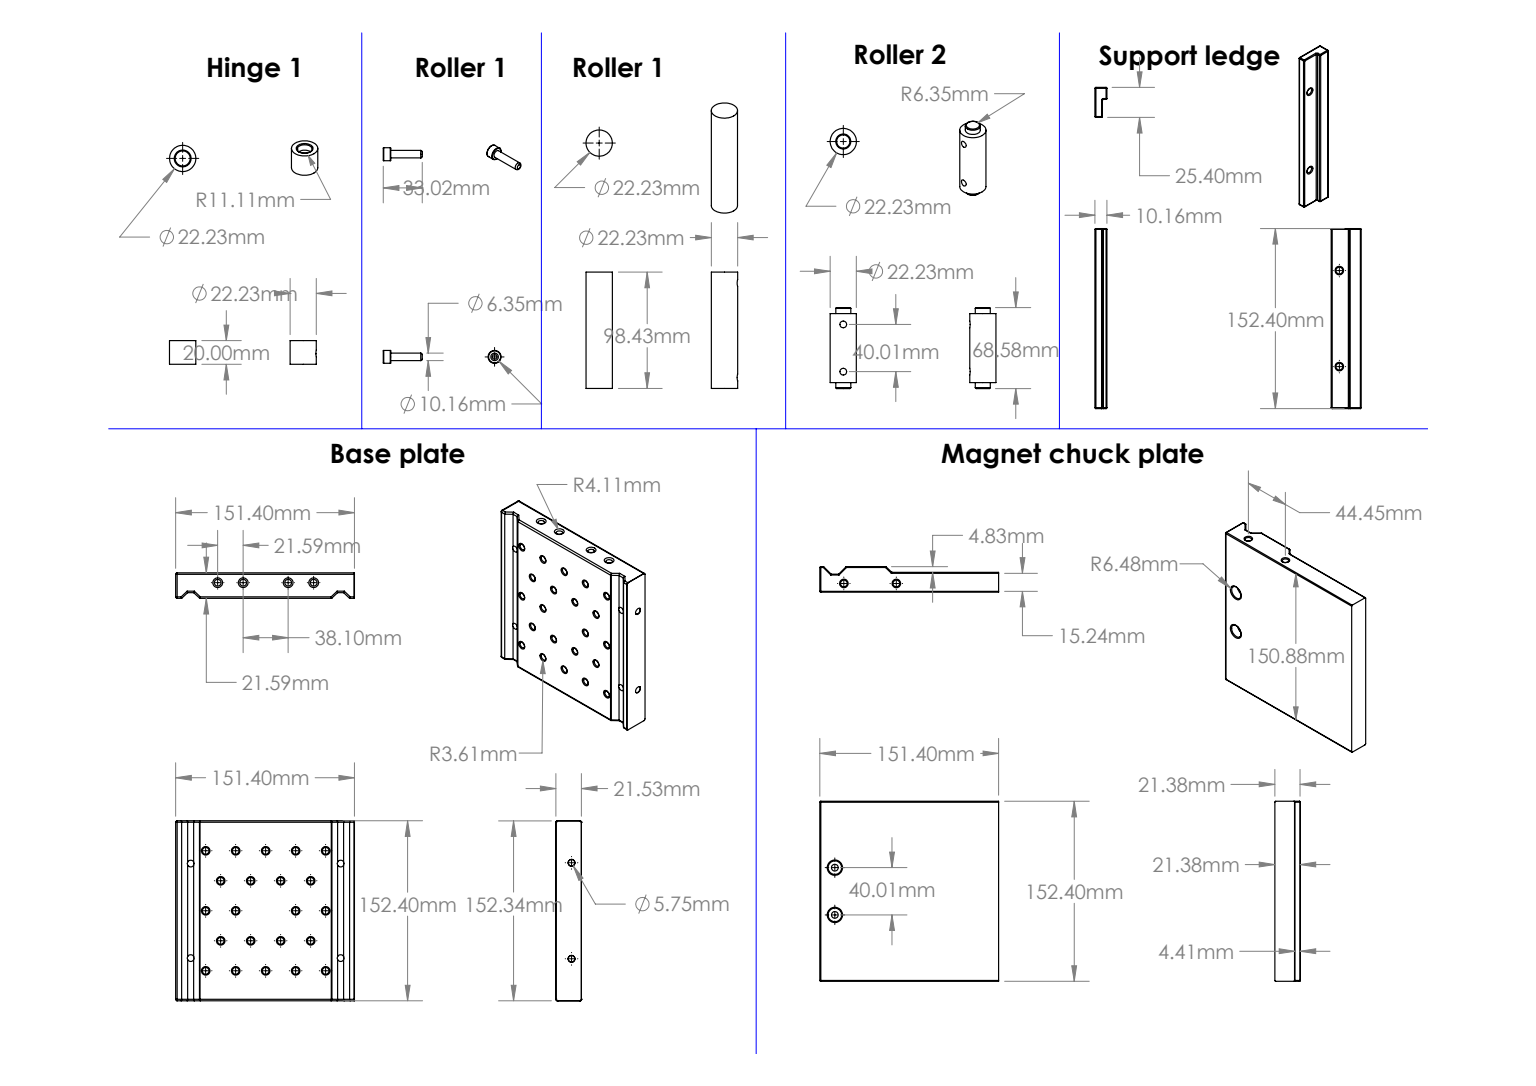
ISO-10303-21;
HEADER;
FILE_DESCRIPTION (('STEP AP214'),
    '1' );
FILE_NAME ('Base Plate.step',
    '2026-10-26T17:37:43',
    ( '' ),
    ( '' ),
    'SwSTEP 2.0',
    'SolidWorks 2024',
    '' );
FILE_SCHEMA (( 'AUTOMOTIVE_DESIGN' ));
ENDSEC;

DATA;
#2=CARTESIAN_POINT ( 'NONE',  ( 137.0307011298872908, -3580.478779010893959, 2249.731360258177119 ) ) ;
#4=DIRECTION ( 'NONE',  ( 0.000000000000000000, 1.000000000000000000, 0.000000000000000000 ) ) ;
#7=CARTESIAN_POINT ( 'NONE',  ( 116.8400000000000034, -3543.299999999999727, 2247.392000000000280 ) ) ;
#9=DIRECTION ( 'NONE',  ( -1.000000000000000000, 0.000000000000000000, 0.000000000000000000 ) ) ;
#13=EDGE_LOOP ( 'NONE', ( #4801, #14751 ) ) ;
#15=CARTESIAN_POINT ( 'NONE',  ( 15.55036781974841453, -3695.600514565457615, 2254.996746371283280 ) ) ;
#18=CARTESIAN_POINT ( 'NONE',  ( 50.79999999999999716, -3619.500000000000000, 2259.837999999999738 ) ) ;
#20=DIRECTION ( 'NONE',  ( 9.756599977372053330E-14, 0.000000000000000000, -1.000000000000000000 ) ) ;
#22=FACE_OUTER_BOUND ( 'NONE', #22533, .T. ) ;
#29=CARTESIAN_POINT ( 'NONE',  ( 17.55427699106284933, -3576.478798487876247, 2245.835327951717773 ) ) ;
#31=DIRECTION ( 'NONE',  ( 0.000000000000000000, 0.000000000000000000, -1.000000000000000000 ) ) ;
#34=CARTESIAN_POINT ( 'NONE',  ( 9.652920519510999497, -3695.699999999999818, 2254.503999999999905 ) ) ;
#37=CARTESIAN_POINT ( 'NONE',  ( 137.2900278743959745, -3657.993505329751770, 2249.258937114173477 ) ) ;
#41=ORIENTED_EDGE ( 'NONE', *, *, #19227, .F. ) ;
#45=EDGE_LOOP ( 'NONE', ( #8949, #290, #14111, #10584 ) ) ;
#48=ORIENTED_EDGE ( 'NONE', *, *, #14973, .T. ) ;
#49=ORIENTED_EDGE ( 'NONE', *, *, #4852, .F. ) ;
#50=DIRECTION ( 'NONE',  ( 0.000000000000000000, 0.000000000000000000, -1.000000000000000000 ) ) ;
#51=ADVANCED_FACE ( 'NONE', ( #16778 ), #19588, .T. ) ;
#54=CYLINDRICAL_SURFACE ( 'NONE', #7821, 5.714999999999998082 ) ;
#58=CARTESIAN_POINT ( 'NONE',  ( 12.69999999999999929, -3579.494999999999891, 2246.630000000000109 ) ) ;
#59=CYLINDRICAL_SURFACE ( 'NONE', #10460, 2.844800000000091700 ) ;
#61=CARTESIAN_POINT ( 'NONE',  ( 116.8400000000000034, -3694.430000000000291, 2247.392000000000280 ) ) ;
#63=EDGE_CURVE ( 'NONE', #17851, #18027, #1534, .T. ) ;
#65=ORIENTED_EDGE ( 'NONE', *, *, #14589, .T. ) ;
#67=DIRECTION ( 'NONE',  ( 0.000000000000000000, 0.000000000000000000, 1.000000000000000000 ) ) ;
#68=ORIENTED_EDGE ( 'NONE', *, *, #2483, .T. ) ;
#71=CARTESIAN_POINT ( 'NONE',  ( 25.39999999999999858, -3660.140000000000327, 2247.392000000000280 ) ) ;
#72=CARTESIAN_POINT ( 'NONE',  ( 41.70680000000000121, -3644.899999999999636, 2239.009999999999764 ) ) ;
#73=CARTESIAN_POINT ( 'NONE',  ( 151.1299999999999955, -3694.430000000000291, 2259.329999999999927 ) ) ;
#75=CARTESIAN_POINT ( 'NONE',  ( 18.25500259602790720, -3658.162202898845862, 2245.347138497373180 ) ) ;
#76=EDGE_CURVE ( 'NONE', #7743, #14640, #1242, .T. ) ;
#78=FACE_OUTER_BOUND ( 'NONE', #21782, .T. ) ;
#79=EDGE_CURVE ( 'NONE', #18611, #6224, #7995, .T. ) ;
#84=CARTESIAN_POINT ( 'NONE',  ( 137.1117535491106594, -3694.976217804482530, 2255.653245237783267 ) ) ;
#85=ORIENTED_EDGE ( 'NONE', *, *, #8808, .F. ) ;
#87=DIRECTION ( 'NONE',  ( 0.000000000000000000, 0.000000000000000000, 1.000000000000000000 ) ) ;
#89=AXIS2_PLACEMENT_3D ( 'NONE', #13714, #3272, #12061 ) ;
#91=CARTESIAN_POINT ( 'NONE',  ( 135.0886139726000010, -3662.880847139000252, 2246.630000000000109 ) ) ;
#93=CYLINDRICAL_SURFACE ( 'NONE', #6462, 1.269999999999882334 ) ;
#96=ADVANCED_FACE ( 'NONE', ( #13964 ), #8465, .F. ) ;
#97=AXIS2_PLACEMENT_3D ( 'NONE', #21852, #23131, #10839 ) ;
#98=DIRECTION ( 'NONE',  ( 0.000000000000000000, 0.000000000000000000, 1.000000000000000000 ) ) ;
#99=AXIS2_PLACEMENT_3D ( 'NONE', #19425, #3130, #10398 ) ;
#101=DIRECTION ( 'NONE',  ( 0.000000000000000000, 0.000000000000000000, 1.000000000000000000 ) ) ;
#102=ORIENTED_EDGE ( 'NONE', *, *, #7130, .F. ) ;
#103=TOROIDAL_SURFACE ( 'NONE', #6096, 3.606799999999999784, 0.7620000000000000107 ) ;
#104=DIRECTION ( 'NONE',  ( 0.000000000000000000, 0.000000000000000000, -1.000000000000000000 ) ) ;
#105=CIRCLE ( 'NONE', #22163, 3.606799999999993567 ) ;
#108=CARTESIAN_POINT ( 'NONE',  ( 85.29320000000001301, -3644.899999999999636, 2239.009999999999764 ) ) ;
#109=B_SPLINE_CURVE_WITH_KNOTS ( 'NONE', 3,
 ( #11658, #15542, #8166, #2887, #6654, #22328, #18938, #6532, #2998, #1356, #1238, #17171, #20933, #8046, #13430, #10031, #13667, #10147, #3112, #15428, #1118, #2762, #4874, #20571, #12026, #4523, #19295, #6764, #17285, #8277, #9904, #15664, #4637, #20688, #8398, #18816, #19176, #8521, #22561, #22681, #20817, #22437, #17053, #1005, #15312, #6412, #19058, #17399, #13905, #11785, #22788, #21052 ),
 .UNSPECIFIED., .F., .F.,
 ( 4, 2, 1, 1, 1, 1, 2, 2, 2, 1, 2, 2, 2, 2, 1, 1, 1, 2, 2, 2, 2, 1, 1, 1, 2, 2, 2, 1, 1, 1, 2, 2, 4 ),
 ( 0.000000000000000000, 0.003906250000015105105, 0.007812500000030210209, 0.01562500000044777723, 0.03125000000089964147, 0.06250000000180337689, 0.1250000000036391445, 0.2500000000076161855, 0.2656250000084233176, 0.2812500000092305052, 0.3125000000108511533, 0.3750000000142236778, 0.5000000000208256745, 0.5019531250208819628, 0.5039062500209382511, 0.5078125000210353956, 0.5156250000208461026, 0.5312500000204676276, 0.5625000000200504058, 0.6250000000192512672, 0.6289062500191696659, 0.6328125000190880645, 0.6406250000187544424, 0.6562500000179013471, 0.6875000000160184088, 0.7500000000124475985, 0.7539062500122738486, 0.7578125000121000987, 0.7656250000119128041, 0.7812500000113792309, 0.8125000000098967501, 0.8750000000066556760, 1.000000000000000000 ),
 .UNSPECIFIED. ) ;
#110=EDGE_LOOP ( 'NONE', ( #14632, #871, #3105, #5719 ) ) ;
#111=CARTESIAN_POINT ( 'NONE',  ( 142.6612001523742208, -3695.684722679518018, 2254.718298691088421 ) ) ;
#112=DIRECTION ( 'NONE',  ( 1.000000000000000000, 0.000000000000000000, 0.000000000000000000 ) ) ;
#115=EDGE_CURVE ( 'NONE', #4940, #21098, #2726, .T. ) ;
#117=CARTESIAN_POINT ( 'NONE',  ( 137.1107034105660034, -3580.676250239197998, 2249.584241783140442 ) ) ;
#119=DIRECTION ( 'NONE',  ( 1.224646799147353207E-16, 1.000000000000000000, -0.000000000000000000 ) ) ;
#121=CIRCLE ( 'NONE', #1224, 2.844800000000091700 ) ;
#122=CARTESIAN_POINT ( 'NONE',  ( 6.996782844457664297, -3579.071241691879095, 2244.547217133379945 ) ) ;
#123=DIRECTION ( 'NONE',  ( 0.000000000000000000, 0.000000000000000000, -1.000000000000000000 ) ) ;
#124=ADVANCED_FACE ( 'NONE', ( #19237 ), #13848, .F. ) ;
#125=DIRECTION ( 'NONE',  ( -1.000000000000000000, 0.000000000000000000, 0.000000000000000000 ) ) ;
#127=EDGE_LOOP ( 'NONE', ( #9464, #14168, #22567, #17753 ) ) ;
#128=CARTESIAN_POINT ( 'NONE',  ( 141.9735787716368804, -3577.784544496731542, 2250.025932887172985 ) ) ;
#130=AXIS2_PLACEMENT_3D ( 'NONE', #3984, #794, #16512 ) ;
#131=CARTESIAN_POINT ( 'NONE',  ( 134.0223127011804252, -3578.842640279839998, 2244.547249493357413 ) ) ;
#132=EDGE_CURVE ( 'NONE', #6511, #15378, #5378, .T. ) ;
#133=EDGE_CURVE ( 'NONE', #17829, #16978, #3861, .T. ) ;
#135=ORIENTED_EDGE ( 'NONE', *, *, #969, .F. ) ;
#138=CIRCLE ( 'NONE', #3486, 0.7619999999999987894 ) ;
#139=CLOSED_SHELL ( 'NONE', ( #18289, #7008, #8518, #22594, #20989, #23105, #16145, #3413, #11794, #2224, #2827, #1410, #16543, #19416, #8130, #13424, #4558, #15262, #22286, #8396, #19575, #9289, #13963, #21111, #15810, #7255, #18256, #22413, #19334, #8366, #20531, #3559, #5670, #14740, #18979, #14141, #9599, #14263, #10124, #6147, #22178, #12747, #12264, #9427, #21177, #17826, #16370, #12412, #15426, #5281, #20386, #14683, #16750, #2410, #10013, #13395, #16311, #7711, #4641, #19449, #4494, #20415, #21019, #22225, #51, #6503, #13150, #17175, #14109, #16374, #18246, #13592, #4477, #20450, #11729, #3837, #17376, #8709, #18820, #14659, #4694, #4420, #5580, #11076, #2706, #6139, #12300, #1249, #21474, #5517, #12872, #14173, #13268, #987, #12573, #13097, #1664, #18403, #22007, #19391, #3382, #1211, #5961, #11237, #5886, #6240, #19563, #17791, #16108, #12536, #16780, #15034, #22219, #16319, #12028, #639, #4268, #6646, #19581, #19988, #13241, #6285, #15946, #4264, #21207, #2054, #22523, #7877, #11589, #22115, #16270, #96, #13253, #16398, #4808, #22277, #13435, #22678, #11382, #13308, #16585, #7024, #2755, #9237, #5116, #15881, #12312, #7534, #10663, #16517, #6439, #10126, #19876, #16966, #14807, #20512, #21309, #6853, #805, #16656, #19994, #11360, #8292, #8247, #511, #18141, #8217, #8284, #20809, #15008, #18035, #14102, #15702, #2487, #7663, #10088, #14883, #1165, #15813, #6527, #13028, #17258, #14527, #3507, #2757, #21880, #10849, #8534, #17415, #20660, #18719, #3789, #13015, #1704, #22836, #5727, #9542, #18530, #20029, #22101, #3836, #20839, #5077, #16041, #11870, #14827, #21582, #6419, #5871, #17134, #3910, #5590, #14945, #16186, #7678, #21286, #12539, #7356, #7419, #6403, #1767, #10423, #16431, #5343, #124, #22382, #20876, #14160, #2061, #4392, #471, #2508, #9317, #22720, #967, #22838, #18612, #8833, #5095, #23099, #12516, #18309, #6530, #2705, #20259, #5803, #15689, #10375, #23161, #22806, #22870, #9927, #11310, #13967, #17673, #19716, #15974, #22128, #14003, #5885, #23135, #5290, #5119, #11638, #6284, #7996, #769, #4193, #15853, #18569, #4096, #19675, #3268, #9017, #3364, #233, #11495, #6410, #14763, #6092, #8252, #7227, #12142, #21432 ) ) ;
#140=VERTEX_POINT ( 'NONE', #15613 ) ;
#141=DIRECTION ( 'NONE',  ( 1.000000000000000000, 0.000000000000000000, 0.000000000000000000 ) ) ;
#143=ORIENTED_EDGE ( 'NONE', *, *, #16586, .F. ) ;
#147=CARTESIAN_POINT ( 'NONE',  ( 86.05520000000001346, -3644.899999999999636, 2261.869999999999891 ) ) ;
#148=CARTESIAN_POINT ( 'NONE',  ( 35.56000000000000227, -3694.430000000000291, 2243.277199999999993 ) ) ;
#149=CIRCLE ( 'NONE', #19230, 4.114799999999974034 ) ;
#152=CARTESIAN_POINT ( 'NONE',  ( 9.823095770001307514, -3695.626565546511301, 2254.929879519301721 ) ) ;
#153=EDGE_LOOP ( 'NONE', ( #3229, #589, #13779, #13464, #20523, #7090, #21786, #14841 ) ) ;
#154=CARTESIAN_POINT ( 'NONE',  ( 18.26408956042804377, -3580.799603742805175, 2245.310931594975045 ) ) ;
#155=CARTESIAN_POINT ( 'NONE',  ( 137.5777489049088160, -3657.610548859369828, 2248.693836209597066 ) ) ;
#156=ORIENTED_EDGE ( 'NONE', *, *, #8169, .T. ) ;
#157=ORIENTED_EDGE ( 'NONE', *, *, #22934, .F. ) ;
#158=CARTESIAN_POINT ( 'NONE',  ( 137.6199768978073905, -3661.447896576730727, 2249.919485654132586 ) ) ;
#159=VERTEX_POINT ( 'NONE', #14082 ) ;
#160=ORIENTED_EDGE ( 'NONE', *, *, #9548, .T. ) ;
#161=ORIENTED_EDGE ( 'NONE', *, *, #12576, .T. ) ;
#162=AXIS2_PLACEMENT_3D ( 'NONE', #11218, #12637, #3839 ) ;
#163=DIRECTION ( 'NONE',  ( 0.000000000000000000, 0.000000000000000000, -1.000000000000000000 ) ) ;
#164=CIRCLE ( 'NONE', #18872, 1.270000000000000018 ) ;
#165=ORIENTED_EDGE ( 'NONE', *, *, #16586, .T. ) ;
#166=ORIENTED_EDGE ( 'NONE', *, *, #22581, .T. ) ;
#167=DIRECTION ( 'NONE',  ( 1.000000000000000000, -0.000000000000000000, -0.000000000000000000 ) ) ;
#169=CARTESIAN_POINT ( 'NONE',  ( 9.956800000000452400, -3660.383257047480583, 2255.967039999999997 ) ) ;
#177=CARTESIAN_POINT ( 'NONE',  ( 142.5448000000000093, -3579.495004790000166, 2250.165035197999714 ) ) ;
#178=EDGE_LOOP ( 'NONE', ( #370, #14088 ) ) ;
#179=AXIS2_PLACEMENT_3D ( 'NONE', #16153, #101, #7252 ) ;
#181=CARTESIAN_POINT ( 'NONE',  ( 151.1299999999999955, -3544.570000000000164, 2240.279999999999745 ) ) ;
#183=CARTESIAN_POINT ( 'NONE',  ( 7.963520823585933606, -3662.703639150101026, 2246.156481404430906 ) ) ;
#188=CARTESIAN_POINT ( 'NONE',  ( 139.6999999999999886, -3579.494999999999891, 2239.009999999999764 ) ) ;
#193=CARTESIAN_POINT ( 'NONE',  ( 147.4191677002133929, -3695.185487567203381, 2260.351709085013226 ) ) ;
#195=CARTESIAN_POINT ( 'NONE',  ( 25.39999999999999858, -3670.300000000000182, 2239.771999999999935 ) ) ;
#196=AXIS2_PLACEMENT_3D ( 'NONE', #17467, #5408, #21233 ) ;
#198=AXIS2_PLACEMENT_3D ( 'NONE', #803, #13353, #20498 ) ;
#201=DIRECTION ( 'NONE',  ( 0.000000000000000000, 0.000000000000000000, -1.000000000000000000 ) ) ;
#202=DIRECTION ( 'NONE',  ( 0.000000000000000000, 0.000000000000000000, -1.000000000000000000 ) ) ;
#203=CARTESIAN_POINT ( 'NONE',  ( 7.471656874357363698, -3577.187248168970200, 2245.090911189840881 ) ) ;
#212=CARTESIAN_POINT ( 'NONE',  ( 127.0000000000000000, -3578.860000000000127, 2247.392000000000280 ) ) ;
#213=CARTESIAN_POINT ( 'NONE',  ( 88.90000000000000568, -3644.899999999999636, 2239.771999999999935 ) ) ;
#215=AXIS2_PLACEMENT_3D ( 'NONE', #7884, #11390, #22164 ) ;
#216=B_SPLINE_CURVE_WITH_KNOTS ( 'NONE', 3,
 ( #18119, #3820, #429, #5713, #3941, #21530, #9448, #2077, #14847, #4055, #12848, #14381, #19885, #21978, #4168, #5485, #12624, #3704, #7461, #5944, #19777, #18463, #10857, #18005, #1953, #14614, #21868, #12732, #9109, #13074, #20121 ),
 .UNSPECIFIED., .F., .F.,
 ( 4, 2, 2, 2, 2, 2, 1, 2, 2, 2, 2, 1, 1, 2, 2, 2, 4 ),
 ( 0.000000000000000000, 0.1250000000032115977, 0.1875000000050884574, 0.2500000000069653172, 0.3750000000111080589, 0.4375000000130825906, 0.4687500000140698009, 0.4843750000143322576, 0.5000000000145947698, 0.6250000000177098336, 0.6875000000192672545, 0.7187500000200460759, 0.7343750000203067563, 0.7421875000204309902, 0.7500000000205552242, 0.8750000000102775566, 1.000000000000000000 ),
 .UNSPECIFIED. ) ;
#218=LINE ( 'NONE', #7366, #10755 ) ;
#219=CIRCLE ( 'NONE', #19664, 3.606799999999993567 ) ;
#222=AXIS2_PLACEMENT_3D ( 'NONE', #21550, #10764, #3608 ) ;
#223=ORIENTED_EDGE ( 'NONE', *, *, #11710, .T. ) ;
#226=CARTESIAN_POINT ( 'NONE',  ( 139.6999999999999886, -3659.504999999999654, 2239.771999999999935 ) ) ;
#228=ORIENTED_EDGE ( 'NONE', *, *, #17836, .F. ) ;
#233=ADVANCED_FACE ( 'NONE', ( #17343 ), #7401, .T. ) ;
#234=AXIS2_PLACEMENT_3D ( 'NONE', #17409, #21062, #21410 ) ;
#235=VECTOR ( 'NONE', #20474, 1000.000000000000000 ) ;
#238=AXIS2_PLACEMENT_3D ( 'NONE', #213, #10759, #14515 ) ;
#239=CARTESIAN_POINT ( 'NONE',  ( 137.7798478441602583, -3581.594086837189934, 2248.178223016279844 ) ) ;
#240=ORIENTED_EDGE ( 'NONE', *, *, #6122, .T. ) ;
#242=AXIS2_PLACEMENT_3D ( 'NONE', #13170, #5587, #11300 ) ;
#246=FACE_OUTER_BOUND ( 'NONE', #8836, .T. ) ;
#249=LINE ( 'NONE', #19809, #13213 ) ;
#251=CARTESIAN_POINT ( 'NONE',  ( 138.0292475174377671, -3577.192411888781862, 2249.696850050126159 ) ) ;
#260=AXIS2_PLACEMENT_3D ( 'NONE', #525, #18221, #2401 ) ;
#262=DIRECTION ( 'NONE',  ( 0.000000000000000000, 0.000000000000000000, -1.000000000000000000 ) ) ;
#264=ORIENTED_EDGE ( 'NONE', *, *, #17863, .T. ) ;
#267=DIRECTION ( 'NONE',  ( 1.073225997510925892E-13, 0.000000000000000000, 1.000000000000000000 ) ) ;
#268=DIRECTION ( 'NONE',  ( -1.000000000000000000, 0.000000000000000000, 0.000000000000000000 ) ) ;
#272=CIRCLE ( 'NONE', #10732, 6.477000000000000313 ) ;
#273=CARTESIAN_POINT ( 'NONE',  ( 20.59150445774999838, -3694.472271328999796, 2260.600000000000364 ) ) ;
#274=CARTESIAN_POINT ( 'NONE',  ( 9.851025909890511301, -3695.599092773431494, 2255.000090470981831 ) ) ;
#275=ORIENTED_EDGE ( 'NONE', *, *, #7383, .T. ) ;
#278=CARTESIAN_POINT ( 'NONE',  ( 117.9067999999989951, -3644.899999999999636, 2260.600000000000364 ) ) ;
#279=VERTEX_POINT ( 'NONE', #21692 ) ;
#280=CARTESIAN_POINT ( 'NONE',  ( 138.4989950604438604, -3662.085293714453655, 2249.468401061301847 ) ) ;
#281=EDGE_CURVE ( 'NONE', #13787, #22341, #17933, .T. ) ;
#283=EDGE_LOOP ( 'NONE', ( #11779, #4580, #14894, #1068 ) ) ;
#284=CIRCLE ( 'NONE', #2157, 0.7619999999999294005 ) ;
#285=CARTESIAN_POINT ( 'NONE',  ( 9.916854418464000176, -3578.905956564000007, 2250.236428761999832 ) ) ;
#286=ORIENTED_EDGE ( 'NONE', *, *, #14831, .T. ) ;
#287=VERTEX_POINT ( 'NONE', #2127 ) ;
#288=CARTESIAN_POINT ( 'NONE',  ( 151.4000000000000057, -3694.430000000000291, 2259.329999999999927 ) ) ;
#290=ORIENTED_EDGE ( 'NONE', *, *, #8429, .F. ) ;
#291=AXIS2_PLACEMENT_3D ( 'NONE', #23158, #21545, #3370 ) ;
#293=CIRCLE ( 'NONE', #11497, 0.7619999999999987894 ) ;
#299=EDGE_LOOP ( 'NONE', ( #10110, #17418, #6158, #21329 ) ) ;
#300=DIRECTION ( 'NONE',  ( -1.000000000000000000, 0.000000000000000000, 0.000000000000000000 ) ) ;
#304=CARTESIAN_POINT ( 'NONE',  ( 1.270000000000000018, -3578.860000000000127, 2244.547199999999975 ) ) ;
#305=ORIENTED_EDGE ( 'NONE', *, *, #9304, .F. ) ;
#306=CARTESIAN_POINT ( 'NONE',  ( 95.25000000000000000, -3544.570000000000164, 2247.392000000000280 ) ) ;
#307=CARTESIAN_POINT ( 'NONE',  ( 63.50000000000000000, -3594.099999999999909, 2259.837999999999738 ) ) ;
#310=CARTESIAN_POINT ( 'NONE',  ( 18.11219821918659179, -3657.669286988329986, 2245.981668378579798 ) ) ;
#311=ORIENTED_EDGE ( 'NONE', *, *, #22098, .F. ) ;
#312=DIRECTION ( 'NONE',  ( -1.000000000000000000, 0.000000000000000000, 0.000000000000000000 ) ) ;
#313=DIRECTION ( 'NONE',  ( -1.000000000000000000, 0.000000000000000000, 0.000000000000000000 ) ) ;
#316=CARTESIAN_POINT ( 'NONE',  ( 142.5448000000000093, -3579.495004790000166, 2250.165035197999714 ) ) ;
#317=FACE_OUTER_BOUND ( 'NONE', #5413, .T. ) ;
#318=CARTESIAN_POINT ( 'NONE',  ( 137.0608322996959316, -3695.185487567919154, 2255.525709084477512 ) ) ;
#319=CARTESIAN_POINT ( 'NONE',  ( 7.834922896206100162, -3576.496315022116505, 2245.808993730167458 ) ) ;
#325=CARTESIAN_POINT ( 'NONE',  ( 29.00679999999900005, -3619.500000000000000, 2239.771999999999935 ) ) ;
#327=ORIENTED_EDGE ( 'NONE', *, *, #11023, .F. ) ;
#331=CARTESIAN_POINT ( 'NONE',  ( 47.19319999999999737, -3670.300000000000182, 2260.600000000000364 ) ) ;
#333=EDGE_CURVE ( 'NONE', #1510, #18918, #3750, .T. ) ;
#336=FACE_OUTER_BOUND ( 'NONE', #5464, .T. ) ;
#337=EDGE_CURVE ( 'NONE', #11629, #10297, #6048, .T. ) ;
#338=ORIENTED_EDGE ( 'NONE', *, *, #15407, .T. ) ;
#340=DIRECTION ( 'NONE',  ( 1.000000000000000000, 0.000000000000000000, 0.000000000000000000 ) ) ;
#342=ORIENTED_EDGE ( 'NONE', *, *, #3117, .T. ) ;
#344=CARTESIAN_POINT ( 'NONE',  ( 137.7661303793067873, -3581.581515421061795, 2248.220692510852587 ) ) ;
#347=AXIS2_PLACEMENT_3D ( 'NONE', #19188, #3123, #5242 ) ;
#352=CARTESIAN_POINT ( 'NONE',  ( 1.270000000000000018, -3694.430000000000291, 2240.279999999999745 ) ) ;
#353=CARTESIAN_POINT ( 'NONE',  ( 133.9849999999989905, -3579.494999999999891, 2239.771999999999935 ) ) ;
#356=CARTESIAN_POINT ( 'NONE',  ( 138.7293422311318807, -3576.819596326436567, 2249.374802684401402 ) ) ;
#357=ORIENTED_EDGE ( 'NONE', *, *, #14314, .T. ) ;
#359=AXIS2_PLACEMENT_3D ( 'NONE', #17047, #1111, #22432 ) ;
#360=DIRECTION ( 'NONE',  ( 0.000000000000000000, 0.000000000000000000, 1.000000000000000000 ) ) ;
#362=CARTESIAN_POINT ( 'NONE',  ( 6.985000000000000320, -3659.504999999999654, 2239.771999999999935 ) ) ;
#369=EDGE_CURVE ( 'NONE', #923, #11706, #14203, .T. ) ;
#370=ORIENTED_EDGE ( 'NONE', *, *, #1712, .T. ) ;
#371=EDGE_CURVE ( 'NONE', #830, #1510, #5294, .T. ) ;
#372=CYLINDRICAL_SURFACE ( 'NONE', #653, 1.269999999999882334 ) ;
#373=DIRECTION ( 'NONE',  ( 0.000000000000000000, 0.000000000000000000, 1.000000000000000000 ) ) ;
#375=ORIENTED_EDGE ( 'NONE', *, *, #3846, .F. ) ;
#379=DIRECTION ( 'NONE',  ( 0.8068916933307923589, -0.5906994119124941989, 0.000000000000000000 ) ) ;
#380=ORIENTED_EDGE ( 'NONE', *, *, #14174, .F. ) ;
#382=CARTESIAN_POINT ( 'NONE',  ( 18.14049516396890027, -3581.245129373504369, 2245.841260512669123 ) ) ;
#386=CARTESIAN_POINT ( 'NONE',  ( 138.2628149773561290, -3661.960543573507948, 2249.578175895470395 ) ) ;
#388=ORIENTED_EDGE ( 'NONE', *, *, #4639, .T. ) ;
#394=DIRECTION ( 'NONE',  ( -1.000000000000000000, 0.000000000000000000, 0.000000000000000000 ) ) ;
#397=ORIENTED_EDGE ( 'NONE', *, *, #13639, .F. ) ;
#399=CARTESIAN_POINT ( 'NONE',  ( 7.254607931487381478, -3581.231065619790570, 2245.814675045431159 ) ) ;
#402=EDGE_CURVE ( 'NONE', #14892, #830, #14431, .T. ) ;
#405=ORIENTED_EDGE ( 'NONE', *, *, #418, .F. ) ;
#409=EDGE_CURVE ( 'NONE', #2915, #8062, #11888, .T. ) ;
#413=DIRECTION ( 'NONE',  ( 1.000000000000000000, 0.000000000000000000, 0.000000000000000000 ) ) ;
#418=EDGE_CURVE ( 'NONE', #21665, #9059, #5768, .T. ) ;
#419=DIRECTION ( 'NONE',  ( 0.000000000000000000, 1.000000000000000000, 0.000000000000000000 ) ) ;
#421=AXIS2_PLACEMENT_3D ( 'NONE', #17372, #1683, #23118 ) ;
#423=CARTESIAN_POINT ( 'NONE',  ( 147.6218463403696433, -3543.408637598981386, 2259.843959195220123 ) ) ;
#425=CARTESIAN_POINT ( 'NONE',  ( 147.5078116312014060, -3695.420022018752661, 2260.129812754224076 ) ) ;
#427=DIRECTION ( 'NONE',  ( 1.000000000000000000, 0.000000000000000000, 0.000000000000000000 ) ) ;
#428=DIRECTION ( 'NONE',  ( 1.000000000000000000, 0.000000000000000000, 0.000000000000000000 ) ) ;
#429=CARTESIAN_POINT ( 'NONE',  ( 142.2430419228115284, -3544.409801990574579, 2255.766443268943476 ) ) ;
#434=EDGE_CURVE ( 'NONE', #17725, #22994, #2393, .T. ) ;
#436=DIRECTION ( 'NONE',  ( 0.000000000000000000, 0.000000000000000000, -1.000000000000000000 ) ) ;
#437=CIRCLE ( 'NONE', #19133, 0.7619999999999987894 ) ;
#444=VERTEX_POINT ( 'NONE', #17555 ) ;
#445=CARTESIAN_POINT ( 'NONE',  ( 50.79999999999999716, -3568.700000000000273, 2259.837999999999738 ) ) ;
#446=DIRECTION ( 'NONE',  ( 0.000000000000000000, 0.000000000000000000, -1.000000000000000000 ) ) ;
#448=FACE_OUTER_BOUND ( 'NONE', #9717, .T. ) ;
#449=CIRCLE ( 'NONE', #16159, 1.269999999999882334 ) ;
#453=DIRECTION ( 'NONE',  ( -1.000000000000000000, -0.000000000000000000, -0.000000000000000000 ) ) ;
#454=DIRECTION ( 'NONE',  ( -1.224646799147353207E-16, 1.000000000000000000, 0.000000000000000000 ) ) ;
#456=CARTESIAN_POINT ( 'NONE',  ( 137.9046276598544978, -3581.701726360760404, 2247.546642836707633 ) ) ;
#457=ORIENTED_EDGE ( 'NONE', *, *, #13685, .F. ) ;
#458=CARTESIAN_POINT ( 'NONE',  ( 145.3734778515583344, -3580.182493284074553, 2244.873281192526065 ) ) ;
#465=CARTESIAN_POINT ( 'NONE',  ( 25.39999999999999858, -3660.140000000000327, 2244.547199999999975 ) ) ;
#466=CARTESIAN_POINT ( 'NONE',  ( 145.4149999980000132, -3659.715610845466017, 2244.570779584676529 ) ) ;
#468=EDGE_CURVE ( 'NONE', #10446, #7103, #4622, .T. ) ;
#469=CARTESIAN_POINT ( 'NONE',  ( 141.6187116912652186, -3577.394048819144245, 2249.830271027571598 ) ) ;
#471=ADVANCED_FACE ( 'NONE', ( #6567 ), #18840, .T. ) ;
#473=VERTEX_POINT ( 'NONE', #13826 ) ;
#474=DIRECTION ( 'NONE',  ( 0.000000000000000000, -1.000000000000000000, 0.000000000000000000 ) ) ;
#475=CARTESIAN_POINT ( 'NONE',  ( 15.54870723730916104, -3543.401189131915999, 2255.000759462869155 ) ) ;
#477=ORIENTED_EDGE ( 'NONE', *, *, #20451, .T. ) ;
#478=CARTESIAN_POINT ( 'NONE',  ( 127.0000000000000000, -3568.700000000000273, 2239.771999999999935 ) ) ;
#485=CARTESIAN_POINT ( 'NONE',  ( 13.71111753102643327, -3576.835601115875306, 2249.390789936909187 ) ) ;
#487=DIRECTION ( 'NONE',  ( 0.000000000000000000, 0.000000000000000000, -1.000000000000000000 ) ) ;
#488=ORIENTED_EDGE ( 'NONE', *, *, #7154, .F. ) ;
#489=DIRECTION ( 'NONE',  ( 0.000000000000000000, -1.000000000000000000, 0.000000000000000000 ) ) ;
#494=ORIENTED_EDGE ( 'NONE', *, *, #11128, .T. ) ;
#495=CARTESIAN_POINT ( 'NONE',  ( 18.12359179772333206, -3581.296656515060022, 2245.923799407296883 ) ) ;
#499=ORIENTED_EDGE ( 'NONE', *, *, #7556, .F. ) ;
#500=CIRCLE ( 'NONE', #22927, 3.606800000000000228 ) ;
#501=EDGE_CURVE ( 'NONE', #14295, #9663, #683, .T. ) ;
#502=CARTESIAN_POINT ( 'NONE',  ( 141.3123101578824787, -3661.849600747001659, 2249.666225506271530 ) ) ;
#505=ORIENTED_EDGE ( 'NONE', *, *, #11069, .T. ) ;
#507=DIRECTION ( 'NONE',  ( -1.000000000000000000, 0.000000000000000000, 0.000000000000000000 ) ) ;
#511=ADVANCED_FACE ( 'NONE', ( #11306 ), #18000, .F. ) ;
#513=ORIENTED_EDGE ( 'NONE', *, *, #7023, .T. ) ;
#514=CARTESIAN_POINT ( 'NONE',  ( 6.985153502415998972, -3659.391482155004724, 2244.644944835688875 ) ) ;
#515=CARTESIAN_POINT ( 'NONE',  ( 7.283171614331794608, -3581.316932381231254, 2245.957881525527227 ) ) ;
#516=EDGE_CURVE ( 'NONE', #8087, #21408, #6409, .T. ) ;
#521=CARTESIAN_POINT ( 'NONE',  ( 76.20000000000000284, -3670.300000000000182, 2259.837999999999738 ) ) ;
#525=CARTESIAN_POINT ( 'NONE',  ( 15.24000000000000021, -3695.699999999999818, 2255.774000000000342 ) ) ;
#526=EDGE_CURVE ( 'NONE', #16634, #17242, #1905, .T. ) ;
#533=ORIENTED_EDGE ( 'NONE', *, *, #21014, .F. ) ;
#537=DIRECTION ( 'NONE',  ( 1.000000000000000000, -0.000000000000000000, 1.224646799147353207E-16 ) ) ;
#539=CYLINDRICAL_SURFACE ( 'NONE', #15070, 2.844799999998995244 ) ;
#541=CIRCLE ( 'NONE', #4305, 2.844800000000091700 ) ;
#542=LINE ( 'NONE', #21648, #18834 ) ;
#543=ORIENTED_EDGE ( 'NONE', *, *, #6594, .F. ) ;
#547=CARTESIAN_POINT ( 'NONE',  ( 145.4149999978999972, -3659.505243078000149, 2244.618209833000492 ) ) ;
#548=EDGE_CURVE ( 'NONE', #6059, #12867, #16146, .T. ) ;
#549=CARTESIAN_POINT ( 'NONE',  ( 10.01629450381963693, -3580.440293654210564, 2249.758428457885657 ) ) ;
#550=CARTESIAN_POINT ( 'NONE',  ( 38.10000000000000142, -3594.099999999999909, 2261.869999999999891 ) ) ;
#551=EDGE_LOOP ( 'NONE', ( #13315, #19240, #6873, #12519 ) ) ;
#552=FACE_OUTER_BOUND ( 'NONE', #9739, .T. ) ;
#553=VERTEX_POINT ( 'NONE', #5596 ) ;
#557=DIRECTION ( 'NONE',  ( -1.000000000000000000, 0.000000000000000000, 0.000000000000000000 ) ) ;
#558=VECTOR ( 'NONE', #12526, 1000.000000000000000 ) ;
#559=EDGE_CURVE ( 'NONE', #12638, #14575, #4895, .T. ) ;
#560=DIRECTION ( 'NONE',  ( 0.000000000000000000, 0.000000000000000000, -1.000000000000000000 ) ) ;
#561=TOROIDAL_SURFACE ( 'NONE', #15532, 3.606799999999999784, 0.7620000000000000107 ) ;
#566=CARTESIAN_POINT ( 'NONE',  ( 133.2229999999989900, -3579.494999999999891, 2239.771999999999935 ) ) ;
#569=CARTESIAN_POINT ( 'NONE',  ( 127.0000000000000000, -3619.500000000000000, 2239.771999999999935 ) ) ;
#572=VERTEX_POINT ( 'NONE', #14610 ) ;
#573=B_SPLINE_CURVE_WITH_KNOTS ( 'NONE', 3,
 ( #8571, #6467, #2818, #12194, #6355, #17224, #3164, #8457, #6587, #4928, #17460, #6814, #19231, #11959, #13955, #4695, #17114, #22735, #1290, #13608, #21105, #10199, #10317, #13841, #5050, #20988, #17338, #15366, #12074, #1412, #19346, #16993, #13728, #943, #11845, #10078, #8335, #8216, #4579, #15480, #22380 ),
 .UNSPECIFIED., .F., .F.,
 ( 4, 2, 2, 1, 1, 2, 2, 2, 2, 1, 1, 1, 2, 2, 2, 2, 2, 2, 2, 1, 1, 2, 2, 4 ),
 ( 0.000000000000000000, 0.1249999999964153119, 0.1874999999948339380, 0.2187499999938449513, 0.2343749999936358408, 0.2421874999938173900, 0.2499999999939989115, 0.3749999999956662444, 0.4374999999964459541, 0.4687499999966819875, 0.4843749999968000042, 0.4921874999968590125, 0.4960937499968964826, 0.4999999999969340081, 0.5624999999948754326, 0.5937499999937037032, 0.6249999999925319738, 0.6874999999899414904, 0.7187499999887656532, 0.7343749999881804547, 0.7421874999878907975, 0.7460937499877459134, 0.7499999999876010293, 1.000000000000000000 ),
 .UNSPECIFIED. ) ;
#579=AXIS2_PLACEMENT_3D ( 'NONE', #12558, #10797, #10682 ) ;
#581=LINE ( 'NONE', #9484, #20792 ) ;
#584=CARTESIAN_POINT ( 'NONE',  ( 142.2297613316639797, -3578.193174660338627, 2250.157761700695119 ) ) ;
#586=B_SPLINE_CURVE_WITH_KNOTS ( 'NONE', 3,
 ( #14737, #5248, #12392, #19538, #3477, #12506 ),
 .UNSPECIFIED., .F., .F.,
 ( 4, 1, 1, 4 ),
 ( 0.000000000000000000, 0.3333333333333000081, 0.6666666666667000474, 1.000000000000000000 ),
 .UNSPECIFIED. ) ;
#589=ORIENTED_EDGE ( 'NONE', *, *, #12880, .F. ) ;
#591=CARTESIAN_POINT ( 'NONE',  ( 142.5448000000000093, -3659.504999999999654, 2256.063560000000052 ) ) ;
#593=AXIS2_PLACEMENT_3D ( 'NONE', #5374, #17902, #21270 ) ;
#594=ORIENTED_EDGE ( 'NONE', *, *, #22385, .F. ) ;
#596=ORIENTED_EDGE ( 'NONE', *, *, #22546, .F. ) ;
#597=CARTESIAN_POINT ( 'NONE',  ( 57.14999999999999858, -3543.300000000000182, 2251.506800000000112 ) ) ;
#600=CARTESIAN_POINT ( 'NONE',  ( 14.56785476897627341, -3577.348371727691301, 2249.802387783117410 ) ) ;
#601=CARTESIAN_POINT ( 'NONE',  ( 141.5643557054172845, -3581.643940524072150, 2246.800655991665735 ) ) ;
#605=CARTESIAN_POINT ( 'NONE',  ( 20.43202061276000236, -3694.678775005999796, 2260.577432963000319 ) ) ;
#608=AXIS2_PLACEMENT_3D ( 'NONE', #1214, #8376, #22656 ) ;
#609=AXIS2_PLACEMENT_3D ( 'NONE', #5564, #4025, #11052 ) ;
#610=DIRECTION ( 'NONE',  ( 0.000000000000000000, 0.000000000000000000, -1.000000000000000000 ) ) ;
#613=CARTESIAN_POINT ( 'NONE',  ( 141.7318470609411065, -3661.497086795617179, 2249.892725811761011 ) ) ;
#614=ORIENTED_EDGE ( 'NONE', *, *, #19767, .F. ) ;
#615=AXIS2_PLACEMENT_3D ( 'NONE', #11553, #18701, #2651 ) ;
#617=ORIENTED_EDGE ( 'NONE', *, *, #76, .T. ) ;
#620=EDGE_CURVE ( 'NONE', #3298, #2966, #20610, .T. ) ;
#621=ORIENTED_EDGE ( 'NONE', *, *, #8439, .F. ) ;
#622=ORIENTED_EDGE ( 'NONE', *, *, #5424, .F. ) ;
#623=CARTESIAN_POINT ( 'NONE',  ( 147.3199999999999932, -3544.570000000000164, 2260.600000000000364 ) ) ;
#624=DIRECTION ( 'NONE',  ( 0.000000000000000000, 0.000000000000000000, -1.000000000000000000 ) ) ;
#630=CARTESIAN_POINT ( 'NONE',  ( 145.3796772601000100, -3660.139769217999856, 2244.548186305999934 ) ) ;
#632=DIRECTION ( 'NONE',  ( 1.000000000000000000, 0.000000000000000000, 0.000000000000000000 ) ) ;
#634=EDGE_CURVE ( 'NONE', #10444, #22942, #12024, .T. ) ;
#637=DIRECTION ( 'NONE',  ( -1.000000000000000000, 0.000000000000000000, 0.000000000000000000 ) ) ;
#638=DIRECTION ( 'NONE',  ( -1.000000000000000000, 0.000000000000000000, 0.000000000000000000 ) ) ;
#639=ADVANCED_FACE ( 'NONE', ( #13525 ), #4161, .T. ) ;
#640=ORIENTED_EDGE ( 'NONE', *, *, #11917, .T. ) ;
#642=DIRECTION ( 'NONE',  ( 0.000000000000000000, 0.000000000000000000, -1.000000000000000000 ) ) ;
#645=ORIENTED_EDGE ( 'NONE', *, *, #5737, .F. ) ;
#648=CARTESIAN_POINT ( 'NONE',  ( 18.35682388039437640, -3658.691851779573881, 2244.943199301839741 ) ) ;
#650=VERTEX_POINT ( 'NONE', #22192 ) ;
#653=AXIS2_PLACEMENT_3D ( 'NONE', #7513, #14669, #21470 ) ;
#655=CARTESIAN_POINT ( 'NONE',  ( 111.4552000000009997, -3644.899999999999636, 2261.869999999999891 ) ) ;
#656=DIRECTION ( 'NONE',  ( -1.000000000000000000, 0.000000000000000000, 0.000000000000000000 ) ) ;
#658=CARTESIAN_POINT ( 'NONE',  ( 20.37014473194848918, -3695.033231289878131, 2260.474410595720656 ) ) ;
#659=ORIENTED_EDGE ( 'NONE', *, *, #20177, .T. ) ;
#663=ORIENTED_EDGE ( 'NONE', *, *, #15516, .F. ) ;
#664=CARTESIAN_POINT ( 'NONE',  ( 145.1453925538234273, -3657.768934968029953, 2245.814674103072775 ) ) ;
#666=CARTESIAN_POINT ( 'NONE',  ( 9.913021306595382498, -3580.067331691507206, 2249.967926883056407 ) ) ;
#667=LINE ( 'NONE', #14627, #2267 ) ;
#669=CARTESIAN_POINT ( 'NONE',  ( 134.0204252830999962, -3660.140268639000169, 2244.547525601999951 ) ) ;
#670=CARTESIAN_POINT ( 'NONE',  ( 9.652920519510999497, -3695.699999999999818, 2254.503999999999905 ) ) ;
#673=DIRECTION ( 'NONE',  ( -0.000000000000000000, 1.000000000000000000, 0.000000000000000000 ) ) ;
#674=CARTESIAN_POINT ( 'NONE',  ( 13.60653736635324762, -3662.201562304035178, 2249.352418353455505 ) ) ;
#675=CIRCLE ( 'NONE', #12272, 3.606800000000000228 ) ;
#679=DIRECTION ( 'NONE',  ( 1.000000000000000000, 0.000000000000000000, 0.000000000000000000 ) ) ;
#680=ORIENTED_EDGE ( 'NONE', *, *, #11726, .T. ) ;
#681=DIRECTION ( 'NONE',  ( -1.000000000000000000, 0.000000000000000000, 0.000000000000000000 ) ) ;
#682=CYLINDRICAL_SURFACE ( 'NONE', #10572, 2.844800000000001550 ) ;
#683=B_SPLINE_CURVE_WITH_KNOTS ( 'NONE', 3,
 ( #20967, #4674, #15583, #4912, #10968, #9219, #12727, #19881, #9444, #11089, #193, #4051, #12620, #11197, #19772, #16699, #4164, #425, #21750, #7344, #13070, #14726, #20221, #21863, #12959, #2187, #7564, #16360, #5708, #20001, #1949 ),
 .UNSPECIFIED., .F., .F.,
 ( 4, 2, 2, 2, 2, 2, 1, 2, 2, 2, 2, 1, 1, 2, 2, 2, 4 ),
 ( 0.000000000000000000, 0.1249999999996052324, 0.1874999999994706734, 0.2499999999993361421, 0.3749999999984279242, 0.4374999999981442622, 0.4687499999978084197, 0.4843749999976455500, 0.4999999999974826803, 0.6249999999991210364, 0.6874999999997667421, 0.7187499999998425704, 0.7343750000001272316, 0.7421875000001436629, 0.7500000000001599831, 0.8750000000000800471, 1.000000000000000000 ),
 .UNSPECIFIED. ) ;
#684=EDGE_LOOP ( 'NONE', ( #19969, #16210, #13476, #14572, #12675, #15722, #4180, #12665 ) ) ;
#686=CARTESIAN_POINT ( 'NONE',  ( 20.82707948048999924, -3695.699999999999818, 2259.329999999999927 ) ) ;
#687=ORIENTED_EDGE ( 'NONE', *, *, #12448, .F. ) ;
#688=CARTESIAN_POINT ( 'NONE',  ( 145.3843004971977564, -3580.087277415173048, 2244.825193658660282 ) ) ;
#690=EDGE_CURVE ( 'NONE', #10874, #18714, #15406, .T. ) ;
#692=DIRECTION ( 'NONE',  ( -1.000000000000000000, 0.000000000000000000, 0.000000000000000000 ) ) ;
#693=EDGE_CURVE ( 'NONE', #7794, #10683, #1154, .T. ) ;
#694=CARTESIAN_POINT ( 'NONE',  ( 17.56334821106831967, -3662.506481300412815, 2245.813177206671298 ) ) ;
#696=LINE ( 'NONE', #18724, #15131 ) ;
#699=LINE ( 'NONE', #4216, #9234 ) ;
#700=ORIENTED_EDGE ( 'NONE', *, *, #6839, .T. ) ;
#704=CARTESIAN_POINT ( 'NONE',  ( 15.70174596896855057, -3543.300000000022010, 2254.617539517661498 ) ) ;
#708=AXIS2_PLACEMENT_3D ( 'NONE', #9587, #453, #16733 ) ;
#711=CARTESIAN_POINT ( 'NONE',  ( 11.57570654715081737, -3576.881424651616726, 2249.436186243917291 ) ) ;
#713=CARTESIAN_POINT ( 'NONE',  ( 141.7107714205274931, -3581.507805183896835, 2248.433351161166229 ) ) ;
#719=CARTESIAN_POINT ( 'NONE',  ( 136.8551930557000276, -3659.332964842520141, 2250.125630000906767 ) ) ;
#720=ORIENTED_EDGE ( 'NONE', *, *, #5225, .T. ) ;
#722=ORIENTED_EDGE ( 'NONE', *, *, #10015, .F. ) ;
#723=FACE_OUTER_BOUND ( 'NONE', #15167, .T. ) ;
#724=VERTEX_POINT ( 'NONE', #18794 ) ;
#726=CARTESIAN_POINT ( 'NONE',  ( 133.2229999999999848, -3659.504999999999654, 2239.771999999999935 ) ) ;
#727=ORIENTED_EDGE ( 'NONE', *, *, #369, .T. ) ;
#728=CARTESIAN_POINT ( 'NONE',  ( 7.003448455909224712, -3659.044352728992635, 2244.765892648666977 ) ) ;
#731=CIRCLE ( 'NONE', #1095, 4.114799999999974034 ) ;
#734=CARTESIAN_POINT ( 'NONE',  ( 12.69999999999999929, -3579.494999999999891, 2246.630000000000109 ) ) ;
#736=CARTESIAN_POINT ( 'NONE',  ( 142.4974789541179234, -3658.986641539371703, 2249.992541019687451 ) ) ;
#738=ORIENTED_EDGE ( 'NONE', *, *, #22032, .F. ) ;
#744=ORIENTED_EDGE ( 'NONE', *, *, #18244, .F. ) ;
#745=DIRECTION ( 'NONE',  ( 0.000000000000000000, 0.000000000000000000, 1.000000000000000000 ) ) ;
#747=CARTESIAN_POINT ( 'NONE',  ( 18.33711823532055973, -3658.564445501008322, 2245.022483595459107 ) ) ;
#749=VERTEX_POINT ( 'NONE', #20786 ) ;
#752=CARTESIAN_POINT ( 'NONE',  ( 117.1447999999989946, -3644.899999999999636, 2239.771999999999935 ) ) ;
#754=CARTESIAN_POINT ( 'NONE',  ( 127.0000000000000000, -3660.140000000000327, 2244.547199999999975 ) ) ;
#755=DIRECTION ( 'NONE',  ( 0.000000000000000000, 0.000000000000000000, 1.000000000000000000 ) ) ;
#756=CARTESIAN_POINT ( 'NONE',  ( 101.5999999999999943, -3670.300000000000182, 2239.771999999999935 ) ) ;
#757=CARTESIAN_POINT ( 'NONE',  ( 20.82707948048999924, -3695.699999999999818, 2259.329999999999927 ) ) ;
#760=AXIS2_PLACEMENT_3D ( 'NONE', #9119, #16259, #5610 ) ;
#764=CARTESIAN_POINT ( 'NONE',  ( 1.270000000000000018, -3660.140000000000327, 2250.236800000000130 ) ) ;
#765=AXIS2_PLACEMENT_3D ( 'NONE', #17214, #2932, #21303 ) ;
#769=ADVANCED_FACE ( 'NONE', ( #9773 ), #6049, .T. ) ;
#771=CARTESIAN_POINT ( 'NONE',  ( 134.9056831650161712, -3576.384005279409848, 2245.990590281915502 ) ) ;
#773=DIRECTION ( 'NONE',  ( 0.000000000000000000, 0.000000000000000000, -1.000000000000000000 ) ) ;
#775=CARTESIAN_POINT ( 'NONE',  ( 14.60105122252583598, -3661.621915575120056, 2249.820482541457750 ) ) ;
#780=DIRECTION ( 'NONE',  ( 0.000000000000000000, 0.000000000000000000, 1.000000000000000000 ) ) ;
#781=FACE_BOUND ( 'NONE', #2465, .T. ) ;
#783=DIRECTION ( 'NONE',  ( 0.000000000000000000, 0.000000000000000000, -1.000000000000000000 ) ) ;
#786=VECTOR ( 'NONE', #17705, 1000.000000000000000 ) ;
#791=CARTESIAN_POINT ( 'NONE',  ( 145.4031900104867532, -3579.124489882064609, 2244.559018039585226 ) ) ;
#792=CARTESIAN_POINT ( 'NONE',  ( 18.21505860824958489, -3661.003409629256566, 2244.681372502921931 ) ) ;
#794=DIRECTION ( 'NONE',  ( 0.000000000000000000, 0.000000000000000000, 1.000000000000000000 ) ) ;
#795=CARTESIAN_POINT ( 'NONE',  ( 137.3409534416252882, -3577.904103566719641, 2250.071838006614144 ) ) ;
#797=CIRCLE ( 'NONE', #11314, 2.844799999999994444 ) ;
#799=EDGE_CURVE ( 'NONE', #13105, #20246, #7087, .T. ) ;
#801=CARTESIAN_POINT ( 'NONE',  ( 35.25520000000000209, -3644.899999999999636, 2261.869999999999891 ) ) ;
#802=ORIENTED_EDGE ( 'NONE', *, *, #4244, .F. ) ;
#803=CARTESIAN_POINT ( 'NONE',  ( 41.70680000000000121, -3594.099999999999909, 2259.837999999999738 ) ) ;
#804=CARTESIAN_POINT ( 'NONE',  ( 15.56736770577728812, -3543.382189095376816, 2254.953892137616549 ) ) ;
#805=ADVANCED_FACE ( 'NONE', ( #15870 ), #10238, .T. ) ;
#809=ORIENTED_EDGE ( 'NONE', *, *, #15098, .F. ) ;
#813=CARTESIAN_POINT ( 'NONE',  ( 10.16000000000000014, -3544.570000000000164, 2255.774000000000342 ) ) ;
#814=CARTESIAN_POINT ( 'NONE',  ( 13.24259552251218253, -3576.687580108851762, 2249.232770475404322 ) ) ;
#816=CARTESIAN_POINT ( 'NONE',  ( 141.4866483936817474, -3581.708819005992609, 2247.454754559452795 ) ) ;
#818=EDGE_CURVE ( 'NONE', #8027, #749, #22847, .T. ) ;
#820=AXIS2_PLACEMENT_3D ( 'NONE', #17542, #22924, #10165 ) ;
#823=AXIS2_PLACEMENT_3D ( 'NONE', #8783, #454, #20150 ) ;
#825=VERTEX_POINT ( 'NONE', #10356 ) ;
#826=CARTESIAN_POINT ( 'NONE',  ( 20.66695186275289586, -3543.364998063555959, 2259.731097527611382 ) ) ;
#827=EDGE_CURVE ( 'NONE', #13681, #7121, #20278, .T. ) ;
#829=EDGE_CURVE ( 'NONE', #8062, #928, #9069, .T. ) ;
#830=VERTEX_POINT ( 'NONE', #15641 ) ;
#831=AXIS2_PLACEMENT_3D ( 'NONE', #4811, #14196, #10553 ) ;
#832=DIRECTION ( 'NONE',  ( 0.000000000000000000, 0.000000000000000000, 1.000000000000000000 ) ) ;
#837=EDGE_CURVE ( 'NONE', #159, #10812, #12396, .T. ) ;
#838=DIRECTION ( 'NONE',  ( -1.000000000000000000, 0.000000000000000000, 0.000000000000000000 ) ) ;
#843=CARTESIAN_POINT ( 'NONE',  ( 7.127793039152298782, -3658.235454836550616, 2245.278666177176092 ) ) ;
#844=CARTESIAN_POINT ( 'NONE',  ( 50.79999999999999716, -3619.500000000000000, 2260.600000000000364 ) ) ;
#846=AXIS2_PLACEMENT_3D ( 'NONE', #22613, #20873, #1170 ) ;
#848=DIRECTION ( 'NONE',  ( 0.000000000000000000, 1.000000000000000000, 0.000000000000000000 ) ) ;
#850=TOROIDAL_SURFACE ( 'NONE', #13965, 3.606799999999999784, 0.7620000000000000107 ) ;
#854=EDGE_LOOP ( 'NONE', ( #8023, #7975, #7190, #21142 ) ) ;
#855=CARTESIAN_POINT ( 'NONE',  ( 137.1478751023463474, -3544.290797603923693, 2255.743570596557220 ) ) ;
#856=ORIENTED_EDGE ( 'NONE', *, *, #6594, .T. ) ;
#857=AXIS2_PLACEMENT_3D ( 'NONE', #11933, #20845, #22816 ) ;
#859=DIRECTION ( 'NONE',  ( -1.000000000000000000, 0.000000000000000000, 0.000000000000000000 ) ) ;
#862=DIRECTION ( 'NONE',  ( 0.7249994335945011414, 0.000000000000000000, -0.6887494619146010688 ) ) ;
#869=DIRECTION ( 'NONE',  ( 0.000000000000000000, 0.000000000000000000, -1.000000000000000000 ) ) ;
#871=ORIENTED_EDGE ( 'NONE', *, *, #559, .F. ) ;
#873=CARTESIAN_POINT ( 'NONE',  ( 145.0770480762069781, -3657.568064249584950, 2246.174318179428155 ) ) ;
#874=AXIS2_PLACEMENT_3D ( 'NONE', #21453, #5403, #3402 ) ;
#875=CYLINDRICAL_SURFACE ( 'NONE', #3817, 2.844800000000091700 ) ;
#876=CARTESIAN_POINT ( 'NONE',  ( 9.855099624826999971, -3659.717132568602665, 2250.213600093685272 ) ) ;
#879=CARTESIAN_POINT ( 'NONE',  ( 151.1299999999999955, -3544.570000000000164, 2259.329999999999927 ) ) ;
#881=ORIENTED_EDGE ( 'NONE', *, *, #371, .F. ) ;
#882=CARTESIAN_POINT ( 'NONE',  ( 85.29320000000001301, -3594.099999999999909, 2260.600000000000364 ) ) ;
#883=CARTESIAN_POINT ( 'NONE',  ( 14.89040167505680401, -3661.320454366029480, 2249.980433560093843 ) ) ;
#895=EDGE_LOOP ( 'NONE', ( #856, #7799, #9527, #3867 ) ) ;
#896=EDGE_CURVE ( 'NONE', #1677, #13988, #5664, .T. ) ;
#898=EDGE_CURVE ( 'NONE', #22077, #9946, #21383, .T. ) ;
#899=ORIENTED_EDGE ( 'NONE', *, *, #15246, .T. ) ;
#900=CARTESIAN_POINT ( 'NONE',  ( 145.1993249291396069, -3581.050454772452667, 2245.576347930728843 ) ) ;
#905=CIRCLE ( 'NONE', #11387, 1.269999999999993356 ) ;
#908=DIRECTION ( 'NONE',  ( 0.000000000000000000, 0.000000000000000000, -1.000000000000000000 ) ) ;
#912=B_SPLINE_CURVE_WITH_KNOTS ( 'NONE', 3,
 ( #15628, #20771, #22755, #13981 ),
 .UNSPECIFIED., .F., .F.,
 ( 4, 4 ),
 ( 0.000000000000000000, 1.000000000000000000 ),
 .UNSPECIFIED. ) ;
#916=DIRECTION ( 'NONE',  ( 0.000000000000000000, 0.000000000000000000, -1.000000000000000000 ) ) ;
#919=CARTESIAN_POINT ( 'NONE',  ( 18.41519309055000164, -3659.504912144000173, 2244.618989493999834 ) ) ;
#922=ORIENTED_EDGE ( 'NONE', *, *, #20905, .F. ) ;
#923=VERTEX_POINT ( 'NONE', #16335 ) ;
#924=DIRECTION ( 'NONE',  ( 0.000000000000000000, 0.000000000000000000, -1.000000000000000000 ) ) ;
#926=B_SPLINE_CURVE_WITH_KNOTS ( 'NONE', 3,
 ( #9817, #18617, #7734, #4437, #20157, #11573, #11239, #17080, #4543, #792, #22125, #14886, #13456, #2457, #11348, #6204, #18387, #16964, #6323, #13223, #20489, #20371, #20269, #2337, #22014, #16621, #13113, #14991, #8073, #18843, #5872, #2562, #2785, #4208, #9931, #18720, #9601, #18498, #8187, #21907, #9709, #16848, #15220, #694, #7843, #15108, #22231 ),
 .UNSPECIFIED., .F., .F.,
 ( 4, 2, 2, 1, 1, 2, 2, 2, 2, 1, 1, 1, 1, 2, 2, 2, 2, 2, 1, 2, 2, 2, 2, 1, 1, 2, 2, 4 ),
 ( 0.000000000000000000, 0.1250000000146304913, 0.1875000000219457230, 0.2187500000256033528, 0.2343750000274318346, 0.2421875000283457424, 0.2500000000292596503, 0.3750000000440060766, 0.4375000000513063481, 0.4687500000549565393, 0.4843750000567812464, 0.4921875000575812731, 0.4960937500578705417, 0.4980468750579331028, 0.5000000000579956083, 0.5625000000547328849, 0.5937500000531019673, 0.6093750000522863974, 0.6171875000518064480, 0.6210937500514964738, 0.6250000000511864995, 0.6875000000439721592, 0.7187500000402435862, 0.7343750000383787446, 0.7421875000375531828, 0.7460937500370307118, 0.7500000000365082409, 1.000000000000000000 ),
 .UNSPECIFIED. ) ;
#928=VERTEX_POINT ( 'NONE', #12699 ) ;
#929=AXIS2_PLACEMENT_3D ( 'NONE', #20726, #4336, #20384 ) ;
#931=CARTESIAN_POINT ( 'NONE',  ( 10.99145740650285319, -3577.220312686051329, 2249.716781721822827 ) ) ;
#934=CARTESIAN_POINT ( 'NONE',  ( 142.0761082949672982, -3581.059198188035680, 2249.196594758551328 ) ) ;
#935=ORIENTED_EDGE ( 'NONE', *, *, #12718, .F. ) ;
#939=EDGE_CURVE ( 'NONE', #17172, #16346, #1530, .T. ) ;
#940=DIRECTION ( 'NONE',  ( -1.000000000000000000, 0.000000000000000000, 0.000000000000000000 ) ) ;
#943=CARTESIAN_POINT ( 'NONE',  ( 134.2700811556670999, -3657.722455772349349, 2245.892455863900068 ) ) ;
#945=CIRCLE ( 'NONE', #2107, 3.606800000000000228 ) ;
#947=AXIS2_PLACEMENT_3D ( 'NONE', #9154, #360, #5985 ) ;
#949=EDGE_LOOP ( 'NONE', ( #16333, #1362, #2481, #15726 ) ) ;
#950=ORIENTED_EDGE ( 'NONE', *, *, #15391, .T. ) ;
#951=CARTESIAN_POINT ( 'NONE',  ( 130.6067999999989979, -3670.300000000000182, 2239.009999999999764 ) ) ;
#955=DIRECTION ( 'NONE',  ( 0.000000000000000000, -1.000000000000000000, 0.000000000000000000 ) ) ;
#956=EDGE_CURVE ( 'NONE', #5163, #4127, #15793, .T. ) ;
#958=CARTESIAN_POINT ( 'NONE',  ( 7.179249868354160569, -3658.027629572277874, 2245.486160608427326 ) ) ;
#961=AXIS2_PLACEMENT_3D ( 'NONE', #7228, #7453, #21861 ) ;
#964=DIRECTION ( 'NONE',  ( 0.000000000000000000, -1.000000000000000000, 0.000000000000000000 ) ) ;
#965=DIRECTION ( 'NONE',  ( 0.000000000000000000, 0.000000000000000000, 1.000000000000000000 ) ) ;
#967=ADVANCED_FACE ( 'NONE', ( #21497 ), #19739, .F. ) ;
#968=DIRECTION ( 'NONE',  ( 1.000000000000000000, 0.000000000000000000, 0.000000000000000000 ) ) ;
#969=EDGE_CURVE ( 'NONE', #12882, #7229, #14290, .T. ) ;
#971=CIRCLE ( 'NONE', #15574, 0.7619999999999987894 ) ;
#974=FACE_OUTER_BOUND ( 'NONE', #6628, .T. ) ;
#980=CARTESIAN_POINT ( 'NONE',  ( 117.9067999999989951, -3594.099999999999909, 2260.600000000000364 ) ) ;
#982=VERTEX_POINT ( 'NONE', #17970 ) ;
#985=TOROIDAL_SURFACE ( 'NONE', #6999, 3.606799999999999784, 0.7620000000000000107 ) ;
#987=ADVANCED_FACE ( 'NONE', ( #16214 ), #20275, .T. ) ;
#988=EDGE_CURVE ( 'NONE', #6309, #16212, #2601, .T. ) ;
#989=VECTOR ( 'NONE', #22563, 1000.000000000000000 ) ;
#992=FACE_OUTER_BOUND ( 'NONE', #6317, .T. ) ;
#998=DIRECTION ( 'NONE',  ( 0.000000000000000000, 0.000000000000000000, -1.000000000000000000 ) ) ;
#999=CIRCLE ( 'NONE', #8125, 1.269999999999882334 ) ;
#1002=DIRECTION ( 'NONE',  ( 0.000000000000000000, 0.000000000000000000, 1.000000000000000000 ) ) ;
#1005=CARTESIAN_POINT ( 'NONE',  ( 144.5506343064713803, -3662.527019523321087, 2245.844349661943852 ) ) ;
#1006=ORIENTED_EDGE ( 'NONE', *, *, #12155, .F. ) ;
#1007=CARTESIAN_POINT ( 'NONE',  ( 105.2067999999999870, -3568.700000000000273, 2259.837999999999738 ) ) ;
#1008=CARTESIAN_POINT ( 'NONE',  ( 14.17818779929573658, -3661.936027002551782, 2249.598227899164613 ) ) ;
#1009=ORIENTED_EDGE ( 'NONE', *, *, #7436, .T. ) ;
#1010=FACE_OUTER_BOUND ( 'NONE', #19730, .T. ) ;
#1012=CIRCLE ( 'NONE', #20868, 1.269999999999882334 ) ;
#1015=DIRECTION ( 'NONE',  ( 1.000000000000000000, 0.000000000000000000, 0.000000000000000000 ) ) ;
#1018=AXIS2_PLACEMENT_3D ( 'NONE', #17663, #8653, #21200 ) ;
#1023=DIRECTION ( 'NONE',  ( 0.000000000000000000, 0.000000000000000000, 1.000000000000000000 ) ) ;
#1029=EDGE_CURVE ( 'NONE', #4102, #3301, #16883, .T. ) ;
#1033=AXIS2_PLACEMENT_3D ( 'NONE', #1523, #3286, #15281 ) ;
#1034=EDGE_CURVE ( 'NONE', #2027, #9562, #13521, .T. ) ;
#1039=DIRECTION ( 'NONE',  ( 0.000000000000000000, 0.000000000000000000, -1.000000000000000000 ) ) ;
#1042=ORIENTED_EDGE ( 'NONE', *, *, #5637, .T. ) ;
#1043=EDGE_LOOP ( 'NONE', ( #18572, #7602, #16545, #8314 ) ) ;
#1049=DIRECTION ( 'NONE',  ( -1.000000000000000000, 0.000000000000000000, 0.000000000000000000 ) ) ;
#1053=CARTESIAN_POINT ( 'NONE',  ( 141.5833498427044788, -3581.627187199552282, 2248.052646821879534 ) ) ;
#1059=DIRECTION ( 'NONE',  ( 1.000000000000000000, 0.000000000000000000, 0.000000000000000000 ) ) ;
#1061=CARTESIAN_POINT ( 'NONE',  ( 142.4730284656999970, -3660.140000970000074, 2250.236800000000130 ) ) ;
#1063=AXIS2_PLACEMENT_3D ( 'NONE', #9805, #5967, #12995 ) ;
#1068=ORIENTED_EDGE ( 'NONE', *, *, #5816, .T. ) ;
#1072=ORIENTED_EDGE ( 'NONE', *, *, #10277, .F. ) ;
#1073=DIRECTION ( 'NONE',  ( -1.000000000000000000, 0.000000000000000000, 0.000000000000000000 ) ) ;
#1074=CARTESIAN_POINT ( 'NONE',  ( 137.1599999999999966, -3544.570000000000164, 2255.774000000000342 ) ) ;
#1075=DIRECTION ( 'NONE',  ( 0.000000000000000000, 0.000000000000000000, -1.000000000000000000 ) ) ;
#1079=DIRECTION ( 'NONE',  ( 0.000000000000000000, 0.000000000000000000, 1.000000000000000000 ) ) ;
#1082=CARTESIAN_POINT ( 'NONE',  ( 141.9222097098283371, -3657.728223441102273, 2248.902296121618747 ) ) ;
#1083=CARTESIAN_POINT ( 'NONE',  ( 35.56000000000000227, -3694.430000000000291, 2251.506800000000112 ) ) ;
#1089=CIRCLE ( 'NONE', #359, 4.114799999999974034 ) ;
#1095=AXIS2_PLACEMENT_3D ( 'NONE', #16221, #14126, #21385 ) ;
#1097=EDGE_CURVE ( 'NONE', #7706, #11149, #20418, .T. ) ;
#1100=DIRECTION ( 'NONE',  ( 0.000000000000000000, 0.000000000000000000, 1.000000000000000000 ) ) ;
#1105=ORIENTED_EDGE ( 'NONE', *, *, #10084, .F. ) ;
#1107=DIRECTION ( 'NONE',  ( 0.000000000000000000, -2.331176954594000018E-14, 1.000000000000000000 ) ) ;
#1108=EDGE_CURVE ( 'NONE', #10881, #6183, #10904, .T. ) ;
#1110=CARTESIAN_POINT ( 'NONE',  ( 10.19827476683941825, -3580.849530610950296, 2249.426096155833875 ) ) ;
#1111=DIRECTION ( 'NONE',  ( 0.000000000000000000, -1.000000000000000000, 0.000000000000000000 ) ) ;
#1117=FACE_OUTER_BOUND ( 'NONE', #19737, .T. ) ;
#1118=CARTESIAN_POINT ( 'NONE',  ( 144.9133339346259390, -3661.846445636756471, 2245.115832528513693 ) ) ;
#1119=DIRECTION ( 'NONE',  ( 0.000000000000000000, -1.000000000000000000, 0.000000000000000000 ) ) ;
#1124=DIRECTION ( 'NONE',  ( 0.000000000000000000, 0.000000000000000000, -1.000000000000000000 ) ) ;
#1125=VECTOR ( 'NONE', #6435, 1000.000000000000000 ) ;
#1127=CARTESIAN_POINT ( 'NONE',  ( 136.8551930557000276, -3659.505009668000184, 2250.165028799000083 ) ) ;
#1128=CARTESIAN_POINT ( 'NONE',  ( 134.3871257470999865, -3581.600847139000052, 2246.630000000000109 ) ) ;
#1139=DIRECTION ( 'NONE',  ( -1.000000000000000000, 0.000000000000000000, 0.000000000000000000 ) ) ;
#1143=CYLINDRICAL_SURFACE ( 'NONE', #10596, 5.714999999999999858 ) ;
#1145=CARTESIAN_POINT ( 'NONE',  ( 137.2727299238133583, -3578.011210012966785, 2250.107278179072637 ) ) ;
#1148=CARTESIAN_POINT ( 'NONE',  ( 1.270000000000000018, -3543.299999999999727, 2240.279999999999745 ) ) ;
#1152=CARTESIAN_POINT ( 'NONE',  ( 10.13128874078853414, -3658.282160798511995, 2249.547058791628388 ) ) ;
#1153=ORIENTED_EDGE ( 'NONE', *, *, #16561, .T. ) ;
#1154=CIRCLE ( 'NONE', #16503, 3.606799999999993567 ) ;
#1156=CARTESIAN_POINT ( 'NONE',  ( 134.1795861059526374, -3580.969250050632581, 2245.481136081417844 ) ) ;
#1157=EDGE_LOOP ( 'NONE', ( #19411, #15979, #3547, #7427 ) ) ;
#1159=CARTESIAN_POINT ( 'NONE',  ( 29.00679999999900005, -3568.700000000000273, 2259.837999999999738 ) ) ;
#1161=CARTESIAN_POINT ( 'NONE',  ( 141.6023748289098592, -3581.610180818415756, 2248.119666950691226 ) ) ;
#1165=ADVANCED_FACE ( 'NONE', ( #11612 ), #6827, .T. ) ;
#1167=CARTESIAN_POINT ( 'NONE',  ( 14.58530482363100766, -3581.625685692691150, 2248.064425038887748 ) ) ;
#1169=EDGE_CURVE ( 'NONE', #18991, #7862, #5466, .T. ) ;
#1170=DIRECTION ( 'NONE',  ( 0.000000000000000000, 1.000000000000000000, 0.000000000000000000 ) ) ;
#1172=ORIENTED_EDGE ( 'NONE', *, *, #5841, .F. ) ;
#1173=CARTESIAN_POINT ( 'NONE',  ( 0.000000000000000000, -3694.430000000000291, 2254.503999999999905 ) ) ;
#1176=DIRECTION ( 'NONE',  ( 0.000000000000000000, -1.000000000000000000, 0.000000000000000000 ) ) ;
#1180=CARTESIAN_POINT ( 'NONE',  ( 151.1299999999999955, -3694.430000000000291, 2239.009999999999764 ) ) ;
#1181=CARTESIAN_POINT ( 'NONE',  ( 134.0175234625681639, -3660.113920206924831, 2244.547288873641264 ) ) ;
#1183=ORIENTED_EDGE ( 'NONE', *, *, #18454, .T. ) ;
#1185=CIRCLE ( 'NONE', #9064, 3.606799999998994366 ) ;
#1192=CARTESIAN_POINT ( 'NONE',  ( 0.000000000000000000, -3695.699999999999818, 2260.600000000000364 ) ) ;
#1194=DIRECTION ( 'NONE',  ( 0.000000000000000000, 0.000000000000000000, -1.000000000000000000 ) ) ;
#1195=EDGE_CURVE ( 'NONE', #5090, #6776, #8349, .T. ) ;
#1196=CIRCLE ( 'NONE', #13926, 3.606799999999993567 ) ;
#1197=EDGE_CURVE ( 'NONE', #9068, #1906, #14089, .T. ) ;
#1198=CARTESIAN_POINT ( 'NONE',  ( 141.9794657906317070, -3657.802918816917099, 2249.014193234177128 ) ) ;
#1199=AXIS2_PLACEMENT_3D ( 'NONE', #4778, #19071, #10279 ) ;
#1201=VECTOR ( 'NONE', #1139, 1000.000000000000000 ) ;
#1202=CARTESIAN_POINT ( 'NONE',  ( 123.3932000000010021, -3670.300000000000182, 2239.009999999999764 ) ) ;
#1203=CIRCLE ( 'NONE', #2699, 2.844799999998998796 ) ;
#1207=DIRECTION ( 'NONE',  ( 0.000000000000000000, 1.000000000000000000, 0.000000000000000000 ) ) ;
#1208=ORIENTED_EDGE ( 'NONE', *, *, #17127, .F. ) ;
#1211=ADVANCED_FACE ( 'NONE', ( #4941 ), #19241, .F. ) ;
#1213=AXIS2_PLACEMENT_3D ( 'NONE', #22153, #5785, #14682 ) ;
#1214=CARTESIAN_POINT ( 'NONE',  ( 151.1299999999999955, -3694.430000000000291, 2259.329999999999927 ) ) ;
#1215=ORIENTED_EDGE ( 'NONE', *, *, #418, .T. ) ;
#1216=CARTESIAN_POINT ( 'NONE',  ( 97.99320000000000164, -3619.500000000000000, 2239.771999999999935 ) ) ;
#1224=AXIS2_PLACEMENT_3D ( 'NONE', #10858, #14615, #21755 ) ;
#1227=DIRECTION ( 'NONE',  ( 0.000000000000000000, 1.000000000000000000, 0.000000000000000000 ) ) ;
#1229=CARTESIAN_POINT ( 'NONE',  ( 10.58917828235573921, -3581.402186961769075, 2248.668793006535452 ) ) ;
#1230=CARTESIAN_POINT ( 'NONE',  ( 9.879064962501331593, -3659.930690980918371, 2250.236800000000130 ) ) ;
#1234=FACE_OUTER_BOUND ( 'NONE', #3100, .T. ) ;
#1235=EDGE_CURVE ( 'NONE', #14115, #3220, #6064, .T. ) ;
#1237=FACE_OUTER_BOUND ( 'NONE', #16909, .T. ) ;
#1238=CARTESIAN_POINT ( 'NONE',  ( 145.2534987145345440, -3660.862304053093339, 2244.636253111490532 ) ) ;
#1241=CARTESIAN_POINT ( 'NONE',  ( 11.45794194510839681, -3662.064378513683096, 2249.487216201922820 ) ) ;
#1242=CIRCLE ( 'NONE', #12846, 3.606799999999993567 ) ;
#1244=CARTESIAN_POINT ( 'NONE',  ( 151.1299999999999955, -3695.699999999999818, 2259.329999999999927 ) ) ;
#1246=CARTESIAN_POINT ( 'NONE',  ( 7.387125747139000609, -3581.600847139000052, 2246.630000000000109 ) ) ;
#1249=ADVANCED_FACE ( 'NONE', ( #5064 ), #11632, .T. ) ;
#1250=ORIENTED_EDGE ( 'NONE', *, *, #12458, .F. ) ;
#1251=CARTESIAN_POINT ( 'NONE',  ( 6.985153502415999860, -3659.505556594000154, 2244.618656866000038 ) ) ;
#1252=VERTEX_POINT ( 'NONE', #1180 ) ;
#1253=CARTESIAN_POINT ( 'NONE',  ( 1.270000000000000018, -3544.570000000000164, 2239.009999999999764 ) ) ;
#1257=DIRECTION ( 'NONE',  ( 0.000000000000000000, 0.000000000000000000, -1.000000000000000000 ) ) ;
#1259=DIRECTION ( 'NONE',  ( -1.000000000000000000, 0.000000000000000000, 0.000000000000000000 ) ) ;
#1260=CYLINDRICAL_SURFACE ( 'NONE', #5745, 2.844799999999994444 ) ;
#1262=DIRECTION ( 'NONE',  ( -1.000000000000000000, 0.000000000000000000, 0.000000000000000000 ) ) ;
#1263=B_SPLINE_CURVE_WITH_KNOTS ( 'NONE', 3,
 ( #22636, #8483, #10342, #17489, #22757, #8591, #6843, #13983, #12223, #10459, #19372, #3309, #17602, #8707, #22985, #5429, #21600, #17953, #7525, #154, #5784, #2025, #10809, #16542, #5556, #14453, #9295, #7185, #12915, #9407, #16316, #382, #20184, #7635, #3893, #9175, #1903, #495, #12687, #19835, #16428 ),
 .UNSPECIFIED., .F., .F.,
 ( 4, 2, 2, 1, 1, 2, 2, 2, 2, 1, 1, 1, 2, 2, 2, 2, 2, 2, 2, 1, 1, 2, 2, 4 ),
 ( 0.000000000000000000, 0.1249999999979331533, 0.1874999999971100062, 0.2187499999967864872, 0.2343749999967179587, 0.2421874999969684528, 0.2499999999972189468, 0.3750000000075985329, 0.4375000000129096733, 0.4687500000155650492, 0.4843750000170347070, 0.4921875000177692860, 0.4960937500180022108, 0.5000000000182350801, 0.5625000000188430382, 0.5937500000189966931, 0.6250000000191502370, 0.6875000000194086969, 0.7187500000195379268, 0.7343750000196028749, 0.7421875000200089945, 0.7460937500199683603, 0.7500000000199277261, 1.000000000000000000 ),
 .UNSPECIFIED. ) ;
#1264=ORIENTED_EDGE ( 'NONE', *, *, #19451, .F. ) ;
#1265=AXIS2_PLACEMENT_3D ( 'NONE', #6682, #19325, #16038 ) ;
#1268=AXIS2_PLACEMENT_3D ( 'NONE', #17644, #3353, #21409 ) ;
#1270=DIRECTION ( 'NONE',  ( 0.000000000000000000, 0.000000000000000000, -1.000000000000000000 ) ) ;
#1271=CARTESIAN_POINT ( 'NONE',  ( 9.916981607687798572, -3658.814059329320116, 2249.942683905858303 ) ) ;
#1272=ORIENTED_EDGE ( 'NONE', *, *, #10390, .F. ) ;
#1278=ORIENTED_EDGE ( 'NONE', *, *, #4244, .T. ) ;
#1279=CARTESIAN_POINT ( 'NONE',  ( 18.37893127878000143, -3660.140301727999940, 2244.547200027999679 ) ) ;
#1282=ORIENTED_EDGE ( 'NONE', *, *, #9851, .T. ) ;
#1284=VECTOR ( 'NONE', #17170, 1000.000000000000000 ) ;
#1286=VECTOR ( 'NONE', #7795, 1000.000000000000000 ) ;
#1287=AXIS2_PLACEMENT_3D ( 'NONE', #5797, #5569, #16104 ) ;
#1288=FACE_OUTER_BOUND ( 'NONE', #22159, .T. ) ;
#1289=DIRECTION ( 'NONE',  ( 0.000000000000000000, 0.000000000000000000, 1.000000000000000000 ) ) ;
#1290=CARTESIAN_POINT ( 'NONE',  ( 134.1335424281758435, -3658.210520966862987, 2245.301510576022338 ) ) ;
#1291=DIRECTION ( 'NONE',  ( -1.000000000000000000, 0.000000000000000000, 0.000000000000000000 ) ) ;
#1296=EDGE_LOOP ( 'NONE', ( #17068, #11898, #4290, #1902 ) ) ;
#1297=CARTESIAN_POINT ( 'NONE',  ( 127.0000000000000000, -3568.700000000000273, 2259.837999999999738 ) ) ;
#1299=CIRCLE ( 'NONE', #3937, 1.269999999999993356 ) ;
#1305=ORIENTED_EDGE ( 'NONE', *, *, #6122, .F. ) ;
#1308=CARTESIAN_POINT ( 'NONE',  ( 104.4447999999999865, -3670.300000000000182, 2261.869999999999891 ) ) ;
#1312=CARTESIAN_POINT ( 'NONE',  ( 95.25000000000000000, -3544.570000000000164, 2251.506800000000112 ) ) ;
#1313=CARTESIAN_POINT ( 'NONE',  ( 114.2999999999999972, -3594.099999999999909, 2260.600000000000364 ) ) ;
#1314=AXIS2_PLACEMENT_3D ( 'NONE', #4707, #20997, #12205 ) ;
#1317=CARTESIAN_POINT ( 'NONE',  ( 141.8962106656137223, -3657.696406372347610, 2248.849616286249784 ) ) ;
#1318=CIRCLE ( 'NONE', #23015, 1.269999999999882334 ) ;
#1319=ORIENTED_EDGE ( 'NONE', *, *, #10226, .T. ) ;
#1320=AXIS2_PLACEMENT_3D ( 'NONE', #13380, #12199, #15718 ) ;
#1324=DIRECTION ( 'NONE',  ( 1.000000000000000000, 0.000000000000000000, 0.000000000000000000 ) ) ;
#1328=CARTESIAN_POINT ( 'NONE',  ( 4.771025910096229339, -3543.400907226851814, 2259.826090471561656 ) ) ;
#1332=VECTOR ( 'NONE', #11913, 1000.000000000000000 ) ;
#1333=DIRECTION ( 'NONE',  ( -1.000000000000000000, 0.000000000000000000, 0.000000000000000000 ) ) ;
#1334=EDGE_CURVE ( 'NONE', #928, #5746, #19520, .T. ) ;
#1336=CIRCLE ( 'NONE', #593, 0.7619999999999987894 ) ;
#1337=DIRECTION ( 'NONE',  ( 0.000000000000000000, 0.000000000000000000, -1.000000000000000000 ) ) ;
#1341=CARTESIAN_POINT ( 'NONE',  ( 41.70680000000000121, -3594.099999999999909, 2239.009999999999764 ) ) ;
#1342=TOROIDAL_SURFACE ( 'NONE', #7346, 4.114799999999999791, 1.270000000000000018 ) ;
#1346=EDGE_CURVE ( 'NONE', #10418, #1443, #22133, .T. ) ;
#1348=CARTESIAN_POINT ( 'NONE',  ( 10.56087945680325113, -3581.370517028351969, 2248.730192196002918 ) ) ;
#1349=CARTESIAN_POINT ( 'NONE',  ( 98.75520000000000209, -3670.300000000000182, 2259.837999999999738 ) ) ;
#1351=ORIENTED_EDGE ( 'NONE', *, *, #1766, .T. ) ;
#1352=DIRECTION ( 'NONE',  ( 1.000000000000000000, 0.000000000000000000, 0.000000000000000000 ) ) ;
#1353=EDGE_CURVE ( 'NONE', #20927, #5223, #20628, .T. ) ;
#1356=CARTESIAN_POINT ( 'NONE',  ( 145.2869493186738907, -3660.716514101495250, 2244.602361446073246 ) ) ;
#1357=CARTESIAN_POINT ( 'NONE',  ( 131.8733694595999850, -3694.556024844999683, 2260.595783923999988 ) ) ;
#1360=CARTESIAN_POINT ( 'NONE',  ( 147.4837675257009550, -3543.632335307654103, 2260.189864799524003 ) ) ;
#1361=AXIS2_PLACEMENT_3D ( 'NONE', #1007, #1119, #19060 ) ;
#1362=ORIENTED_EDGE ( 'NONE', *, *, #10523, .F. ) ;
#1367=LINE ( 'NONE', #6541, #15671 ) ;
#1369=DIRECTION ( 'NONE',  ( 0.000000000000000000, 0.000000000000000000, -1.000000000000000000 ) ) ;
#1374=ORIENTED_EDGE ( 'NONE', *, *, #10850, .T. ) ;
#1384=CARTESIAN_POINT ( 'NONE',  ( 139.6999999999999886, -3579.494999999999891, 2272.030000000000200 ) ) ;
#1385=DIRECTION ( 'NONE',  ( 0.000000000000000000, -1.000000000000000000, 0.000000000000000000 ) ) ;
#1387=ORIENTED_EDGE ( 'NONE', *, *, #9099, .T. ) ;
#1389=AXIS2_PLACEMENT_3D ( 'NONE', #7265, #4, #3976 ) ;
#1390=DIRECTION ( 'NONE',  ( -1.000000000000000000, 0.000000000000000000, 0.000000000000000000 ) ) ;
#1391=ORIENTED_EDGE ( 'NONE', *, *, #15719, .F. ) ;
#1392=DIRECTION ( 'NONE',  ( 0.000000000000000000, 1.000000000000000000, 0.000000000000000000 ) ) ;
#1393=CARTESIAN_POINT ( 'NONE',  ( 10.31040564863712561, -3657.961501593514186, 2249.221529667188406 ) ) ;
#1395=AXIS2_PLACEMENT_3D ( 'NONE', #9735, #13373, #16539 ) ;
#1397=FACE_OUTER_BOUND ( 'NONE', #9744, .T. ) ;
#1400=CARTESIAN_POINT ( 'NONE',  ( 151.4000000000000057, -3578.860000000000127, 2247.392000000000280 ) ) ;
#1401=EDGE_CURVE ( 'NONE', #17090, #13554, #12783, .T. ) ;
#1403=EDGE_CURVE ( 'NONE', #16556, #1252, #14309, .T. ) ;
#1404=DIRECTION ( 'NONE',  ( 0.000000000000000000, 0.000000000000000000, -1.000000000000000000 ) ) ;
#1405=ORIENTED_EDGE ( 'NONE', *, *, #17358, .F. ) ;
#1406=CARTESIAN_POINT ( 'NONE',  ( 151.1299999999999955, -3694.430000000000291, 2260.600000000000364 ) ) ;
#1410=ADVANCED_FACE ( 'NONE', ( #22 ), #13541, .T. ) ;
#1412=CARTESIAN_POINT ( 'NONE',  ( 134.2370284977077688, -3657.825934259354199, 2245.736048003489941 ) ) ;
#1413=CARTESIAN_POINT ( 'NONE',  ( 50.79999999999999716, -3568.700000000000273, 2239.009999999999764 ) ) ;
#1415=DIRECTION ( 'NONE',  ( 0.000000000000000000, 0.000000000000000000, -1.000000000000000000 ) ) ;
#1417=EDGE_CURVE ( 'NONE', #10346, #15928, #14322, .T. ) ;
#1420=DIRECTION ( 'NONE',  ( 0.000000000000000000, 0.000000000000000000, 1.000000000000000000 ) ) ;
#1422=CIRCLE ( 'NONE', #8122, 0.7619999999999987894 ) ;
#1427=ORIENTED_EDGE ( 'NONE', *, *, #3952, .T. ) ;
#1429=CARTESIAN_POINT ( 'NONE',  ( 134.3871257472000025, -3657.399152860999493, 2246.630000000000109 ) ) ;
#1432=CARTESIAN_POINT ( 'NONE',  ( 47.95519999999999783, -3568.700000000000273, 2239.771999999999935 ) ) ;
#1434=DIRECTION ( 'NONE',  ( 1.000000000000000000, 0.000000000000000000, 0.000000000000000000 ) ) ;
#1435=FACE_OUTER_BOUND ( 'NONE', #2011, .T. ) ;
#1436=CARTESIAN_POINT ( 'NONE',  ( 41.70680000000000121, -3644.899999999999636, 2239.771999999999935 ) ) ;
#1437=CARTESIAN_POINT ( 'NONE',  ( 141.5035269015962172, -3657.304818365388655, 2247.157352627789805 ) ) ;
#1443=VERTEX_POINT ( 'NONE', #14902 ) ;
#1446=VERTEX_POINT ( 'NONE', #2577 ) ;
#1447=DIRECTION ( 'NONE',  ( 1.000000000000000000, 0.000000000000000000, 0.000000000000000000 ) ) ;
#1449=FACE_OUTER_BOUND ( 'NONE', #20289, .T. ) ;
#1452=DIRECTION ( 'NONE',  ( 0.000000000000000000, 0.000000000000000000, -1.000000000000000000 ) ) ;
#1453=CARTESIAN_POINT ( 'NONE',  ( 117.1447999999989946, -3594.099999999999909, 2239.771999999999935 ) ) ;
#1455=TOROIDAL_SURFACE ( 'NONE', #2594, 3.606799999998999695, 0.7620000000000000107 ) ;
#1460=ORIENTED_EDGE ( 'NONE', *, *, #22126, .T. ) ;
#1461=CARTESIAN_POINT ( 'NONE',  ( 1.270000000000000018, -3694.430000000000291, 2260.600000000000364 ) ) ;
#1462=CARTESIAN_POINT ( 'NONE',  ( 10.04341343045742541, -3580.512822074882479, 2249.707644168996922 ) ) ;
#1463=EDGE_CURVE ( 'NONE', #4904, #18111, #16635, .T. ) ;
#1464=DIRECTION ( 'NONE',  ( 0.000000000000000000, 0.000000000000000000, 1.000000000000000000 ) ) ;
#1465=ORIENTED_EDGE ( 'NONE', *, *, #10304, .F. ) ;
#1466=DIRECTION ( 'NONE',  ( 1.000000000000000000, 0.000000000000000000, 0.000000000000000000 ) ) ;
#1467=AXIS2_PLACEMENT_3D ( 'NONE', #19170, #6756, #21048 ) ;
#1470=DIRECTION ( 'NONE',  ( -1.000000000000000000, 0.000000000000000000, 0.000000000000000000 ) ) ;
#1471=DIRECTION ( 'NONE',  ( 0.000000000000000000, 0.000000000000000000, -1.000000000000000000 ) ) ;
#1472=CARTESIAN_POINT ( 'NONE',  ( 10.56659506800342641, -3661.386912547712200, 2249.948988271942653 ) ) ;
#1473=CARTESIAN_POINT ( 'NONE',  ( 147.4427523029042106, -3543.741058431988222, 2260.292570800639169 ) ) ;
#1477=CARTESIAN_POINT ( 'NONE',  ( 73.35520000000001062, -3670.300000000000182, 2261.869999999999891 ) ) ;
#1478=CARTESIAN_POINT ( 'NONE',  ( 25.39999999999999858, -3670.300000000000182, 2261.869999999999891 ) ) ;
#1479=ORIENTED_EDGE ( 'NONE', *, *, #17226, .F. ) ;
#1480=ORIENTED_EDGE ( 'NONE', *, *, #7960, .T. ) ;
#1481=VECTOR ( 'NONE', #692, 1000.000000000000000 ) ;
#1486=CARTESIAN_POINT ( 'NONE',  ( 9.847598318245756488, -3543.397347667041686, 2254.991658123818070 ) ) ;
#1494=CARTESIAN_POINT ( 'NONE',  ( 136.6529205195000145, -3695.699999999999818, 2254.503999999999905 ) ) ;
#1505=AXIS2_PLACEMENT_3D ( 'NONE', #8930, #373, #10574 ) ;
#1507=CIRCLE ( 'NONE', #14628, 5.715000000001058567 ) ;
#1508=CARTESIAN_POINT ( 'NONE',  ( 134.1443423388099063, -3580.833646875505110, 2245.342901023084778 ) ) ;
#1510=VERTEX_POINT ( 'NONE', #5994 ) ;
#1517=CARTESIAN_POINT ( 'NONE',  ( 131.7616391464439971, -3695.609040584405193, 2259.802577514632958 ) ) ;
#1521=CARTESIAN_POINT ( 'NONE',  ( 15.45570990063155392, -3580.206700319643460, 2249.899904268654154 ) ) ;
#1523=CARTESIAN_POINT ( 'NONE',  ( 50.79999999999999716, -3619.500000000000000, 2239.771999999999935 ) ) ;
#1525=CARTESIAN_POINT ( 'NONE',  ( 151.1299999999999955, -3694.430000000000291, 2240.279999999999745 ) ) ;
#1527=ORIENTED_EDGE ( 'NONE', *, *, #18311, .F. ) ;
#1528=CARTESIAN_POINT ( 'NONE',  ( 28.24479999999899604, -3619.500000000000000, 2261.869999999999891 ) ) ;
#1529=EDGE_CURVE ( 'NONE', #4464, #10440, #9436, .T. ) ;
#1530=CIRCLE ( 'NONE', #15007, 0.7619999999999294005 ) ;
#1531=EDGE_CURVE ( 'NONE', #14575, #12638, #18031, .T. ) ;
#1534=LINE ( 'NONE', #20757, #22196 ) ;
#1538=CARTESIAN_POINT ( 'NONE',  ( 127.0000000000000000, -3619.500000000000000, 2261.869999999999891 ) ) ;
#1541=VERTEX_POINT ( 'NONE', #597 ) ;
#1546=CARTESIAN_POINT ( 'NONE',  ( 136.9109231113999954, -3578.930102841999997, 2250.236803302000226 ) ) ;
#1552=CARTESIAN_POINT ( 'NONE',  ( 9.851292762693375948, -3695.598810868125383, 2255.000759462867791 ) ) ;
#1554=CARTESIAN_POINT ( 'NONE',  ( 0.000000000000000000, -3694.430000000000291, 2259.329999999999927 ) ) ;
#1560=ORIENTED_EDGE ( 'NONE', *, *, #14314, .F. ) ;
#1563=DIRECTION ( 'NONE',  ( 0.000000000000000000, 0.000000000000000000, 1.000000000000000000 ) ) ;
#1565=ORIENTED_EDGE ( 'NONE', *, *, #18959, .T. ) ;
#1568=CARTESIAN_POINT ( 'NONE',  ( 76.20000000000000284, -3670.300000000000182, 2261.869999999999891 ) ) ;
#1572=CARTESIAN_POINT ( 'NONE',  ( 25.39999999999999858, -3670.300000000000182, 2239.009999999999764 ) ) ;
#1573=FACE_BOUND ( 'NONE', #14091, .T. ) ;
#1576=AXIS2_PLACEMENT_3D ( 'NONE', #17280, #8391, #4865 ) ;
#1581=DIRECTION ( 'NONE',  ( 1.000000000000000000, 0.000000000000000000, 0.000000000000000000 ) ) ;
#1583=CARTESIAN_POINT ( 'NONE',  ( 10.57556485081456898, -3581.387054496447035, 2248.698531430067760 ) ) ;
#1585=ORIENTED_EDGE ( 'NONE', *, *, #14722, .T. ) ;
#1586=CARTESIAN_POINT ( 'NONE',  ( 76.20000000000000284, -3670.300000000000182, 2239.771999999999935 ) ) ;
#1588=FACE_BOUND ( 'NONE', #11357, .T. ) ;
#1590=AXIS2_PLACEMENT_3D ( 'NONE', #15714, #9850, #22843 ) ;
#1591=CARTESIAN_POINT ( 'NONE',  ( 11.62623776245822249, -3662.139701344950481, 2249.415671503285921 ) ) ;
#1592=DIRECTION ( 'NONE',  ( 1.000000000000000000, 0.000000000000000000, 0.000000000000000000 ) ) ;
#1594=CARTESIAN_POINT ( 'NONE',  ( 35.56000000000000227, -3695.699999999999818, 2251.506800000000112 ) ) ;
#1598=CARTESIAN_POINT ( 'NONE',  ( 14.52771269207012850, -3657.324844698252491, 2247.803865992611463 ) ) ;
#1600=ORIENTED_EDGE ( 'NONE', *, *, #16524, .F. ) ;
#1601=CARTESIAN_POINT ( 'NONE',  ( 147.3199999999999932, -3544.570000000000164, 2260.600000000000364 ) ) ;
#1605=CIRCLE ( 'NONE', #15833, 0.7619999999999987894 ) ;
#1608=DIRECTION ( 'NONE',  ( 0.000000000000000000, 1.000000000000000000, 0.000000000000000000 ) ) ;
#1610=DIRECTION ( 'NONE',  ( 0.7249994335945011414, 0.000000000000000000, -0.6887494619146010688 ) ) ;
#1612=AXIS2_PLACEMENT_3D ( 'NONE', #19935, #10675, #3875 ) ;
#1617=DIRECTION ( 'NONE',  ( -1.000000000000000000, -0.000000000000000000, -0.000000000000000000 ) ) ;
#1618=ORIENTED_EDGE ( 'NONE', *, *, #434, .T. ) ;
#1619=DIRECTION ( 'NONE',  ( 0.000000000000000000, 0.000000000000000000, -1.000000000000000000 ) ) ;
#1620=CIRCLE ( 'NONE', #11354, 2.844799999999009010 ) ;
#1621=EDGE_CURVE ( 'NONE', #10003, #16281, #13024, .T. ) ;
#1624=DIRECTION ( 'NONE',  ( 0.000000000000000000, 0.000000000000000000, 1.000000000000000000 ) ) ;
#1625=EDGE_CURVE ( 'NONE', #7999, #4345, #19946, .T. ) ;
#1627=ORIENTED_EDGE ( 'NONE', *, *, #333, .F. ) ;
#1629=VECTOR ( 'NONE', #3520, 999.9999999999998863 ) ;
#1630=LINE ( 'NONE', #15473, #15052 ) ;
#1635=EDGE_CURVE ( 'NONE', #20696, #7575, #5699, .T. ) ;
#1637=VECTOR ( 'NONE', #5851, 1000.000000000000114 ) ;
#1640=EDGE_CURVE ( 'NONE', #17185, #6183, #20730, .T. ) ;
#1642=EDGE_LOOP ( 'NONE', ( #22112, #11847, #7529, #9622 ) ) ;
#1647=CARTESIAN_POINT ( 'NONE',  ( 5.032733771186362226, -3695.066554911154071, 2260.481515824936196 ) ) ;
#1649=CARTESIAN_POINT ( 'NONE',  ( 0.000000000000000000, -3544.570000000000164, 2259.329999999999927 ) ) ;
#1652=LINE ( 'NONE', #5299, #6943 ) ;
#1654=ORIENTED_EDGE ( 'NONE', *, *, #17458, .T. ) ;
#1656=EDGE_CURVE ( 'NONE', #9562, #2027, #3807, .T. ) ;
#1657=CARTESIAN_POINT ( 'NONE',  ( 91.74479999999999791, -3594.099999999999909, 2261.869999999999891 ) ) ;
#1660=AXIS2_PLACEMENT_3D ( 'NONE', #20002, #313, #3934 ) ;
#1661=DIRECTION ( 'NONE',  ( 0.000000000000000000, 0.000000000000000000, -1.000000000000000000 ) ) ;
#1664=ADVANCED_FACE ( 'NONE', ( #1397 ), #10921, .T. ) ;
#1668=CARTESIAN_POINT ( 'NONE',  ( 137.1312382075398375, -3658.282264947529711, 2249.547148403314168 ) ) ;
#1670=ORIENTED_EDGE ( 'NONE', *, *, #1640, .T. ) ;
#1671=CIRCLE ( 'NONE', #20758, 4.114799999999974034 ) ;
#1672=CARTESIAN_POINT ( 'NONE',  ( 137.0047131064691541, -3660.427569099905668, 2250.225733703707192 ) ) ;
#1673=AXIS2_PLACEMENT_3D ( 'NONE', #5293, #20908, #17823 ) ;
#1675=EDGE_LOOP ( 'NONE', ( #17011, #16139 ) ) ;
#1676=AXIS2_PLACEMENT_3D ( 'NONE', #11507, #20525, #17009 ) ;
#1677=VERTEX_POINT ( 'NONE', #22829 ) ;
#1679=EDGE_CURVE ( 'NONE', #15928, #21490, #19108, .T. ) ;
#1681=ORIENTED_EDGE ( 'NONE', *, *, #21603, .T. ) ;
#1682=EDGE_LOOP ( 'NONE', ( #12031, #5258, #388, #6450 ) ) ;
#1683=DIRECTION ( 'NONE',  ( 0.000000000000000000, 0.000000000000000000, 1.000000000000000000 ) ) ;
#1685=DIRECTION ( 'NONE',  ( 0.000000000000000000, 0.000000000000000000, -1.000000000000000000 ) ) ;
#1686=DIRECTION ( 'NONE',  ( 0.000000000000000000, 0.000000000000000000, 1.000000000000000000 ) ) ;
#1689=FACE_BOUND ( 'NONE', #7308, .T. ) ;
#1691=AXIS2_PLACEMENT_3D ( 'NONE', #4081, #3644, #679 ) ;
#1692=AXIS2_PLACEMENT_3D ( 'NONE', #3746, #18052, #11019 ) ;
#1693=CARTESIAN_POINT ( 'NONE',  ( 47.19319999999999737, -3670.300000000000182, 2239.009999999999764 ) ) ;
#1697=EDGE_CURVE ( 'NONE', #13127, #5536, #12054, .T. ) ;
#1699=AXIS2_PLACEMENT_3D ( 'NONE', #5913, #4591, #8121 ) ;
#1700=CARTESIAN_POINT ( 'NONE',  ( 9.855258736895999405, -3579.517414328000086, 2250.159819663000235 ) ) ;
#1704=ADVANCED_FACE ( 'NONE', ( #3616 ), #15056, .T. ) ;
#1705=ORIENTED_EDGE ( 'NONE', *, *, #23112, .F. ) ;
#1706=DIRECTION ( 'NONE',  ( 1.000000000000000000, 0.000000000000000000, 0.000000000000000000 ) ) ;
#1709=FACE_OUTER_BOUND ( 'NONE', #21775, .T. ) ;
#1710=CARTESIAN_POINT ( 'NONE',  ( 132.0286855373999799, -3694.758336080999925, 2260.557504193999648 ) ) ;
#1711=AXIS2_PLACEMENT_3D ( 'NONE', #4187, #3961, #11332 ) ;
#1712=EDGE_CURVE ( 'NONE', #1677, #10545, #1185, .T. ) ;
#1717=AXIS2_PLACEMENT_3D ( 'NONE', #22465, #4786, #11930 ) ;
#1720=AXIS2_PLACEMENT_3D ( 'NONE', #22933, #19555, #21082 ) ;
#1721=ORIENTED_EDGE ( 'NONE', *, *, #11917, .F. ) ;
#1726=CARTESIAN_POINT ( 'NONE',  ( 15.17971944497489467, -3658.110408443104006, 2249.386264408048191 ) ) ;
#1727=CARTESIAN_POINT ( 'NONE',  ( 136.8052632656678895, -3695.644174308496986, 2254.886265309746705 ) ) ;
#1728=EDGE_LOOP ( 'NONE', ( #22366, #22048, #22055, #11818 ) ) ;
#1730=ORIENTED_EDGE ( 'NONE', *, *, #19464, .T. ) ;
#1731=AXIS2_PLACEMENT_3D ( 'NONE', #15996, #10603, #15649 ) ;
#1733=CIRCLE ( 'NONE', #21933, 2.844799999999994444 ) ;
#1738=DIRECTION ( 'NONE',  ( 0.000000000000000000, 0.000000000000000000, -1.000000000000000000 ) ) ;
#1741=CARTESIAN_POINT ( 'NONE',  ( 72.56166137651000270, -3694.430000000000291, 2315.390696186000241 ) ) ;
#1744=EDGE_LOOP ( 'NONE', ( #17388, #21682, #4617, #3315 ) ) ;
#1746=DIRECTION ( 'NONE',  ( 0.000000000000000000, 0.000000000000000000, 1.000000000000000000 ) ) ;
#1747=ORIENTED_EDGE ( 'NONE', *, *, #9104, .F. ) ;
#1750=EDGE_LOOP ( 'NONE', ( #12144, #21234 ) ) ;
#1751=DIRECTION ( 'NONE',  ( 0.000000000000000000, -1.000000000000000000, 0.000000000000000000 ) ) ;
#1752=CARTESIAN_POINT ( 'NONE',  ( 142.4995878314999800, -3660.024017658000048, 2250.236800000000130 ) ) ;
#1754=ORIENTED_EDGE ( 'NONE', *, *, #20889, .F. ) ;
#1755=ORIENTED_EDGE ( 'NONE', *, *, #21279, .T. ) ;
#1756=CARTESIAN_POINT ( 'NONE',  ( 137.3720204532196476, -3581.130476171526880, 2249.106963701437962 ) ) ;
#1760=DIRECTION ( 'NONE',  ( 0.000000000000000000, 1.000000000000000000, 0.000000000000000000 ) ) ;
#1761=DIRECTION ( 'NONE',  ( 0.000000000000000000, 1.000000000000000000, 0.000000000000000000 ) ) ;
#1762=CIRCLE ( 'NONE', #21961, 4.114799999999974034 ) ;
#1764=LINE ( 'NONE', #6929, #9474 ) ;
#1766=EDGE_CURVE ( 'NONE', #3129, #11209, #9784, .T. ) ;
#1767=ADVANCED_FACE ( 'NONE', ( #21439 ), #16047, .F. ) ;
#1771=EDGE_CURVE ( 'NONE', #16761, #3671, #22510, .T. ) ;
#1775=CARTESIAN_POINT ( 'NONE',  ( 4.742867852766174508, -3695.626565543418110, 2259.755970531261028 ) ) ;
#1777=CARTESIAN_POINT ( 'NONE',  ( 20.12315942192000051, -3544.527728670999750, 2260.413001451000127 ) ) ;
#1779=EDGE_CURVE ( 'NONE', #17500, #17093, #15210, .T. ) ;
#1780=CARTESIAN_POINT ( 'NONE',  ( 139.6999999999999886, -3659.504999999999654, 2255.774000000000342 ) ) ;
#1784=CARTESIAN_POINT ( 'NONE',  ( 72.59320000000001016, -3568.700000000000273, 2239.009999999999764 ) ) ;
#1785=CARTESIAN_POINT ( 'NONE',  ( 17.56231070083699208, -3576.491783798367123, 2245.815664034199017 ) ) ;
#1786=DIRECTION ( 'NONE',  ( -1.000000000000000000, 0.000000000000000000, 0.000000000000000000 ) ) ;
#1788=ORIENTED_EDGE ( 'NONE', *, *, #11296, .T. ) ;
#1790=LINE ( 'NONE', #12796, #22343 ) ;
#1791=DIRECTION ( 'NONE',  ( 1.000000000000000000, 0.000000000000000000, 0.000000000000000000 ) ) ;
#1793=CARTESIAN_POINT ( 'NONE',  ( 21.79320000000099711, -3619.500000000000000, 2239.009999999999764 ) ) ;
#1796=ORIENTED_EDGE ( 'NONE', *, *, #7379, .T. ) ;
#1800=TOROIDAL_SURFACE ( 'NONE', #4406, 3.606799999998999695, 0.7620000000000000107 ) ;
#1804=CARTESIAN_POINT ( 'NONE',  ( 9.855190710340998805, -3579.429666650000399, 2250.179986546000237 ) ) ;
#1805=EDGE_LOOP ( 'NONE', ( #15141, #9589 ) ) ;
#1813=EDGE_CURVE ( 'NONE', #8599, #17497, #4946, .T. ) ;
#1817=CARTESIAN_POINT ( 'NONE',  ( 131.9229944970066413, -3543.650737883654983, 2260.206970375517358 ) ) ;
#1818=B_SPLINE_CURVE_WITH_KNOTS ( 'NONE', 3,
 ( #19225, #10427, #12068, #14068, #6698, #8330, #12189, #22605, #4806, #20866, #11841, #15822, #17567, #15475, #8452, #6582, #1517, #13723, #11954, #10312, #13950, #15598, #5043, #21099 ),
 .UNSPECIFIED., .F., .F.,
 ( 4, 2, 2, 1, 1, 2, 2, 2, 2, 1, 1, 2, 2, 4 ),
 ( 0.000000000000000000, 0.2499999999966758257, 0.3749999999947900564, 0.4374999999941148743, 0.4687499999937840278, 0.4843749999938956052, 0.4999999999940071271, 0.6249999999889135349, 0.6874999999858730781, 0.7187499999848055987, 0.7343749999842796861, 0.7421874999841302500, 0.7499999999839809250, 1.000000000000000000 ),
 .UNSPECIFIED. ) ;
#1823=FACE_BOUND ( 'NONE', #15815, .T. ) ;
#1825=LINE ( 'NONE', #1944, #3225 ) ;
#1826=B_SPLINE_CURVE_WITH_KNOTS ( 'NONE', 3,
 ( #22448, #6422, #17298, #1246 ),
 .UNSPECIFIED., .F., .F.,
 ( 4, 4 ),
 ( 0.000000000000000000, 1.000000000000000000 ),
 .UNSPECIFIED. ) ;
#1827=SPHERICAL_SURFACE ( 'NONE', #8869, 1.270000000000000018 ) ;
#1828=DIRECTION ( 'NONE',  ( -1.000000000000000000, 0.000000000000000000, 0.000000000000000000 ) ) ;
#1829=ORIENTED_EDGE ( 'NONE', *, *, #6722, .F. ) ;
#1830=EDGE_CURVE ( 'NONE', #15313, #17962, #22150, .T. ) ;
#1835=CIRCLE ( 'NONE', #13419, 2.844800000000091700 ) ;
#1837=CYLINDRICAL_SURFACE ( 'NONE', #16065, 0.7619999999999294005 ) ;
#1838=CARTESIAN_POINT ( 'NONE',  ( 14.50450911876278148, -3657.305732182916017, 2247.637440964547750 ) ) ;
#1840=VERTEX_POINT ( 'NONE', #15931 ) ;
#1841=EDGE_CURVE ( 'NONE', #22341, #20273, #10934, .T. ) ;
#1842=CARTESIAN_POINT ( 'NONE',  ( 10.62015369107034424, -3577.553924892425584, 2249.919332792890145 ) ) ;
#1850=EDGE_CURVE ( 'NONE', #11364, #15707, #9804, .T. ) ;
#1852=CARTESIAN_POINT ( 'NONE',  ( 1.270000000000000018, -3695.699999999999818, 2259.329999999999927 ) ) ;
#1853=VECTOR ( 'NONE', #12847, 1000.000000000000114 ) ;
#1854=DIRECTION ( 'NONE',  ( 0.000000000000000000, -1.000000000000000000, 0.000000000000000000 ) ) ;
#1856=VERTEX_POINT ( 'NONE', #6194 ) ;
#1857=CARTESIAN_POINT ( 'NONE',  ( 114.2999999999999972, -3644.899999999999636, 2261.869999999999891 ) ) ;
#1861=DIRECTION ( 'NONE',  ( -1.000000000000000000, 0.000000000000000000, 0.000000000000000000 ) ) ;
#1863=CARTESIAN_POINT ( 'NONE',  ( 142.3769745404992477, -3695.298184790463893, 2255.430976451231345 ) ) ;
#1866=TOROIDAL_SURFACE ( 'NONE', #21327, 3.606799999999999784, 0.7620000000000000107 ) ;
#1868=CARTESIAN_POINT ( 'NONE',  ( 137.6222368942718219, -3581.439509223405366, 2248.597413845674510 ) ) ;
#1870=DIRECTION ( 'NONE',  ( 0.000000000000000000, 1.000000000000000000, 0.000000000000000000 ) ) ;
#1872=DIRECTION ( 'NONE',  ( -1.000000000000000000, 0.000000000000000000, 0.000000000000000000 ) ) ;
#1873=DIRECTION ( 'NONE',  ( 0.000000000000000000, -1.000000000000000000, 0.000000000000000000 ) ) ;
#1874=CIRCLE ( 'NONE', #7493, 3.606799999999993567 ) ;
#1878=CARTESIAN_POINT ( 'NONE',  ( 140.6533150761702586, -3576.814124183825697, 2249.368845734366005 ) ) ;
#1879=ORIENTED_EDGE ( 'NONE', *, *, #16323, .T. ) ;
#1880=CARTESIAN_POINT ( 'NONE',  ( 134.6950185071150088, -3576.735968958820195, 2245.499284827320935 ) ) ;
#1882=VERTEX_POINT ( 'NONE', #7597 ) ;
#1883=DIRECTION ( 'NONE',  ( 0.000000000000000000, 0.000000000000000000, 1.000000000000000000 ) ) ;
#1884=DIRECTION ( 'NONE',  ( 0.000000000000000000, -1.000000000000000000, 0.000000000000000000 ) ) ;
#1887=CARTESIAN_POINT ( 'NONE',  ( 133.9849999999999852, -3659.504999999999654, 2246.630000000000109 ) ) ;
#1889=ORIENTED_EDGE ( 'NONE', *, *, #21889, .F. ) ;
#1892=EDGE_CURVE ( 'NONE', #2232, #15313, #4213, .T. ) ;
#1899=AXIS2_PLACEMENT_3D ( 'NONE', #23040, #8324, #3360 ) ;
#1902=ORIENTED_EDGE ( 'NONE', *, *, #10950, .T. ) ;
#1903=CARTESIAN_POINT ( 'NONE',  ( 18.12377227050810546, -3581.296112607328268, 2245.922901418339279 ) ) ;
#1904=CARTESIAN_POINT ( 'NONE',  ( 95.25000000000000000, -3670.300000000000182, 2247.392000000000280 ) ) ;
#1905=CIRCLE ( 'NONE', #20993, 5.715000000000872937 ) ;
#1906=VERTEX_POINT ( 'NONE', #2553 ) ;
#1908=CARTESIAN_POINT ( 'NONE',  ( 137.7820634117503573, -3661.606662391098325, 2249.829843942283787 ) ) ;
#1913=ORIENTED_EDGE ( 'NONE', *, *, #14986, .T. ) ;
#1917=ORIENTED_EDGE ( 'NONE', *, *, #22733, .F. ) ;
#1920=PLANE ( 'NONE',  #10661 ) ;
#1921=AXIS2_PLACEMENT_3D ( 'NONE', #21651, #8883, #3947 ) ;
#1922=FACE_OUTER_BOUND ( 'NONE', #4676, .T. ) ;
#1923=VERTEX_POINT ( 'NONE', #6082 ) ;
#1934=CARTESIAN_POINT ( 'NONE',  ( 9.855190710340998805, -3579.495000415000050, 2250.165025612000136 ) ) ;
#1939=AXIS2_PLACEMENT_3D ( 'NONE', #6032, #848, #21956 ) ;
#1942=EDGE_CURVE ( 'NONE', #15342, #6713, #6833, .T. ) ;
#1944=CARTESIAN_POINT ( 'NONE',  ( 151.1299999999999955, -3544.570000000000164, 2239.009999999999764 ) ) ;
#1945=CARTESIAN_POINT ( 'NONE',  ( 91.74479999999999791, -3594.099999999999909, 2259.837999999999738 ) ) ;
#1947=CARTESIAN_POINT ( 'NONE',  ( 147.6742428626672563, -3543.355825688684035, 2259.712068108529820 ) ) ;
#1949=CARTESIAN_POINT ( 'NONE',  ( 147.8270794805000037, -3695.699999999999818, 2259.329999999999927 ) ) ;
#1950=DIRECTION ( 'NONE',  ( 0.000000000000000000, 0.000000000000000000, 1.000000000000000000 ) ) ;
#1951=CARTESIAN_POINT ( 'NONE',  ( 57.14999999999999858, -3544.570000000000164, 2243.277199999999993 ) ) ;
#1952=DIRECTION ( 'NONE',  ( 0.000000000000000000, 0.000000000000000000, -1.000000000000000000 ) ) ;
#1953=CARTESIAN_POINT ( 'NONE',  ( 142.5418842717801340, -3543.408637598919540, 2255.017974340328692 ) ) ;
#1954=DIRECTION ( 'NONE',  ( 0.000000000000000000, 0.000000000000000000, -1.000000000000000000 ) ) ;
#1957=CARTESIAN_POINT ( 'NONE',  ( 7.430466206498319792, -3577.282607159902909, 2245.023857075259002 ) ) ;
#1961=AXIS2_PLACEMENT_3D ( 'NONE', #7484, #7261, #9252 ) ;
#1962=DIRECTION ( 'NONE',  ( 0.000000000000000000, 0.000000000000000000, 1.000000000000000000 ) ) ;
#1965=EDGE_CURVE ( 'NONE', #11744, #3669, #1203, .T. ) ;
#1967=EDGE_CURVE ( 'NONE', #21948, #140, #105, .T. ) ;
#1969=CARTESIAN_POINT ( 'NONE',  ( 151.3999999999999773, -3543.329032635400836, 2240.279999999999745 ) ) ;
#1971=DIRECTION ( 'NONE',  ( 0.000000000000000000, 0.000000000000000000, 1.000000000000000000 ) ) ;
#1973=ORIENTED_EDGE ( 'NONE', *, *, #16267, .T. ) ;
#1976=VECTOR ( 'NONE', #8637, 1000.000000000000000 ) ;
#1977=CARTESIAN_POINT ( 'NONE',  ( 101.5999999999999943, -3568.700000000000273, 2239.771999999999935 ) ) ;
#1984=DIRECTION ( 'NONE',  ( 0.000000000000000000, 0.000000000000000000, -1.000000000000000000 ) ) ;
#1985=CIRCLE ( 'NONE', #10963, 5.715000000000001634 ) ;
#1986=ORIENTED_EDGE ( 'NONE', *, *, #18297, .T. ) ;
#1987=CARTESIAN_POINT ( 'NONE',  ( 137.8755860065629975, -3581.677971386929130, 2247.791257809596118 ) ) ;
#1988=EDGE_LOOP ( 'NONE', ( #9422, #22427 ) ) ;
#1989=VECTOR ( 'NONE', #2955, 1000.000000000000000 ) ;
#1992=AXIS2_PLACEMENT_3D ( 'NONE', #21698, #2245, #18064 ) ;
#1995=CARTESIAN_POINT ( 'NONE',  ( 6.985000002048999512, -3579.494756921999851, 2244.617465693000213 ) ) ;
#1996=CYLINDRICAL_SURFACE ( 'NONE', #13744, 5.714999999999998082 ) ;
#1999=CARTESIAN_POINT ( 'NONE',  ( 141.1782708254342822, -3577.063961468278649, 2249.598379591055163 ) ) ;
#2001=CIRCLE ( 'NONE', #5370, 2.844800000000091700 ) ;
#2002=CARTESIAN_POINT ( 'NONE',  ( 135.0631415578579606, -3576.153948019764357, 2246.504844866586154 ) ) ;
#2004=ORIENTED_EDGE ( 'NONE', *, *, #11208, .T. ) ;
#2008=AXIS2_PLACEMENT_3D ( 'NONE', #13031, #20176, #4116 ) ;
#2009=EDGE_CURVE ( 'NONE', #22481, #18295, #3084, .T. ) ;
#2011=EDGE_LOOP ( 'NONE', ( #22425, #17935, #19349, #11921 ) ) ;
#2014=EDGE_LOOP ( 'NONE', ( #20946, #5388 ) ) ;
#2015=DIRECTION ( 'NONE',  ( 1.000000000000000000, 0.000000000000000000, 0.000000000000000000 ) ) ;
#2017=FACE_OUTER_BOUND ( 'NONE', #15289, .T. ) ;
#2019=AXIS2_PLACEMENT_3D ( 'NONE', #17462, #22736, #15605 ) ;
#2023=DIRECTION ( 'NONE',  ( 0.000000000000000000, 0.000000000000000000, 1.000000000000000000 ) ) ;
#2025=CARTESIAN_POINT ( 'NONE',  ( 18.26136626118261574, -3580.811168666933554, 2245.321774183003981 ) ) ;
#2026=CARTESIAN_POINT ( 'NONE',  ( 137.3727324534160914, -3657.868512552856373, 2249.105625754800258 ) ) ;
#2027=VERTEX_POINT ( 'NONE', #9473 ) ;
#2029=CARTESIAN_POINT ( 'NONE',  ( 141.5159261927328487, -3661.696737588060842, 2249.774008737822442 ) ) ;
#2030=EDGE_LOOP ( 'NONE', ( #18560, #22944, #14148, #10652, #19150, #6316, #6195, #22525 ) ) ;
#2032=CIRCLE ( 'NONE', #9864, 3.606800000000000228 ) ;
#2036=EDGE_LOOP ( 'NONE', ( #17370, #5477 ) ) ;
#2037=CARTESIAN_POINT ( 'NONE',  ( 15.44319999999931525, -3658.626742952524637, 2255.967040000000907 ) ) ;
#2040=DIRECTION ( 'NONE',  ( 0.000000000000000000, 0.000000000000000000, 1.000000000000000000 ) ) ;
#2041=ORIENTED_EDGE ( 'NONE', *, *, #6288, .F. ) ;
#2043=DIRECTION ( 'NONE',  ( 0.000000000000000000, -1.000000000000000000, 0.000000000000000000 ) ) ;
#2044=CARTESIAN_POINT ( 'NONE',  ( 7.322952892593269425, -3581.431939765986954, 2246.174326570242556 ) ) ;
#2054=ADVANCED_FACE ( 'NONE', ( #2444 ), #682, .F. ) ;
#2055=CARTESIAN_POINT ( 'NONE',  ( 28.24479999999899604, -3619.500000000000000, 2259.837999999999738 ) ) ;
#2059=CARTESIAN_POINT ( 'NONE',  ( 57.14999999999999858, -3670.300000000000182, 2247.392000000000280 ) ) ;
#2060=EDGE_CURVE ( 'NONE', #279, #16346, #14693, .T. ) ;
#2061=ADVANCED_FACE ( 'NONE', ( #13914 ), #17067, .F. ) ;
#2062=DIRECTION ( 'NONE',  ( 0.000000000000000000, 0.000000000000000000, 1.000000000000000000 ) ) ;
#2068=CARTESIAN_POINT ( 'NONE',  ( 50.79999999999999716, -3670.300000000000182, 2259.837999999999738 ) ) ;
#2070=B_SPLINE_CURVE_WITH_KNOTS ( 'NONE', 3,
 ( #10430, #6927, #8794, #17571, #1521, #6701, #8569, #8679, #22956, #15942, #14072, #11957, #15827, #19229, #23073, #14194, #17336, #13954, #12314, #21224, #4926, #5173, #7050, #21336, #11844, #19110, #18997, #3163, #2939, #20986, #10076, #17222, #1167, #8334, #10316, #15711, #22841, #6585, #12073, #3047, #15478, #10198, #13726 ),
 .UNSPECIFIED., .F., .F.,
 ( 4, 2, 2, 1, 1, 2, 2, 2, 1, 2, 2, 2, 2, 2, 2, 2, 2, 2, 2, 2, 2, 2, 4 ),
 ( 0.000000000000000000, 0.1249999999996564692, 0.1874999999994266253, 0.2187499999993604283, 0.2343749999993274824, 0.2421874999993110233, 0.2499999999992945365, 0.3124999999992997823, 0.3437499999992194577, 0.3593749999991818767, 0.3749999999991442956, 0.4374999999991522337, 0.4687499999992162381, 0.4999999999992802424, 0.5624999999995130562, 0.5937499999996295186, 0.6093749999995666800, 0.6249999999995037303, 0.6874999999994484412, 0.7187499999995694555, 0.7499999999996904698, 0.8749999999998452349, 1.000000000000000000 ),
 .UNSPECIFIED. ) ;
#2072=VECTOR ( 'NONE', #19583, 1000.000000000000000 ) ;
#2077=CARTESIAN_POINT ( 'NONE',  ( 142.2882464502881703, -3544.023782197908986, 2255.653245238742784 ) ) ;
#2078=EDGE_CURVE ( 'NONE', #2568, #6304, #10195, .T. ) ;
#2079=CARTESIAN_POINT ( 'NONE',  ( 137.1349041368046073, -3694.826579460890571, 2255.711176449251980 ) ) ;
#2080=CARTESIAN_POINT ( 'NONE',  ( 7.790018067753250897, -3576.570178142666919, 2245.703553554133578 ) ) ;
#2083=CARTESIAN_POINT ( 'NONE',  ( 127.0000000000000000, -3568.700000000000273, 2239.771999999999935 ) ) ;
#2087=CARTESIAN_POINT ( 'NONE',  ( 101.5999999999999943, -3568.700000000000273, 2239.771999999999935 ) ) ;
#2088=DIRECTION ( 'NONE',  ( -1.000000000000000000, 0.000000000000000000, 0.000000000000000000 ) ) ;
#2090=CIRCLE ( 'NONE', #17035, 0.7619999999999294005 ) ;
#2094=VERTEX_POINT ( 'NONE', #17300 ) ;
#2095=CARTESIAN_POINT ( 'NONE',  ( 22.55520000000100111, -3619.500000000000000, 2239.771999999999935 ) ) ;
#2099=CARTESIAN_POINT ( 'NONE',  ( 35.25520000000000209, -3594.099999999999909, 2239.771999999999935 ) ) ;
#2100=EDGE_CURVE ( 'NONE', #10158, #3298, #5011, .T. ) ;
#2104=ORIENTED_EDGE ( 'NONE', *, *, #896, .F. ) ;
#2105=LINE ( 'NONE', #20031, #16052 ) ;
#2107=AXIS2_PLACEMENT_3D ( 'NONE', #23144, #22913, #12497 ) ;
#2109=ORIENTED_EDGE ( 'NONE', *, *, #369, .F. ) ;
#2110=TOROIDAL_SURFACE ( 'NONE', #17803, 3.606799999998999695, 0.7620000000000000107 ) ;
#2111=CARTESIAN_POINT ( 'NONE',  ( 137.0429226604888697, -3580.511331052818605, 2249.708490802025153 ) ) ;
#2112=ORIENTED_EDGE ( 'NONE', *, *, #22032, .T. ) ;
#2115=CARTESIAN_POINT ( 'NONE',  ( 133.9850000019999925, -3579.494756921999851, 2244.617465693000213 ) ) ;
#2119=DIRECTION ( 'NONE',  ( 0.000000000000000000, 0.000000000000000000, 1.000000000000000000 ) ) ;
#2121=CARTESIAN_POINT ( 'NONE',  ( 134.4205046047358110, -3577.301034214552146, 2245.005495992568740 ) ) ;
#2126=CIRCLE ( 'NONE', #9291, 2.844800000000091700 ) ;
#2127=CARTESIAN_POINT ( 'NONE',  ( 97.99320000000000164, -3568.700000000000273, 2239.009999999999764 ) ) ;
#2129=AXIS2_PLACEMENT_3D ( 'NONE', #17400, #5234, #15666 ) ;
#2130=EDGE_LOOP ( 'NONE', ( #2406, #19171, #16491, #20611 ) ) ;
#2131=EDGE_CURVE ( 'NONE', #18714, #22886, #9455, .T. ) ;
#2135=CARTESIAN_POINT ( 'NONE',  ( 86.05520000000001346, -3644.899999999999636, 2239.771999999999935 ) ) ;
#2136=DIRECTION ( 'NONE',  ( 0.8928571428588499836, -0.4503400076008471919, 0.000000000000000000 ) ) ;
#2137=FACE_OUTER_BOUND ( 'NONE', #1043, .T. ) ;
#2139=ORIENTED_EDGE ( 'NONE', *, *, #14366, .F. ) ;
#2143=AXIS2_PLACEMENT_3D ( 'NONE', #21953, #3683, #18096 ) ;
#2145=CARTESIAN_POINT ( 'NONE',  ( 139.6999999999999886, -3579.494999999999891, 2272.030000000000200 ) ) ;
#2146=VERTEX_POINT ( 'NONE', #4884 ) ;
#2149=CARTESIAN_POINT ( 'NONE',  ( 137.9086613251612050, -3657.294972066808896, 2247.463768499330854 ) ) ;
#2154=CARTESIAN_POINT ( 'NONE',  ( 138.6914917811226644, -3662.165394498078058, 2249.389780753679133 ) ) ;
#2155=EDGE_LOOP ( 'NONE', ( #7599, #8779, #13413, #12237 ) ) ;
#2157=AXIS2_PLACEMENT_3D ( 'NONE', #14536, #3859, #17918 ) ;
#2158=EDGE_CURVE ( 'NONE', #3136, #20114, #8191, .T. ) ;
#2160=VERTEX_POINT ( 'NONE', #8290 ) ;
#2164=DIRECTION ( 'NONE',  ( 0.000000000000000000, 0.000000000000000000, 1.000000000000000000 ) ) ;
#2167=LINE ( 'NONE', #3680, #8110 ) ;
#2168=CIRCLE ( 'NONE', #21251, 0.7620000000000126672 ) ;
#2171=DIRECTION ( 'NONE',  ( 0.000000000000000000, 0.000000000000000000, 1.000000000000000000 ) ) ;
#2174=DIRECTION ( 'NONE',  ( 0.6887494619146540265, 0.000000000000000000, -0.7249994335944508483 ) ) ;
#2176=AXIS2_PLACEMENT_3D ( 'NONE', #9993, #4724, #6377 ) ;
#2180=FACE_OUTER_BOUND ( 'NONE', #14430, .T. ) ;
#2181=CIRCLE ( 'NONE', #22734, 0.7620000000000126672 ) ;
#2183=FACE_OUTER_BOUND ( 'NONE', #17695, .T. ) ;
#2185=CARTESIAN_POINT ( 'NONE',  ( 18.09330115235438186, -3657.614207040705423, 2246.082635417008532 ) ) ;
#2187=CARTESIAN_POINT ( 'NONE',  ( 147.6247279057841411, -3695.594480551547804, 2259.836851275938898 ) ) ;
#2196=CARTESIAN_POINT ( 'NONE',  ( 7.408172492505058493, -3577.337006982063031, 2244.988840501819595 ) ) ;
#2201=DIRECTION ( 'NONE',  ( 0.000000000000000000, 0.000000000000000000, -1.000000000000000000 ) ) ;
#2203=DIRECTION ( 'NONE',  ( 0.000000000000000000, 0.000000000000000000, 1.000000000000000000 ) ) ;
#2205=CARTESIAN_POINT ( 'NONE',  ( 124.1552000000010025, -3670.300000000000182, 2261.869999999999891 ) ) ;
#2208=ORIENTED_EDGE ( 'NONE', *, *, #1697, .T. ) ;
#2209=AXIS2_PLACEMENT_3D ( 'NONE', #14471, #2040, #3558 ) ;
#2211=CARTESIAN_POINT ( 'NONE',  ( 22.55520000000100111, -3670.300000000000182, 2261.869999999999891 ) ) ;
#2212=ORIENTED_EDGE ( 'NONE', *, *, #19029, .F. ) ;
#2213=DIRECTION ( 'NONE',  ( 0.000000000000000000, 1.000000000000000000, 0.000000000000000000 ) ) ;
#2217=FACE_OUTER_BOUND ( 'NONE', #11646, .T. ) ;
#2219=ORIENTED_EDGE ( 'NONE', *, *, #11782, .T. ) ;
#2221=FACE_OUTER_BOUND ( 'NONE', #7778, .T. ) ;
#2223=CARTESIAN_POINT ( 'NONE',  ( 145.2268399904062051, -3580.949329744816623, 2245.461031122561053 ) ) ;
#2224=ADVANCED_FACE ( 'NONE', ( #19421 ), #19532, .F. ) ;
#2226=EDGE_CURVE ( 'NONE', #11524, #18611, #17893, .T. ) ;
#2228=DIRECTION ( 'NONE',  ( -0.6723379328345788775, -0.7402443542991228309, 0.000000000000000000 ) ) ;
#2229=DIRECTION ( 'NONE',  ( 0.6887494619146010688, 0.000000000000000000, -0.7249994335945012525 ) ) ;
#2230=CARTESIAN_POINT ( 'NONE',  ( 97.99320000000000164, -3670.300000000000182, 2239.771999999999935 ) ) ;
#2231=DIRECTION ( 'NONE',  ( 0.000000000000000000, 1.000000000000000000, 0.000000000000000000 ) ) ;
#2232=VERTEX_POINT ( 'NONE', #16134 ) ;
#2233=CARTESIAN_POINT ( 'NONE',  ( 134.5048218173213854, -3577.113698916038629, 2245.146221591076028 ) ) ;
#2237=EDGE_CURVE ( 'NONE', #10346, #10620, #5379, .T. ) ;
#2239=( GEOMETRIC_REPRESENTATION_CONTEXT ( 3 ) GLOBAL_UNCERTAINTY_ASSIGNED_CONTEXT ( ( #16504 ) ) GLOBAL_UNIT_ASSIGNED_CONTEXT ( ( #20317, #4258, #3913 ) ) REPRESENTATION_CONTEXT ( 'NONE', 'WORKASPACE' ) );
#2240=CARTESIAN_POINT ( 'NONE',  ( 10.90494491371777208, -3657.298020409254605, 2247.542647217488138 ) ) ;
#2244=ORIENTED_EDGE ( 'NONE', *, *, #13583, .T. ) ;
#2245=DIRECTION ( 'NONE',  ( 0.000000000000000000, 0.000000000000000000, -1.000000000000000000 ) ) ;
#2246=CARTESIAN_POINT ( 'NONE',  ( 15.20315289981203932, -3578.142343932459426, 2250.145168982875020 ) ) ;
#2248=EDGE_LOOP ( 'NONE', ( #14161, #15954, #19817, #5907 ) ) ;
#2254=LINE ( 'NONE', #3891, #1201 ) ;
#2255=VERTEX_POINT ( 'NONE', #7118 ) ;
#2257=( GEOMETRIC_REPRESENTATION_CONTEXT ( 3 ) GLOBAL_UNCERTAINTY_ASSIGNED_CONTEXT ( ( #16741 ) ) GLOBAL_UNIT_ASSIGNED_CONTEXT ( ( #21126, #3419, #23094 ) ) REPRESENTATION_CONTEXT ( 'NONE', 'WORKASPACE' ) );
#2262=ORIENTED_EDGE ( 'NONE', *, *, #8594, .F. ) ;
#2263=CARTESIAN_POINT ( 'NONE',  ( 141.1384052739540209, -3661.961130177203358, 2249.578382423867879 ) ) ;
#2265=EDGE_CURVE ( 'NONE', #13234, #279, #18063, .T. ) ;
#2267=VECTOR ( 'NONE', #21768, 1000.000000000000000 ) ;
#2268=CARTESIAN_POINT ( 'NONE',  ( 9.903023377516998238, -3578.971306245000051, 2250.235372913999981 ) ) ;
#2269=EDGE_LOOP ( 'NONE', ( #2708, #12650, #18630, #10324 ) ) ;
#2271=DIRECTION ( 'NONE',  ( 0.000000000000000000, -1.000000000000000000, 0.000000000000000000 ) ) ;
#2272=CARTESIAN_POINT ( 'NONE',  ( 151.1299999999999955, -3544.570000000000164, 2259.329999999999927 ) ) ;
#2274=EDGE_CURVE ( 'NONE', #12156, #11527, #121, .T. ) ;
#2275=ORIENTED_EDGE ( 'NONE', *, *, #9441, .T. ) ;
#2276=FACE_OUTER_BOUND ( 'NONE', #6897, .T. ) ;
#2277=CARTESIAN_POINT ( 'NONE',  ( 29.00679999999900005, -3619.500000000000000, 2239.009999999999764 ) ) ;
#2281=EDGE_LOOP ( 'NONE', ( #2685, #16254, #18447, #22500 ) ) ;
#2284=CARTESIAN_POINT ( 'NONE',  ( 0.000000000000000000, -3660.140000000000327, 2243.277199999999993 ) ) ;
#2286=DIRECTION ( 'NONE',  ( -1.224646799147353207E-16, 1.000000000000000000, 0.000000000000000000 ) ) ;
#2295=CARTESIAN_POINT ( 'NONE',  ( 147.8270794805000037, -3543.299999999999727, 2259.329999999999927 ) ) ;
#2297=CARTESIAN_POINT ( 'NONE',  ( 34.49320000000000164, -3594.099999999999909, 2259.837999999999738 ) ) ;
#2302=LINE ( 'NONE', #4504, #8714 ) ;
#2311=AXIS2_PLACEMENT_3D ( 'NONE', #1538, #21240, #11971 ) ;
#2314=ORIENTED_EDGE ( 'NONE', *, *, #12075, .F. ) ;
#2318=VERTEX_POINT ( 'NONE', #7571 ) ;
#2321=CARTESIAN_POINT ( 'NONE',  ( 139.6999999999999886, -3659.504999999999654, 2239.771999999999935 ) ) ;
#2322=ORIENTED_EDGE ( 'NONE', *, *, #15440, .T. ) ;
#2326=AXIS2_PLACEMENT_3D ( 'NONE', #7377, #12647, #5514 ) ;
#2329=DIRECTION ( 'NONE',  ( 0.000000000000000000, 0.000000000000000000, -1.000000000000000000 ) ) ;
#2330=ORIENTED_EDGE ( 'NONE', *, *, #16011, .T. ) ;
#2331=CARTESIAN_POINT ( 'NONE',  ( 137.1599999999999966, -3544.570000000000164, 2255.774000000000342 ) ) ;
#2332=ORIENTED_EDGE ( 'NONE', *, *, #7003, .F. ) ;
#2335=CIRCLE ( 'NONE', #4565, 2.844799999998998796 ) ;
#2337=CARTESIAN_POINT ( 'NONE',  ( 17.89998574415049504, -3661.876074222023362, 2245.138158857901090 ) ) ;
#2338=TOROIDAL_SURFACE ( 'NONE', #9061, 4.114799999999999791, 1.270000000000000018 ) ;
#2340=DIRECTION ( 'NONE',  ( 0.000000000000000000, 0.000000000000000000, -1.000000000000000000 ) ) ;
#2343=AXIS2_PLACEMENT_3D ( 'NONE', #3245, #10157, #17412 ) ;
#2344=CARTESIAN_POINT ( 'NONE',  ( 138.8064908466931229, -3576.792948563582740, 2249.346826069327562 ) ) ;
#2345=B_SPLINE_CURVE_WITH_KNOTS ( 'NONE', 3,
 ( #6182, #16292, #19704, #131, #5405, #21455, #21799, #9033, #19930, #12661, #16940, #11138, #13320, #7163, #7934, #10903, #16179, #18277, #5761, #2121, #12894, #20052, #9382, #7275, #3987, #14547, #2233, #18051, #16826, #14312, #20470, #12547, #21683, #3869, #18161, #1880, #3745, #14426, #5642, #9151, #11017, #5532, #15082, #3634, #7395, #12775, #771, #4415, #21579, #11550, #2002, #10787 ),
 .UNSPECIFIED., .F., .F.,
 ( 4, 2, 1, 1, 1, 1, 2, 2, 2, 1, 2, 2, 2, 2, 1, 1, 1, 2, 2, 2, 2, 1, 1, 1, 2, 2, 2, 1, 1, 1, 2, 2, 4 ),
 ( 0.000000000000000000, 0.003906250000035784743, 0.007812500000071569486, 0.01562500000014313897, 0.03125000000029341807, 0.06250000000097141739, 0.1250000000023522018, 0.2500000000051094684, 0.2656250000053414495, 0.2812500000055733751, 0.3125000000065150108, 0.3750000000082734930, 0.5000000000120827792, 0.5019531250121850308, 0.5039062500122872823, 0.5078125000120770061, 0.5156250000117660326, 0.5312500000110412790, 0.5625000000099311670, 0.6250000000077041706, 0.6289062500076025852, 0.6328125000075008888, 0.6406250000076526563, 0.6562500000081283869, 0.6875000000090798480, 0.7500000000109762199, 0.7539062500107607256, 0.7578125000105452314, 0.7656250000102002851, 0.7812500000095102815, 0.8125000000080342399, 0.8750000000053581584, 1.000000000000000000 ),
 .UNSPECIFIED. ) ;
#2346=EDGE_LOOP ( 'NONE', ( #7676, #13469, #20053, #4228 ) ) ;
#2350=ORIENTED_EDGE ( 'NONE', *, *, #20870, .T. ) ;
#2351=EDGE_CURVE ( 'NONE', #22988, #6254, #18464, .T. ) ;
#2354=AXIS2_PLACEMENT_3D ( 'NONE', #1904, #21366, #3429 ) ;
#2360=ORIENTED_EDGE ( 'NONE', *, *, #9679, .T. ) ;
#2363=CARTESIAN_POINT ( 'NONE',  ( 14.01878970267436131, -3576.973962030261191, 2249.521889377991101 ) ) ;
#2364=EDGE_CURVE ( 'NONE', #6776, #6888, #10586, .T. ) ;
#2366=ORIENTED_EDGE ( 'NONE', *, *, #17387, .F. ) ;
#2372=CARTESIAN_POINT ( 'NONE',  ( 67.10679999999999268, -3644.899999999999636, 2239.771999999999935 ) ) ;
#2375=CIRCLE ( 'NONE', #18451, 3.606799999999993567 ) ;
#2378=AXIS2_PLACEMENT_3D ( 'NONE', #2392, #20318, #11291 ) ;
#2379=CARTESIAN_POINT ( 'NONE',  ( 141.6834302667064662, -3661.544945296150217, 2249.865925870181400 ) ) ;
#2380=AXIS2_PLACEMENT_3D ( 'NONE', #11967, #22619, #19118 ) ;
#2381=EDGE_LOOP ( 'NONE', ( #22434, #18228, #18853, #7550, #7622, #543, #15958, #14647, #11502, #20253 ) ) ;
#2382=EDGE_LOOP ( 'NONE', ( #3944, #2350 ) ) ;
#2386=DIRECTION ( 'NONE',  ( 1.000000000000000000, 0.000000000000000000, 0.000000000000000000 ) ) ;
#2388=CIRCLE ( 'NONE', #6907, 1.270000000000000018 ) ;
#2389=ORIENTED_EDGE ( 'NONE', *, *, #22609, .F. ) ;
#2390=CARTESIAN_POINT ( 'NONE',  ( 7.146169398868164713, -3658.157008654403398, 2245.351788695067626 ) ) ;
#2392=CARTESIAN_POINT ( 'NONE',  ( 151.1299999999999955, -3694.430000000000291, 2239.009999999999764 ) ) ;
#2393=B_SPLINE_CURVE_WITH_KNOTS ( 'NONE', 3,
 ( #2573, #6333, #9721, #7971, #15119, #13467, #2240, #20608, #11941, #17442, #6797, #20727, #13940, #15461, #4554, #19212, #8555, #11825, #8198, #22717, #3267, #5034, #22477, #15345, #17206, #22593, #18981, #2922, #15697, #17323, #6448, #10299, #18856, #1393, #2798, #22938, #10414, #6688, #4796, #13589, #19330, #1152, #12058, #9944, #22826, #12179, #19093, #3150, #1271, #3033, #21088 ),
 .UNSPECIFIED., .F., .F.,
 ( 4, 2, 2, 2, 2, 1, 2, 2, 2, 2, 1, 1, 1, 2, 2, 2, 2, 2, 2, 1, 1, 2, 2, 2, 2, 1, 2, 2, 4 ),
 ( 0.000000000000000000, 0.1250000000061616823, 0.1875000000094276253, 0.2500000000126935684, 0.3125000000159595670, 0.3437500000176187398, 0.3593750000186234361, 0.3750000000196281325, 0.4375000000244468890, 0.4687500000268562395, 0.4843750000280609425, 0.4921875000287578295, 0.4960937500291060509, 0.4980468750292800784, 0.5000000000294539948, 0.5312500000300575120, 0.5625000000306610293, 0.5937500000312645465, 0.6093750000316296989, 0.6171875000318279847, 0.6210937500318399751, 0.6230468750317533777, 0.6250000000316668913, 0.6875000000274392731, 0.7187500000253340682, 0.7343750000242814657, 0.7421875000237551090, 0.7500000000232288633, 1.000000000000000000 ),
 .UNSPECIFIED. ) ;
#2394=CARTESIAN_POINT ( 'NONE',  ( 116.8400000000000034, -3670.300000000000182, 2247.392000000000280 ) ) ;
#2397=CARTESIAN_POINT ( 'NONE',  ( 142.3526667532784415, -3658.477248352761308, 2249.700313726392324 ) ) ;
#2398=CARTESIAN_POINT ( 'NONE',  ( 7.775933288980430014, -3662.408063519517327, 2245.667439000669219 ) ) ;
#2401=DIRECTION ( 'NONE',  ( 0.000000000000000000, -1.000000000000000000, 0.000000000000000000 ) ) ;
#2402=DIRECTION ( 'NONE',  ( 0.000000000000000000, -1.000000000000000000, 0.000000000000000000 ) ) ;
#2405=CARTESIAN_POINT ( 'NONE',  ( 18.25858294719762043, -3658.177107789667843, 2245.332874465672376 ) ) ;
#2406=ORIENTED_EDGE ( 'NONE', *, *, #17721, .F. ) ;
#2408=CARTESIAN_POINT ( 'NONE',  ( 139.6999999999999886, -3579.494999999999891, 2246.630000000000109 ) ) ;
#2410=ADVANCED_FACE ( 'NONE', ( #9339 ), #12086, .T. ) ;
#2411=EDGE_CURVE ( 'NONE', #9808, #10881, #7979, .T. ) ;
#2417=CIRCLE ( 'NONE', #15504, 0.7619999999999294005 ) ;
#2418=CARTESIAN_POINT ( 'NONE',  ( 7.619002919287616749, -3576.878850740295547, 2245.350237844942058 ) ) ;
#2419=ORIENTED_EDGE ( 'NONE', *, *, #18994, .F. ) ;
#2421=AXIS2_PLACEMENT_3D ( 'NONE', #14663, #11021, #9610 ) ;
#2425=CARTESIAN_POINT ( 'NONE',  ( 9.856504185002760821, -3579.622864616615061, 2250.134322108942342 ) ) ;
#2429=DIRECTION ( 'NONE',  ( 0.000000000000000000, 0.000000000000000000, 1.000000000000000000 ) ) ;
#2432=CARTESIAN_POINT ( 'NONE',  ( 38.10000000000000142, -3644.899999999999636, 2259.837999999999738 ) ) ;
#2433=EDGE_LOOP ( 'NONE', ( #10818, #7057 ) ) ;
#2435=CARTESIAN_POINT ( 'NONE',  ( 13.69877355052640056, -3662.169030373610894, 2249.386253497014877 ) ) ;
#2438=VECTOR ( 'NONE', #9310, 1000.000000000000000 ) ;
#2439=EDGE_LOOP ( 'NONE', ( #10885, #22374, #15745, #935, #2314, #21837, #11328, #19676, #5055, #7825, #11231, #11730 ) ) ;
#2440=DIRECTION ( 'NONE',  ( 0.000000000000000000, 1.000000000000000000, 0.000000000000000000 ) ) ;
#2444=FACE_OUTER_BOUND ( 'NONE', #14061, .T. ) ;
#2450=ORIENTED_EDGE ( 'NONE', *, *, #17383, .F. ) ;
#2452=VECTOR ( 'NONE', #4908, 1000.000000000000000 ) ;
#2454=AXIS2_PLACEMENT_3D ( 'NONE', #13206, #15090, #18600 ) ;
#2457=CARTESIAN_POINT ( 'NONE',  ( 18.05792386179019360, -3661.493495574527515, 2244.888583955523700 ) ) ;
#2458=AXIS2_PLACEMENT_3D ( 'NONE', #1173, #2704, #20409 ) ;
#2459=CARTESIAN_POINT ( 'NONE',  ( 131.9679797520999784, -3544.321224513000288, 2260.577432830999896 ) ) ;
#2460=LINE ( 'NONE', #14994, #12098 ) ;
#2461=CARTESIAN_POINT ( 'NONE',  ( 137.6667760428054805, -3577.504318391805100, 2249.893487662036478 ) ) ;
#2464=DIRECTION ( 'NONE',  ( 0.000000000000000000, 0.000000000000000000, 1.000000000000000000 ) ) ;
#2465=EDGE_LOOP ( 'NONE', ( #17999, #15347 ) ) ;
#2467=CARTESIAN_POINT ( 'NONE',  ( 123.3932000000010021, -3619.500000000000000, 2259.837999999999738 ) ) ;
#2470=AXIS2_PLACEMENT_3D ( 'NONE', #12635, #21543, #14394 ) ;
#2477=CARTESIAN_POINT ( 'NONE',  ( 20.34169023495000062, -3694.797466901999996, 2260.545675974999995 ) ) ;
#2478=CARTESIAN_POINT ( 'NONE',  ( 14.85554178696724925, -3577.638356783953441, 2249.961210317602308 ) ) ;
#2480=CARTESIAN_POINT ( 'NONE',  ( 142.3168752137765409, -3580.610805610244370, 2249.634253063868982 ) ) ;
#2481=ORIENTED_EDGE ( 'NONE', *, *, #5577, .T. ) ;
#2483=EDGE_CURVE ( 'NONE', #3518, #4940, #6607, .T. ) ;
#2485=ORIENTED_EDGE ( 'NONE', *, *, #7515, .T. ) ;
#2486=DIRECTION ( 'NONE',  ( 0.000000000000000000, -1.000000000000000000, 0.000000000000000000 ) ) ;
#2487=ADVANCED_FACE ( 'NONE', ( #11976, #19128, #12093, #13975, #5191 ), #13747, .T. ) ;
#2488=AXIS2_PLACEMENT_3D ( 'NONE', #21146, #1207, #13766 ) ;
#2495=ORIENTED_EDGE ( 'NONE', *, *, #16030, .T. ) ;
#2496=ORIENTED_EDGE ( 'NONE', *, *, #9066, .T. ) ;
#2497=CARTESIAN_POINT ( 'NONE',  ( 1.270000000000000018, -3544.570000000000164, 2240.279999999999745 ) ) ;
#2500=DIRECTION ( 'NONE',  ( 0.000000000000000000, 0.000000000000000000, -1.000000000000000000 ) ) ;
#2501=ORIENTED_EDGE ( 'NONE', *, *, #19684, .F. ) ;
#2503=CARTESIAN_POINT ( 'NONE',  ( 7.254080984692166112, -3657.771749848715444, 2245.815507489473475 ) ) ;
#2508=ADVANCED_FACE ( 'NONE', ( #21005 ), #17708, .F. ) ;
#2510=EDGE_CURVE ( 'NONE', #5555, #4126, #22550, .T. ) ;
#2512=CARTESIAN_POINT ( 'NONE',  ( 151.1299999999999955, -3660.140000000000327, 2247.392000000000280 ) ) ;
#2513=DIRECTION ( 'NONE',  ( -1.000000000000000000, 0.000000000000000000, 0.000000000000000000 ) ) ;
#2514=ORIENTED_EDGE ( 'NONE', *, *, #13583, .F. ) ;
#2516=LINE ( 'NONE', #5933, #8790 ) ;
#2524=EDGE_CURVE ( 'NONE', #9946, #13188, #6949, .T. ) ;
#2525=AXIS2_PLACEMENT_3D ( 'NONE', #10033, #773, #13550 ) ;
#2529=FACE_OUTER_BOUND ( 'NONE', #12517, .T. ) ;
#2530=DIRECTION ( 'NONE',  ( 1.000000000000000000, 0.000000000000000000, 0.000000000000000000 ) ) ;
#2531=CARTESIAN_POINT ( 'NONE',  ( 20.53778376327932520, -3695.473260056960498, 2260.054522072026884 ) ) ;
#2532=ORIENTED_EDGE ( 'NONE', *, *, #21399, .T. ) ;
#2539=ORIENTED_EDGE ( 'NONE', *, *, #402, .T. ) ;
#2540=DIRECTION ( 'NONE',  ( 0.000000000000000000, 0.000000000000000000, -1.000000000000000000 ) ) ;
#2542=EDGE_CURVE ( 'NONE', #1923, #9353, #2710, .T. ) ;
#2545=CARTESIAN_POINT ( 'NONE',  ( 1.270000000000000018, -3695.699999999999818, 2240.279999999999745 ) ) ;
#2548=ORIENTED_EDGE ( 'NONE', *, *, #17718, .F. ) ;
#2549=EDGE_CURVE ( 'NONE', #7810, #20367, #4529, .T. ) ;
#2551=CARTESIAN_POINT ( 'NONE',  ( 85.29320000000001301, -3644.899999999999636, 2260.600000000000364 ) ) ;
#2552=DIRECTION ( 'NONE',  ( -1.000000000000000000, 0.000000000000000000, 0.000000000000000000 ) ) ;
#2553=CARTESIAN_POINT ( 'NONE',  ( 144.3113860273000171, -3576.119152860999748, 2246.630000000000109 ) ) ;
#2559=CARTESIAN_POINT ( 'NONE',  ( 145.2825357078243940, -3580.718563226084370, 2245.237727082246693 ) ) ;
#2562=CARTESIAN_POINT ( 'NONE',  ( 17.74539221806004363, -3662.189252963443778, 2245.418801174103464 ) ) ;
#2563=TOROIDAL_SURFACE ( 'NONE', #14556, 3.606799999998999695, 0.7620000000000000107 ) ;
#2564=CARTESIAN_POINT ( 'NONE',  ( 127.0000000000000000, -3568.700000000000273, 2259.837999999999738 ) ) ;
#2566=EDGE_CURVE ( 'NONE', #22942, #9004, #5736, .T. ) ;
#2567=CARTESIAN_POINT ( 'NONE',  ( 137.1051927857304236, -3578.289462873045977, 2250.192425027783884 ) ) ;
#2568=VERTEX_POINT ( 'NONE', #17833 ) ;
#2571=ORIENTED_EDGE ( 'NONE', *, *, #20905, .T. ) ;
#2573=CARTESIAN_POINT ( 'NONE',  ( 10.78733304872000076, -3657.399152860999493, 2246.630000000000109 ) ) ;
#2576=ORIENTED_EDGE ( 'NONE', *, *, #18385, .T. ) ;
#2577=CARTESIAN_POINT ( 'NONE',  ( 18.01287425286000143, -3581.600847139000052, 2246.630000000000109 ) ) ;
#2580=ORIENTED_EDGE ( 'NONE', *, *, #5073, .T. ) ;
#2582=CARTESIAN_POINT ( 'NONE',  ( 13.82650316938843282, -3576.881401190747965, 2249.436478869484290 ) ) ;
#2584=CARTESIAN_POINT ( 'NONE',  ( 142.0561911310684877, -3581.089035798021541, 2249.159696853207151 ) ) ;
#2586=DIRECTION ( 'NONE',  ( 0.000000000000000000, 0.000000000000000000, -1.000000000000000000 ) ) ;
#2590=DIRECTION ( 'NONE',  ( -1.224646799147353207E-16, 1.000000000000000000, 0.000000000000000000 ) ) ;
#2591=CIRCLE ( 'NONE', #12333, 1.269999999999882334 ) ;
#2592=CARTESIAN_POINT ( 'NONE',  ( 142.5448000000000093, -3579.494999999999891, 2256.063560000000052 ) ) ;
#2594=AXIS2_PLACEMENT_3D ( 'NONE', #21867, #5943, #656 ) ;
#2599=DIRECTION ( 'NONE',  ( 0.000000000000000000, 0.000000000000000000, -1.000000000000000000 ) ) ;
#2600=ORIENTED_EDGE ( 'NONE', *, *, #17520, .T. ) ;
#2601=LINE ( 'NONE', #20311, #10161 ) ;
#2603=CIRCLE ( 'NONE', #20214, 3.606800000000000228 ) ;
#2605=CARTESIAN_POINT ( 'NONE',  ( 7.133249611714339800, -3658.211785038479775, 2245.300344505144039 ) ) ;
#2606=CARTESIAN_POINT ( 'NONE',  ( 0.000000000000000000, 0.000000000000000000, 0.000000000000000000 ) ) ;
#2612=CARTESIAN_POINT ( 'NONE',  ( 85.29320000000001301, -3594.099999999999909, 2239.771999999999935 ) ) ;
#2613=DIRECTION ( 'NONE',  ( 0.000000000000000000, 0.000000000000000000, -1.000000000000000000 ) ) ;
#2614=DIRECTION ( 'NONE',  ( 0.000000000000000000, 0.000000000000000000, -1.000000000000000000 ) ) ;
#2616=VERTEX_POINT ( 'NONE', #10450 ) ;
#2617=DIRECTION ( 'NONE',  ( 1.000000000000000000, 0.000000000000000000, 0.000000000000000000 ) ) ;
#2625=ORIENTED_EDGE ( 'NONE', *, *, #17236, .F. ) ;
#2626=ORIENTED_EDGE ( 'NONE', *, *, #10002, .T. ) ;
#2629=CARTESIAN_POINT ( 'NONE',  ( 20.17309679555000201, -3694.556024844999683, 2260.454626673999883 ) ) ;
#2634=DIRECTION ( 'NONE',  ( -1.000000000000000000, 0.000000000000000000, 0.000000000000000000 ) ) ;
#2638=DIRECTION ( 'NONE',  ( 0.000000000000000000, 1.000000000000000000, 0.000000000000000000 ) ) ;
#2646=FACE_BOUND ( 'NONE', #5108, .T. ) ;
#2647=AXIS2_PLACEMENT_3D ( 'NONE', #6740, #13880, #1447 ) ;
#2650=ORIENTED_EDGE ( 'NONE', *, *, #501, .F. ) ;
#2651=DIRECTION ( 'NONE',  ( -1.000000000000000000, 0.000000000000000000, 0.000000000000000000 ) ) ;
#2657=DIRECTION ( 'NONE',  ( 0.000000000000000000, 0.000000000000000000, -1.000000000000000000 ) ) ;
#2659=EDGE_LOOP ( 'NONE', ( #15616, #9569, #19849, #1405 ) ) ;
#2666=ORIENTED_EDGE ( 'NONE', *, *, #18028, .F. ) ;
#2667=CARTESIAN_POINT ( 'NONE',  ( 145.1235917977560632, -3581.296656515026825, 2245.923799407241859 ) ) ;
#2669=CARTESIAN_POINT ( 'NONE',  ( 38.10000000000000142, -3594.099999999999909, 2259.837999999999738 ) ) ;
#2674=ORIENTED_EDGE ( 'NONE', *, *, #9713, .F. ) ;
#2678=VECTOR ( 'NONE', #4917, 1000.000000000000000 ) ;
#2679=DIRECTION ( 'NONE',  ( 1.000000000000000000, -0.000000000000000000, 1.224646799147353207E-16 ) ) ;
#2680=VERTEX_POINT ( 'NONE', #10799 ) ;
#2681=DIRECTION ( 'NONE',  ( -1.000000000000000000, 0.000000000000000000, 0.000000000000000000 ) ) ;
#2685=ORIENTED_EDGE ( 'NONE', *, *, #5585, .F. ) ;
#2688=CIRCLE ( 'NONE', #97, 2.844800000000001550 ) ;
#2692=CARTESIAN_POINT ( 'NONE',  ( 11.02948398983750167, -3577.192243618181237, 2249.696728442258973 ) ) ;
#2693=CARTESIAN_POINT ( 'NONE',  ( 142.3664352233508623, -3580.490377153994359, 2249.725648386253852 ) ) ;
#2696=AXIS2_PLACEMENT_3D ( 'NONE', #2145, #13037, #22462 ) ;
#2699=AXIS2_PLACEMENT_3D ( 'NONE', #9696, #7717, #16837 ) ;
#2701=CARTESIAN_POINT ( 'NONE',  ( 20.37014473018363958, -3543.966768725831571, 2260.474410600547344 ) ) ;
#2704=DIRECTION ( 'NONE',  ( 1.000000000000000000, 0.000000000000000000, 0.000000000000000000 ) ) ;
#2705=ADVANCED_FACE ( 'NONE', ( #10914 ), #11258, .F. ) ;
#2706=ADVANCED_FACE ( 'NONE', ( #9395 ), #12462, .T. ) ;
#2707=ORIENTED_EDGE ( 'NONE', *, *, #2226, .F. ) ;
#2708=ORIENTED_EDGE ( 'NONE', *, *, #5511, .F. ) ;
#2709=AXIS2_PLACEMENT_3D ( 'NONE', #15787, #7686, #11203 ) ;
#2710=CIRCLE ( 'NONE', #15824, 5.714999999999950120 ) ;
#2712=VERTEX_POINT ( 'NONE', #2135 ) ;
#2715=ORIENTED_EDGE ( 'NONE', *, *, #1401, .F. ) ;
#2716=CIRCLE ( 'NONE', #6482, 3.606799999999993567 ) ;
#2717=CARTESIAN_POINT ( 'NONE',  ( 7.026240522554910051, -3658.819843006041538, 2244.872055837873631 ) ) ;
#2720=CIRCLE ( 'NONE', #6125, 1.269999999999882334 ) ;
#2722=LINE ( 'NONE', #12103, #22508 ) ;
#2723=DIRECTION ( 'NONE',  ( 1.000000000000000000, 0.000000000000000000, 0.000000000000000000 ) ) ;
#2724=B_SPLINE_CURVE_WITH_KNOTS ( 'NONE', 3,
 ( #13679, #6423, #6543, #13562, #2774, #5889, #20171, #9917, #8060, #13442, #20582, #20701, #19189, #6892, #16020, #21300, #19420, #17770, #7117, #12152, #10393, #1726, #14034, #10624, #20944, #8531, #21186, #5243, #19306, #12035, #5361, #3472, #12500, #14157, #23037, #5010, #15907, #14267, #7012, #12384, #3356, #5131, #19531, #10507, #22916, #8876, #17532, #23146, #12274, #19650, #17892, #21412, #17648, #3591, #10274, #10746, #1598, #3124, #8759, #1838, #8984, #22691, #6663, #13800 ),
 .UNSPECIFIED., .F., .F.,
 ( 4, 2, 1, 1, 2, 2, 2, 2, 1, 2, 2, 2, 2, 1, 1, 2, 2, 2, 2, 1, 2, 2, 2, 2, 1, 2, 2, 2, 2, 2, 2, 2, 1, 2, 2, 4 ),
 ( 0.001021189648326963767, 0.06345736529341350352, 0.09467545311595677859, 0.1102844970271577435, 0.1180890189827582121, 0.1258935409383586945, 0.1883297165821066210, 0.2195478044041626053, 0.2351568483152942923, 0.2429613702709592371, 0.2507658922266241541, 0.3132020678728795748, 0.3444201556960073685, 0.3600291996077152334, 0.3678337215635693047, 0.3717359825415584296, 0.3756382435195474989, 0.4068563313439385043, 0.4224653752561136066, 0.4302698972122011578, 0.4341721581902011073, 0.4380744191682010014, 0.4692925069923846726, 0.4849015509043257399, 0.4927060728601833084, 0.4966083338381755974, 0.5005105948161677754, 0.5629467704654305127, 0.5941648582901043474, 0.6097739022023097588, 0.6253829461145151702, 0.6878191217629900933, 0.7190372095870988245, 0.7346462534990108040, 0.7502552974109228945, 1.000000000000000000 ),
 .UNSPECIFIED. ) ;
#2725=AXIS2_PLACEMENT_3D ( 'NONE', #8586, #12095, #8474 ) ;
#2726=CIRCLE ( 'NONE', #10229, 2.844799999999994444 ) ;
#2729=EDGE_LOOP ( 'NONE', ( #18788, #2576 ) ) ;
#2733=CIRCLE ( 'NONE', #2019, 2.844800000000091700 ) ;
#2734=CARTESIAN_POINT ( 'NONE',  ( 136.8551999999999964, -3659.504999999999654, 2256.063560000000052 ) ) ;
#2736=TOROIDAL_SURFACE ( 'NONE', #5762, 3.606799999999999784, 0.7620000000000000107 ) ;
#2737=ORIENTED_EDGE ( 'NONE', *, *, #4275, .T. ) ;
#2738=ORIENTED_EDGE ( 'NONE', *, *, #6251, .T. ) ;
#2744=DIRECTION ( 'NONE',  ( 0.000000000000000000, 0.000000000000000000, -1.000000000000000000 ) ) ;
#2752=AXIS2_PLACEMENT_3D ( 'NONE', #20959, #7134, #1262 ) ;
#2753=AXIS2_PLACEMENT_3D ( 'NONE', #7655, #2171, #11061 ) ;
#2754=CARTESIAN_POINT ( 'NONE',  ( 9.901643740141382821, -3580.009520309946765, 2249.994425513007627 ) ) ;
#2755=ADVANCED_FACE ( 'NONE', ( #12905 ), #18177, .T. ) ;
#2757=ADVANCED_FACE ( 'NONE', ( #3882 ), #372, .T. ) ;
#2762=CARTESIAN_POINT ( 'NONE',  ( 144.9135508633802942, -3661.845961013772467, 2245.115470801160882 ) ) ;
#2765=CARTESIAN_POINT ( 'NONE',  ( 14.37045735331549956, -3661.808175004912755, 2249.696654784097973 ) ) ;
#2767=ORIENTED_EDGE ( 'NONE', *, *, #5212, .T. ) ;
#2770=VECTOR ( 'NONE', #7819, 1000.000000000000000 ) ;
#2774=CARTESIAN_POINT ( 'NONE',  ( 15.51466946139100145, -3659.084409417217103, 2250.034617945921127 ) ) ;
#2775=DIRECTION ( 'NONE',  ( 0.000000000000000000, 0.000000000000000000, -1.000000000000000000 ) ) ;
#2783=CARTESIAN_POINT ( 'NONE',  ( 127.0000000000000000, -3670.300000000000182, 2261.869999999999891 ) ) ;
#2784=DIRECTION ( 'NONE',  ( -1.000000000000000000, 0.000000000000000000, 0.000000000000000000 ) ) ;
#2785=CARTESIAN_POINT ( 'NONE',  ( 17.73948428411033973, -3662.200341972358729, 2245.430382740787081 ) ) ;
#2786=AXIS2_PLACEMENT_3D ( 'NONE', #16461, #21743, #21516 ) ;
#2790=DIRECTION ( 'NONE',  ( 0.000000000000000000, 1.000000000000000000, 0.000000000000000000 ) ) ;
#2791=CIRCLE ( 'NONE', #1287, 5.714999999999927915 ) ;
#2795=CARTESIAN_POINT ( 'NONE',  ( 142.7470794804999912, -3543.299999999999727, 2254.503999999999905 ) ) ;
#2798=CARTESIAN_POINT ( 'NONE',  ( 10.30318750565348829, -3657.972703622658173, 2249.234803022183314 ) ) ;
#2800=VERTEX_POINT ( 'NONE', #2477 ) ;
#2801=ORIENTED_EDGE ( 'NONE', *, *, #14955, .F. ) ;
#2808=DIRECTION ( 'NONE',  ( 0.000000000000000000, 0.000000000000000000, -1.000000000000000000 ) ) ;
#2812=CARTESIAN_POINT ( 'NONE',  ( 141.6290972793774188, -3581.586076845646858, 2248.209447196302335 ) ) ;
#2816=CARTESIAN_POINT ( 'NONE',  ( 10.16000000000000014, -3578.213872745999652, 2255.774000000000342 ) ) ;
#2818=CARTESIAN_POINT ( 'NONE',  ( 133.9885211612832734, -3659.275430740734464, 2244.678943280418480 ) ) ;
#2819=AXIS2_PLACEMENT_3D ( 'NONE', #16498, #12992, #12554 ) ;
#2821=CIRCLE ( 'NONE', #22638, 4.114799999999974034 ) ;
#2825=AXIS2_PLACEMENT_3D ( 'NONE', #12406, #8659, #10640 ) ;
#2827=ADVANCED_FACE ( 'NONE', ( #7980 ), #2852, .T. ) ;
#2830=ORIENTED_EDGE ( 'NONE', *, *, #548, .F. ) ;
#2832=DIRECTION ( 'NONE',  ( -0.7249994335945011414, 0.000000000000000000, -0.6887494619146010688 ) ) ;
#2833=DIRECTION ( 'NONE',  ( 0.000000000000000000, 0.000000000000000000, 1.000000000000000000 ) ) ;
#2834=EDGE_CURVE ( 'NONE', #140, #21948, #18610, .T. ) ;
#2836=CARTESIAN_POINT ( 'NONE',  ( 7.266527782489568210, -3657.733286618344209, 2245.875159459704719 ) ) ;
#2841=EDGE_CURVE ( 'NONE', #20865, #830, #7753, .T. ) ;
#2850=CARTESIAN_POINT ( 'NONE',  ( 35.56000000000000227, -3543.300000000000182, 2251.506800000000112 ) ) ;
#2852=TOROIDAL_SURFACE ( 'NONE', #14516, 3.606799999999999784, 0.7620000000000000107 ) ;
#2853=AXIS2_PLACEMENT_3D ( 'NONE', #12374, #3461, #10614 ) ;
#2855=DIRECTION ( 'NONE',  ( 0.000000000000000000, -1.000000000000000000, 0.000000000000000000 ) ) ;
#2861=CARTESIAN_POINT ( 'NONE',  ( 18.37161333721848777, -3658.802287535873802, 2244.881330935113056 ) ) ;
#2862=VERTEX_POINT ( 'NONE', #11368 ) ;
#2867=CIRCLE ( 'NONE', #5500, 6.477000000000010971 ) ;
#2870=AXIS2_PLACEMENT_3D ( 'NONE', #12266, #19523, #5350 ) ;
#2871=CARTESIAN_POINT ( 'NONE',  ( 9.855099624826999971, -3659.505002774999411, 2250.165042250000170 ) ) ;
#2872=DIRECTION ( 'NONE',  ( 0.000000000000000000, 0.000000000000000000, -1.000000000000000000 ) ) ;
#2873=FACE_OUTER_BOUND ( 'NONE', #3318, .T. ) ;
#2874=CARTESIAN_POINT ( 'NONE',  ( 20.66917619022257924, -3695.636872341213348, 2259.725418502411685 ) ) ;
#2875=ORIENTED_EDGE ( 'NONE', *, *, #2901, .T. ) ;
#2878=EDGE_LOOP ( 'NONE', ( #12663, #21022, #8564, #17436 ) ) ;
#2881=CARTESIAN_POINT ( 'NONE',  ( 10.84819624241226421, -3581.654767633020128, 2247.929782366414656 ) ) ;
#2882=CIRCLE ( 'NONE', #5898, 0.7619999999999294005 ) ;
#2885=CARTESIAN_POINT ( 'NONE',  ( 95.25000000000000000, -3544.570000000000164, 2250.236800000000130 ) ) ;
#2886=LINE ( 'NONE', #10030, #1284 ) ;
#2887=CARTESIAN_POINT ( 'NONE',  ( 145.3776872988880768, -3660.157359719874876, 2244.547249493355139 ) ) ;
#2889=DIRECTION ( 'NONE',  ( -1.224646799147353207E-16, 1.000000000000000000, 0.000000000000000000 ) ) ;
#2892=EDGE_LOOP ( 'NONE', ( #8692, #7310, #275, #505 ) ) ;
#2895=VECTOR ( 'NONE', #22037, 1000.000000000000000 ) ;
#2901=EDGE_CURVE ( 'NONE', #21361, #2318, #971, .T. ) ;
#2902=VECTOR ( 'NONE', #19901, 1000.000000000000000 ) ;
#2906=CARTESIAN_POINT ( 'NONE',  ( 9.851243568427076269, -3543.401189131950559, 2255.000779105281708 ) ) ;
#2908=CARTESIAN_POINT ( 'NONE',  ( 9.916854418464000176, -3578.905956564000007, 2250.236428761999832 ) ) ;
#2911=DIRECTION ( 'NONE',  ( 0.000000000000000000, 0.000000000000000000, -1.000000000000000000 ) ) ;
#2912=CARTESIAN_POINT ( 'NONE',  ( 127.0000000000000000, -3670.300000000000182, 2259.837999999999738 ) ) ;
#2914=CARTESIAN_POINT ( 'NONE',  ( 137.4507161353425886, -3577.751214325344790, 2250.012832018660902 ) ) ;
#2915=VERTEX_POINT ( 'NONE', #20505 ) ;
#2916=CARTESIAN_POINT ( 'NONE',  ( 28.24479999999899604, -3568.700000000000273, 2239.771999999999935 ) ) ;
#2920=EDGE_LOOP ( 'NONE', ( #23069, #22694, #15755, #16947 ) ) ;
#2921=LINE ( 'NONE', #9943, #15921 ) ;
#2922=CARTESIAN_POINT ( 'NONE',  ( 10.49306405180820612, -3657.709384941907501, 2248.871247615949414 ) ) ;
#2926=CARTESIAN_POINT ( 'NONE',  ( 134.3066495004684668, -3581.385628414011080, 2246.082317947095362 ) ) ;
#2930=CIRCLE ( 'NONE', #5183, 1.269999999999882334 ) ;
#2932=DIRECTION ( 'NONE',  ( 0.000000000000000000, 1.000000000000000000, 0.000000000000000000 ) ) ;
#2934=CARTESIAN_POINT ( 'NONE',  ( 142.2663395169348064, -3580.722924689276624, 2249.542540277683202 ) ) ;
#2935=EDGE_LOOP ( 'NONE', ( #10604, #9279, #17265, #22529 ) ) ;
#2939=CARTESIAN_POINT ( 'NONE',  ( 14.64973061487417816, -3581.566609002860787, 2248.268300351840935 ) ) ;
#2940=PLANE ( 'NONE',  #846 ) ;
#2941=EDGE_CURVE ( 'NONE', #17865, #12626, #11591, .T. ) ;
#2942=ORIENTED_EDGE ( 'NONE', *, *, #21990, .F. ) ;
#2946=TOROIDAL_SURFACE ( 'NONE', #2209, 3.606799999998999695, 0.7620000000000000107 ) ;
#2947=DIRECTION ( 'NONE',  ( 0.000000000000000000, 0.000000000000000000, 1.000000000000000000 ) ) ;
#2954=CARTESIAN_POINT ( 'NONE',  ( 15.49256139849371117, -3660.048737986045126, 2250.235547086222141 ) ) ;
#2955=DIRECTION ( 'NONE',  ( 0.000000000000000000, 0.000000000000000000, -1.000000000000000000 ) ) ;
#2958=EDGE_CURVE ( 'NONE', #17137, #13472, #9222, .T. ) ;
#2960=CYLINDRICAL_SURFACE ( 'NONE', #18180, 1.269999999999882334 ) ;
#2961=DIRECTION ( 'NONE',  ( -1.000000000000000000, 0.000000000000000000, 0.000000000000000000 ) ) ;
#2964=LINE ( 'NONE', #20776, #12455 ) ;
#2965=EDGE_CURVE ( 'NONE', #10895, #22243, #13326, .T. ) ;
#2966=VERTEX_POINT ( 'NONE', #6575 ) ;
#2967=CARTESIAN_POINT ( 'NONE',  ( 137.1293827860164640, -3544.133557167025174, 2255.697297437880934 ) ) ;
#2970=CARTESIAN_POINT ( 'NONE',  ( 4.657535968477718669, -3695.684982101911828, 2259.542693485130258 ) ) ;
#2973=ORIENTED_EDGE ( 'NONE', *, *, #13090, .F. ) ;
#2976=DIRECTION ( 'NONE',  ( 0.000000000000000000, 0.000000000000000000, 1.000000000000000000 ) ) ;
#2977=AXIS2_PLACEMENT_3D ( 'NONE', #8380, #12121, #15522 ) ;
#2978=DIRECTION ( 'NONE',  ( 0.000000000000000000, 1.000000000000000000, 0.000000000000000000 ) ) ;
#2979=EDGE_LOOP ( 'NONE', ( #21611, #7007, #21369, #11499 ) ) ;
#2981=CARTESIAN_POINT ( 'NONE',  ( 124.1552000000010025, -3670.300000000000182, 2239.771999999999935 ) ) ;
#2983=DIRECTION ( 'NONE',  ( 0.000000000000000000, 0.000000000000000000, 1.000000000000000000 ) ) ;
#2984=CARTESIAN_POINT ( 'NONE',  ( 20.52304216182480445, -3695.446428763979839, 2260.091482594895751 ) ) ;
#2988=ORIENTED_EDGE ( 'NONE', *, *, #7501, .T. ) ;
#2991=CARTESIAN_POINT ( 'NONE',  ( 10.78723565514999905, -3581.600816721000228, 2246.630000000000109 ) ) ;
#2995=ORIENTED_EDGE ( 'NONE', *, *, #13453, .T. ) ;
#2998=CARTESIAN_POINT ( 'NONE',  ( 145.3283279854914554, -3660.498787106118925, 2244.568960851285283 ) ) ;
#2999=PLANE ( 'NONE',  #14483 ) ;
#3001=CARTESIAN_POINT ( 'NONE',  ( 10.97468688268398651, -3661.767038422824953, 2249.725556830857840 ) ) ;
#3003=CARTESIAN_POINT ( 'NONE',  ( 147.4094809636181651, -3543.848287272899142, 2260.375776696899720 ) ) ;
#3006=CARTESIAN_POINT ( 'NONE',  ( 47.19319999999999737, -3619.500000000000000, 2260.600000000000364 ) ) ;
#3009=DIRECTION ( 'NONE',  ( -1.000000000000000000, 0.000000000000000000, 0.000000000000000000 ) ) ;
#3014=DIRECTION ( 'NONE',  ( -0.000000000000000000, -1.000000000000000000, -0.000000000000000000 ) ) ;
#3020=EDGE_LOOP ( 'NONE', ( #13992, #2580, #9940, #621 ) ) ;
#3021=CARTESIAN_POINT ( 'NONE',  ( 142.5447999999989861, -3579.494999999999891, 2272.030000000000200 ) ) ;
#3022=CARTESIAN_POINT ( 'NONE',  ( 40.94480000000000075, -3644.899999999999636, 2259.837999999999738 ) ) ;
#3023=LINE ( 'NONE', #22707, #5139 ) ;
#3024=FACE_OUTER_BOUND ( 'NONE', #2030, .T. ) ;
#3026=DIRECTION ( 'NONE',  ( 0.000000000000000000, 0.000000000000000000, -1.000000000000000000 ) ) ;
#3029=CARTESIAN_POINT ( 'NONE',  ( 50.79999999999999716, -3568.700000000000273, 2261.869999999999891 ) ) ;
#3032=CARTESIAN_POINT ( 'NONE',  ( 10.16000000000000014, -3660.786127253999894, 2255.774000000000342 ) ) ;
#3033=CARTESIAN_POINT ( 'NONE',  ( 9.855099624826999971, -3659.161788968266592, 2250.086432307065934 ) ) ;
#3034=CIRCLE ( 'NONE', #1921, 0.7619999999999987894 ) ;
#3035=EDGE_LOOP ( 'NONE', ( #18348, #22438 ) ) ;
#3037=VERTEX_POINT ( 'NONE', #19221 ) ;
#3038=ORIENTED_EDGE ( 'NONE', *, *, #434, .F. ) ;
#3042=ORIENTED_EDGE ( 'NONE', *, *, #18959, .F. ) ;
#3046=DIRECTION ( 'NONE',  ( 0.000000000000000000, 0.000000000000000000, -1.000000000000000000 ) ) ;
#3047=CARTESIAN_POINT ( 'NONE',  ( 14.48738767196504362, -3581.708301318878966, 2247.301656039307090 ) ) ;
#3049=DIRECTION ( 'NONE',  ( -1.224646799147353207E-16, 1.000000000000000000, 0.000000000000000000 ) ) ;
#3050=AXIS2_PLACEMENT_3D ( 'NONE', #10447, #5188, #19358 ) ;
#3053=ORIENTED_EDGE ( 'NONE', *, *, #1334, .T. ) ;
#3054=CARTESIAN_POINT ( 'NONE',  ( 15.70174596903387076, -3695.700000000000273, 2254.617539517497789 ) ) ;
#3055=EDGE_CURVE ( 'NONE', #19192, #9415, #12206, .T. ) ;
#3060=ORIENTED_EDGE ( 'NONE', *, *, #2941, .F. ) ;
#3065=EDGE_LOOP ( 'NONE', ( #19908, #11118 ) ) ;
#3070=EDGE_CURVE ( 'NONE', #7277, #17151, #22668, .T. ) ;
#3073=EDGE_CURVE ( 'NONE', #21998, #5163, #20977, .T. ) ;
#3078=CARTESIAN_POINT ( 'NONE',  ( 141.8201150885594757, -3657.608162431468827, 2248.689186079961019 ) ) ;
#3079=AXIS2_PLACEMENT_3D ( 'NONE', #5138, #3014, #15677 ) ;
#3082=CARTESIAN_POINT ( 'NONE',  ( 136.6986430980723242, -3543.300000000018827, 2254.618513951348632 ) ) ;
#3083=EDGE_CURVE ( 'NONE', #15707, #16281, #17060, .T. ) ;
#3084=CIRCLE ( 'NONE', #16193, 2.844799999999994444 ) ;
#3087=CARTESIAN_POINT ( 'NONE',  ( 127.0000000000000000, -3660.140000000000327, 2244.547199999999975 ) ) ;
#3088=VERTEX_POINT ( 'NONE', #22949 ) ;
#3090=CARTESIAN_POINT ( 'NONE',  ( 98.75520000000000209, -3619.500000000000000, 2261.869999999999891 ) ) ;
#3091=AXIS2_PLACEMENT_3D ( 'NONE', #19112, #20750, #15603 ) ;
#3092=CARTESIAN_POINT ( 'NONE',  ( 136.9568000000001291, -3660.383257047432380, 2255.967039999999997 ) ) ;
#3094=DIRECTION ( 'NONE',  ( 0.000000000000000000, 0.000000000000000000, 1.000000000000000000 ) ) ;
#3095=DIRECTION ( 'NONE',  ( 1.000000000000000000, 0.000000000000000000, 0.000000000000000000 ) ) ;
#3096=CARTESIAN_POINT ( 'NONE',  ( 67.10679999999999268, -3594.099999999999909, 2260.600000000000364 ) ) ;
#3098=TOROIDAL_SURFACE ( 'NONE', #11686, 3.606799999999999784, 0.7620000000000000107 ) ;
#3100=EDGE_LOOP ( 'NONE', ( #3885, #513, #22647, #2707 ) ) ;
#3102=AXIS2_PLACEMENT_3D ( 'NONE', #15731, #10573, #12445 ) ;
#3103=ORIENTED_EDGE ( 'NONE', *, *, #7244, .T. ) ;
#3104=LINE ( 'NONE', #1461, #4176 ) ;
#3105=ORIENTED_EDGE ( 'NONE', *, *, #12013, .T. ) ;
#3106=CARTESIAN_POINT ( 'NONE',  ( 10.31606189812206154, -3581.047200597019582, 2249.211077905966249 ) ) ;
#3108=VERTEX_POINT ( 'NONE', #1279 ) ;
#3110=DIRECTION ( 'NONE',  ( 0.000000000000000000, 0.000000000000000000, -1.000000000000000000 ) ) ;
#3111=DIRECTION ( 'NONE',  ( -1.000000000000000000, 0.000000000000000000, 0.000000000000000000 ) ) ;
#3112=CARTESIAN_POINT ( 'NONE',  ( 145.0370523213743184, -3661.552992845433891, 2244.917889001342246 ) ) ;
#3113=VECTOR ( 'NONE', #16563, 1000.000000000000000 ) ;
#3114=CARTESIAN_POINT ( 'NONE',  ( 132.0583097651000060, -3694.797466901999996, 2260.545675974999995 ) ) ;
#3115=CARTESIAN_POINT ( 'NONE',  ( 10.62862398006557640, -3661.455063412160598, 2249.914674052713508 ) ) ;
#3117=EDGE_CURVE ( 'NONE', #9478, #6254, #8101, .T. ) ;
#3122=CARTESIAN_POINT ( 'NONE',  ( 142.2400000000000091, -3695.699999999999818, 2255.774000000000342 ) ) ;
#3123=DIRECTION ( 'NONE',  ( 0.000000000000000000, 0.000000000000000000, -1.000000000000000000 ) ) ;
#3124=CARTESIAN_POINT ( 'NONE',  ( 14.51722411178351813, -3657.316120473550654, 2247.740791187773084 ) ) ;
#3127=EDGE_CURVE ( 'NONE', #20621, #10571, #6305, .T. ) ;
#3129=VERTEX_POINT ( 'NONE', #20356 ) ;
#3130=DIRECTION ( 'NONE',  ( 0.000000000000000000, 0.000000000000000000, -1.000000000000000000 ) ) ;
#3132=CYLINDRICAL_SURFACE ( 'NONE', #16749, 1.270000000000000018 ) ;
#3134=EDGE_CURVE ( 'NONE', #3129, #17497, #23054, .T. ) ;
#3135=DIRECTION ( 'NONE',  ( 0.000000000000000000, 0.000000000000000000, -1.000000000000000000 ) ) ;
#3136=VERTEX_POINT ( 'NONE', #22212 ) ;
#3137=EDGE_CURVE ( 'NONE', #20690, #21069, #12340, .T. ) ;
#3142=CARTESIAN_POINT ( 'NONE',  ( 116.8400000000000034, -3543.299999999999727, 2247.392000000000280 ) ) ;
#3143=VERTEX_POINT ( 'NONE', #22103 ) ;
#3144=CIRCLE ( 'NONE', #7269, 2.844800000000091700 ) ;
#3147=AXIS2_PLACEMENT_3D ( 'NONE', #16949, #2440, #14976 ) ;
#3148=EDGE_LOOP ( 'NONE', ( #16205, #11478, #10065, #4548 ) ) ;
#3150=CARTESIAN_POINT ( 'NONE',  ( 10.05102782082138901, -3658.467715238130495, 2249.693416503429489 ) ) ;
#3158=AXIS2_PLACEMENT_3D ( 'NONE', #2432, #9575, #16721 ) ;
#3160=AXIS2_PLACEMENT_3D ( 'NONE', #2467, #9387, #7744 ) ;
#3163=CARTESIAN_POINT ( 'NONE',  ( 14.67418966406092906, -3581.543406057290667, 2248.337984869423053 ) ) ;
#3164=CARTESIAN_POINT ( 'NONE',  ( 134.0156995028073652, -3658.912717518575846, 2244.825196086624601 ) ) ;
#3167=DIRECTION ( 'NONE',  ( 0.000000000000000000, 1.000000000000000000, 0.000000000000000000 ) ) ;
#3171=DIRECTION ( 'NONE',  ( 0.000000000000000000, 0.000000000000000000, -1.000000000000000000 ) ) ;
#3174=VECTOR ( 'NONE', #6796, 1000.000000000000000 ) ;
#3176=AXIS2_PLACEMENT_3D ( 'NONE', #18766, #22275, #22167 ) ;
#3177=ORIENTED_EDGE ( 'NONE', *, *, #17604, .F. ) ;
#3178=DIRECTION ( 'NONE',  ( 0.000000000000000000, 0.000000000000000000, -1.000000000000000000 ) ) ;
#3179=CARTESIAN_POINT ( 'NONE',  ( 134.0023458843163269, -3659.955155772517628, 2244.552343395693697 ) ) ;
#3182=CARTESIAN_POINT ( 'NONE',  ( 15.48441936004095609, -3660.088012435405744, 2250.236355021178952 ) ) ;
#3183=EDGE_CURVE ( 'NONE', #21998, #5432, #15957, .T. ) ;
#3184=DIRECTION ( 'NONE',  ( 0.000000000000000000, 0.000000000000000000, -1.000000000000000000 ) ) ;
#3191=CARTESIAN_POINT ( 'NONE',  ( 123.3932000000010021, -3619.500000000000000, 2239.009999999999764 ) ) ;
#3195=CARTESIAN_POINT ( 'NONE',  ( 141.6086330389385353, -3657.395487126937496, 2248.141035207103869 ) ) ;
#3197=EDGE_LOOP ( 'NONE', ( #20907, #13516, #18847, #11703, #4967, #1479, #15417, #4245 ) ) ;
#3199=DIRECTION ( 'NONE',  ( 1.224646799147353207E-16, 1.000000000000000000, -0.000000000000000000 ) ) ;
#3200=ORIENTED_EDGE ( 'NONE', *, *, #8644, .T. ) ;
#3201=ORIENTED_EDGE ( 'NONE', *, *, #11389, .T. ) ;
#3202=PLANE ( 'NONE',  #20756 ) ;
#3203=EDGE_LOOP ( 'NONE', ( #7978, #20087, #11756, #156 ) ) ;
#3211=VERTEX_POINT ( 'NONE', #16943 ) ;
#3212=CIRCLE ( 'NONE', #23047, 2.844800000000001550 ) ;
#3218=AXIS2_PLACEMENT_3D ( 'NONE', #8395, #13428, #15424 ) ;
#3220=VERTEX_POINT ( 'NONE', #6184 ) ;
#3222=EDGE_CURVE ( 'NONE', #7743, #4703, #17828, .T. ) ;
#3225=VECTOR ( 'NONE', #1470, 1000.000000000000000 ) ;
#3227=CARTESIAN_POINT ( 'NONE',  ( 10.90747266517406011, -3581.704041953448268, 2247.289616970143470 ) ) ;
#3229=ORIENTED_EDGE ( 'NONE', *, *, #4364, .F. ) ;
#3235=CARTESIAN_POINT ( 'NONE',  ( 50.79999999999999716, -3568.700000000000273, 2259.837999999999738 ) ) ;
#3236=AXIS2_PLACEMENT_3D ( 'NONE', #12461, #3199, #19608 ) ;
#3239=AXIS2_PLACEMENT_3D ( 'NONE', #12375, #1471, #13906 ) ;
#3241=DIRECTION ( 'NONE',  ( -1.000000000000000000, 0.000000000000000000, 0.000000000000000000 ) ) ;
#3243=CARTESIAN_POINT ( 'NONE',  ( 134.0203227398999957, -3578.860230781999689, 2244.548186305999934 ) ) ;
#3244=LINE ( 'NONE', #1477, #1976 ) ;
#3245=CARTESIAN_POINT ( 'NONE',  ( 50.79999999999999716, -3619.500000000000000, 2259.837999999999738 ) ) ;
#3246=ORIENTED_EDGE ( 'NONE', *, *, #18195, .T. ) ;
#3248=EDGE_CURVE ( 'NONE', #7121, #16307, #9906, .T. ) ;
#3249=CIRCLE ( 'NONE', #11121, 3.606799999998994366 ) ;
#3250=ORIENTED_EDGE ( 'NONE', *, *, #19700, .T. ) ;
#3255=PLANE ( 'NONE',  #7573 ) ;
#3256=EDGE_CURVE ( 'NONE', #11901, #10278, #11660, .T. ) ;
#3259=DIRECTION ( 'NONE',  ( 0.000000000000000000, 0.000000000000000000, -1.000000000000000000 ) ) ;
#3262=ORIENTED_EDGE ( 'NONE', *, *, #20859, .F. ) ;
#3266=CARTESIAN_POINT ( 'NONE',  ( 95.25000000000000000, -3695.699999999999818, 2243.277199999999993 ) ) ;
#3267=CARTESIAN_POINT ( 'NONE',  ( 10.59562833397165171, -3657.590649014947303, 2248.654563546086138 ) ) ;
#3268=ADVANCED_FACE ( 'NONE', ( #4763 ), #2999, .T. ) ;
#3271=VERTEX_POINT ( 'NONE', #11444 ) ;
#3272=DIRECTION ( 'NONE',  ( 1.224646799147353207E-16, 1.000000000000000000, -0.000000000000000000 ) ) ;
#3273=ORIENTED_EDGE ( 'NONE', *, *, #16870, .T. ) ;
#3278=DIRECTION ( 'NONE',  ( 0.000000000000000000, -1.000000000000000000, 0.000000000000000000 ) ) ;
#3279=ORIENTED_EDGE ( 'NONE', *, *, #13685, .T. ) ;
#3284=CARTESIAN_POINT ( 'NONE',  ( 97.99320000000000164, -3568.700000000000273, 2239.771999999999935 ) ) ;
#3286=DIRECTION ( 'NONE',  ( 0.000000000000000000, 0.000000000000000000, -1.000000000000000000 ) ) ;
#3287=AXIS2_PLACEMENT_3D ( 'NONE', #1083, #6148, #4488 ) ;
#3288=DIRECTION ( 'NONE',  ( 0.000000000000000000, 0.000000000000000000, -1.000000000000000000 ) ) ;
#3289=CARTESIAN_POINT ( 'NONE',  ( 127.0000000000000000, -3578.860000000000127, 2247.392000000000280 ) ) ;
#3291=CARTESIAN_POINT ( 'NONE',  ( 15.55727146409452821, -3695.607672421357620, 2254.979487869122295 ) ) ;
#3293=ORIENTED_EDGE ( 'NONE', *, *, #15391, .F. ) ;
#3294=DIRECTION ( 'NONE',  ( 0.000000000000000000, 0.000000000000000000, -1.000000000000000000 ) ) ;
#3295=EDGE_CURVE ( 'NONE', #5223, #11524, #23067, .T. ) ;
#3296=DIRECTION ( 'NONE',  ( 0.000000000000000000, 0.000000000000000000, -1.000000000000000000 ) ) ;
#3298=VERTEX_POINT ( 'NONE', #9794 ) ;
#3300=DIRECTION ( 'NONE',  ( 0.000000000000000000, 0.000000000000000000, -1.000000000000000000 ) ) ;
#3301=VERTEX_POINT ( 'NONE', #882 ) ;
#3305=DIRECTION ( 'NONE',  ( 0.7249994335945011414, 6.337882393833011158E-14, 0.6887494619146010688 ) ) ;
#3309=CARTESIAN_POINT ( 'NONE',  ( 18.36105254568060019, -3580.284312841101382, 2244.927052815691695 ) ) ;
#3310=CARTESIAN_POINT ( 'NONE',  ( 141.6126669512999854, -3657.399152860999493, 2246.630000000000109 ) ) ;
#3314=ORIENTED_EDGE ( 'NONE', *, *, #9099, .F. ) ;
#3315=ORIENTED_EDGE ( 'NONE', *, *, #22331, .T. ) ;
#3318=EDGE_LOOP ( 'NONE', ( #3707, #135, #3279, #3349 ) ) ;
#3319=ORIENTED_EDGE ( 'NONE', *, *, #2265, .F. ) ;
#3320=CARTESIAN_POINT ( 'NONE',  ( 4.878250543320599597, -3543.555041885565970, 2260.094480151607968 ) ) ;
#3322=DIRECTION ( 'NONE',  ( 0.000000000000000000, 0.000000000000000000, -1.000000000000000000 ) ) ;
#3324=ORIENTED_EDGE ( 'NONE', *, *, #6354, .T. ) ;
#3326=CARTESIAN_POINT ( 'NONE',  ( 63.50000000000000000, -3594.099999999999909, 2259.837999999999738 ) ) ;
#3327=CARTESIAN_POINT ( 'NONE',  ( 25.39999999999999858, -3619.500000000000000, 2260.600000000000364 ) ) ;
#3330=ORIENTED_EDGE ( 'NONE', *, *, #14544, .F. ) ;
#3333=CARTESIAN_POINT ( 'NONE',  ( 18.41500000000100101, -3579.494999999999891, 2239.771999999999935 ) ) ;
#3336=CARTESIAN_POINT ( 'NONE',  ( 10.87628247337022636, -3581.678378035377136, 2246.973460001757303 ) ) ;
#3337=ORIENTED_EDGE ( 'NONE', *, *, #1656, .T. ) ;
#3341=AXIS2_PLACEMENT_3D ( 'NONE', #17167, #22555, #6526 ) ;
#3343=EDGE_CURVE ( 'NONE', #6627, #22920, #12983, .T. ) ;
#3347=CARTESIAN_POINT ( 'NONE',  ( 12.63689026076125721, -3662.349833683567795, 2249.183488215769103 ) ) ;
#3349=ORIENTED_EDGE ( 'NONE', *, *, #15885, .F. ) ;
#3352=EDGE_LOOP ( 'NONE', ( #20811, #2532 ) ) ;
#3353=DIRECTION ( 'NONE',  ( 0.000000000000000000, 0.000000000000000000, -1.000000000000000000 ) ) ;
#3354=DIRECTION ( 'NONE',  ( 0.000000000000000000, 0.000000000000000000, -1.000000000000000000 ) ) ;
#3356=CARTESIAN_POINT ( 'NONE',  ( 14.84429988771011466, -3657.635452944057306, 2248.741321748801511 ) ) ;
#3359=EDGE_CURVE ( 'NONE', #20703, #2146, #17452, .T. ) ;
#3360=DIRECTION ( 'NONE',  ( 0.000000000000000000, 0.000000000000000000, -1.000000000000000000 ) ) ;
#3361=ORIENTED_EDGE ( 'NONE', *, *, #17352, .F. ) ;
#3364=ADVANCED_FACE ( 'NONE', ( #16009 ), #15594, .T. ) ;
#3370=DIRECTION ( 'NONE',  ( -1.000000000000000000, 0.000000000000000000, 0.000000000000000000 ) ) ;
#3374=DIRECTION ( 'NONE',  ( 0.000000000000000000, 0.000000000000000000, -1.000000000000000000 ) ) ;
#3375=EDGE_CURVE ( 'NONE', #8201, #2255, #10345, .T. ) ;
#3379=LINE ( 'NONE', #17554, #14801 ) ;
#3382=ADVANCED_FACE ( 'NONE', ( #17760 ), #18577, .T. ) ;
#3386=CARTESIAN_POINT ( 'NONE',  ( 132.1456718464000062, -3694.678775005999796, 2260.506484774000000 ) ) ;
#3389=DIRECTION ( 'NONE',  ( 0.6723379328151413148, 0.7402443543167774864, 0.000000000000000000 ) ) ;
#3391=LINE ( 'NONE', #15596, #18095 ) ;
#3397=DIRECTION ( 'NONE',  ( 1.000000000000000000, 0.000000000000000000, 0.000000000000000000 ) ) ;
#3399=EDGE_CURVE ( 'NONE', #21490, #18111, #3663, .T. ) ;
#3402=DIRECTION ( 'NONE',  ( 0.000000000000000000, 0.000000000000000000, 1.000000000000000000 ) ) ;
#3404=FACE_OUTER_BOUND ( 'NONE', #8035, .T. ) ;
#3406=CARTESIAN_POINT ( 'NONE',  ( 151.1299999999999955, -3578.860000000000127, 2247.392000000000280 ) ) ;
#3407=EDGE_LOOP ( 'NONE', ( #21322, #4039 ) ) ;
#3409=EDGE_CURVE ( 'NONE', #10931, #16647, #22682, .T. ) ;
#3411=CARTESIAN_POINT ( 'NONE',  ( 20.17309679552000290, -3544.443975155000317, 2260.454626673999883 ) ) ;
#3413=ADVANCED_FACE ( 'NONE', ( #19637 ), #3580, .F. ) ;
#3417=DIRECTION ( 'NONE',  ( 1.224646799147353207E-16, 1.000000000000000000, -0.000000000000000000 ) ) ;
#3418=CYLINDRICAL_SURFACE ( 'NONE', #1505, 1.270000000000000018 ) ;
#3419=( NAMED_UNIT ( * ) PLANE_ANGLE_UNIT ( ) SI_UNIT ( $, .RADIAN. ) );
#3420=EDGE_CURVE ( 'NONE', #13646, #20939, #5902, .T. ) ;
#3422=DIRECTION ( 'NONE',  ( 0.000000000000000000, 0.000000000000000000, 1.000000000000000000 ) ) ;
#3425=DIRECTION ( 'NONE',  ( 1.000000000000000000, 0.000000000000000000, 0.000000000000000000 ) ) ;
#3429=DIRECTION ( 'NONE',  ( 0.000000000000000000, 0.000000000000000000, -1.000000000000000000 ) ) ;
#3438=CARTESIAN_POINT ( 'NONE',  ( 123.3932000000010021, -3670.300000000000182, 2260.600000000000364 ) ) ;
#3439=ORIENTED_EDGE ( 'NONE', *, *, #20177, .F. ) ;
#3441=CARTESIAN_POINT ( 'NONE',  ( 142.5447999999993272, -3659.956214629431543, 2256.063560000000962 ) ) ;
#3445=ORIENTED_EDGE ( 'NONE', *, *, #333, .T. ) ;
#3446=DIRECTION ( 'NONE',  ( 0.000000000000000000, 0.000000000000000000, 1.000000000000000000 ) ) ;
#3447=FACE_BOUND ( 'NONE', #19442, .T. ) ;
#3453=CARTESIAN_POINT ( 'NONE',  ( 131.8035393939117341, -3543.438513001066440, 2259.907745842177974 ) ) ;
#3457=DIRECTION ( 'NONE',  ( 0.000000000000000000, 0.000000000000000000, -1.000000000000000000 ) ) ;
#3459=FACE_BOUND ( 'NONE', #1750, .T. ) ;
#3460=DIRECTION ( 'NONE',  ( -1.000000000000000000, 0.000000000000000000, 0.000000000000000000 ) ) ;
#3461=DIRECTION ( 'NONE',  ( -0.000000000000000000, 1.000000000000000000, 0.000000000000000000 ) ) ;
#3462=DIRECTION ( 'NONE',  ( 0.000000000000000000, -1.000000000000000000, 0.000000000000000000 ) ) ;
#3464=CARTESIAN_POINT ( 'NONE',  ( 9.926995637850000165, -3660.140002548000211, 2250.236801297000056 ) ) ;
#3465=DIRECTION ( 'NONE',  ( 0.000000000000000000, 0.000000000000000000, 1.000000000000000000 ) ) ;
#3470=AXIS2_PLACEMENT_3D ( 'NONE', #19594, #22977, #14209 ) ;
#3472=CARTESIAN_POINT ( 'NONE',  ( 15.00430973647434207, -3657.836720156582942, 2249.062018686695865 ) ) ;
#3473=CARTESIAN_POINT ( 'NONE',  ( 137.0287870094147422, -3695.282573428062278, 2255.445345400565202 ) ) ;
#3474=CARTESIAN_POINT ( 'NONE',  ( 10.37685559933697554, -3577.852505989571910, 2250.052669706260076 ) ) ;
#3475=ORIENTED_EDGE ( 'NONE', *, *, #19626, .F. ) ;
#3476=EDGE_CURVE ( 'NONE', #9977, #19601, #23081, .T. ) ;
#3477=CARTESIAN_POINT ( 'NONE',  ( 132.2768405780999785, -3544.527728670999750, 2260.413001451000127 ) ) ;
#3478=EDGE_CURVE ( 'NONE', #14198, #5385, #10364, .T. ) ;
#3482=EDGE_CURVE ( 'NONE', #19496, #3614, #18592, .T. ) ;
#3483=PLANE ( 'NONE',  #7214 ) ;
#3484=DIRECTION ( 'NONE',  ( -1.000000000000000000, 0.000000000000000000, 0.000000000000000000 ) ) ;
#3485=CARTESIAN_POINT ( 'NONE',  ( 20.09942059832000183, -3694.430000000000291, 2260.390449568000349 ) ) ;
#3486=AXIS2_PLACEMENT_3D ( 'NONE', #9986, #22396, #11398 ) ;
#3487=CYLINDRICAL_SURFACE ( 'NONE', #16375, 1.269999999999898099 ) ;
#3488=DIRECTION ( 'NONE',  ( -0.7249994335945011414, 0.000000000000000000, 0.6887494619146010688 ) ) ;
#3491=EDGE_LOOP ( 'NONE', ( #17907, #11275 ) ) ;
#3493=CARTESIAN_POINT ( 'NONE',  ( 18.41499999999999915, -3659.504999999999654, 2246.630000000000109 ) ) ;
#3497=ORIENTED_EDGE ( 'NONE', *, *, #5585, .T. ) ;
#3499=CARTESIAN_POINT ( 'NONE',  ( 142.5447969220999767, -3659.599750067000059, 2250.186720660999981 ) ) ;
#3503=CARTESIAN_POINT ( 'NONE',  ( 136.8708886487836480, -3579.840085227391228, 2250.069118183399041 ) ) ;
#3504=EDGE_CURVE ( 'NONE', #16691, #10464, #22326, .T. ) ;
#3505=ORIENTED_EDGE ( 'NONE', *, *, #9833, .T. ) ;
#3506=CARTESIAN_POINT ( 'NONE',  ( 145.4149999194000316, -3579.495498070999474, 2244.618783703000190 ) ) ;
#3507=ADVANCED_FACE ( 'NONE', ( #11192 ), #1827, .T. ) ;
#3510=FACE_OUTER_BOUND ( 'NONE', #13026, .T. ) ;
#3511=CARTESIAN_POINT ( 'NONE',  ( 139.6999999999999886, -3659.504999999999654, 2246.630000000000109 ) ) ;
#3512=CIRCLE ( 'NONE', #10626, 2.844800000000091700 ) ;
#3514=DIRECTION ( 'NONE',  ( 0.000000000000000000, -1.000000000000000000, 0.000000000000000000 ) ) ;
#3515=EDGE_LOOP ( 'NONE', ( #14355, #15325, #10772, #722, #20412, #21842, #22936, #4256, #6040 ) ) ;
#3516=FACE_OUTER_BOUND ( 'NONE', #12231, .T. ) ;
#3518=VERTEX_POINT ( 'NONE', #1945 ) ;
#3519=CARTESIAN_POINT ( 'NONE',  ( 5.080000000000000071, -3694.746619019253558, 2260.599999999999454 ) ) ;
#3520=DIRECTION ( 'NONE',  ( 0.7249994335944036639, 0.000000000000000000, 0.6887494619147036534 ) ) ;
#3521=FACE_OUTER_BOUND ( 'NONE', #17562, .T. ) ;
#3522=ORIENTED_EDGE ( 'NONE', *, *, #5424, .T. ) ;
#3527=CIRCLE ( 'NONE', #4664, 4.114799999999974034 ) ;
#3531=DIRECTION ( 'NONE',  ( 0.000000000000000000, 0.000000000000000000, -1.000000000000000000 ) ) ;
#3536=DIRECTION ( 'NONE',  ( 1.000000000000000000, 0.000000000000000000, 0.000000000000000000 ) ) ;
#3538=CARTESIAN_POINT ( 'NONE',  ( 147.8270794805000037, -3695.699999999999818, 2259.329999999999927 ) ) ;
#3540=CARTESIAN_POINT ( 'NONE',  ( 136.9819489059368323, -3658.646220300227014, 2249.821879689220168 ) ) ;
#3542=CIRCLE ( 'NONE', #2488, 4.114799999999974034 ) ;
#3543=ORIENTED_EDGE ( 'NONE', *, *, #7244, .F. ) ;
#3544=AXIS2_PLACEMENT_3D ( 'NONE', #9275, #16407, #21687 ) ;
#3545=CARTESIAN_POINT ( 'NONE',  ( 34.49320000000000164, -3644.899999999999636, 2260.600000000000364 ) ) ;
#3546=AXIS2_PLACEMENT_3D ( 'NONE', #7593, #16496, #1861 ) ;
#3547=ORIENTED_EDGE ( 'NONE', *, *, #2009, .T. ) ;
#3552=DIRECTION ( 'NONE',  ( 0.000000000000000000, 0.000000000000000000, -1.000000000000000000 ) ) ;
#3553=ORIENTED_EDGE ( 'NONE', *, *, #8384, .T. ) ;
#3554=ORIENTED_EDGE ( 'NONE', *, *, #8673, .T. ) ;
#3558=DIRECTION ( 'NONE',  ( 1.000000000000000000, 0.000000000000000000, 0.000000000000000000 ) ) ;
#3559=ADVANCED_FACE ( 'NONE', ( #2183 ), #21606, .T. ) ;
#3562=EDGE_CURVE ( 'NONE', #8027, #9982, #6264, .T. ) ;
#3565=B_SPLINE_CURVE_WITH_KNOTS ( 'NONE', 3,
 ( #7621, #22339, #14781, #1128 ),
 .UNSPECIFIED., .F., .F.,
 ( 4, 4 ),
 ( 0.000000000000000000, 1.000000000000000000 ),
 .UNSPECIFIED. ) ;
#3566=AXIS2_PLACEMENT_3D ( 'NONE', #12523, #19671, #1746 ) ;
#3576=DIRECTION ( 'NONE',  ( 1.000000000000000000, 0.000000000000000000, 0.000000000000000000 ) ) ;
#3578=CARTESIAN_POINT ( 'NONE',  ( 10.16000000000000014, -3660.786127253999894, 2255.774000000000342 ) ) ;
#3579=DIRECTION ( 'NONE',  ( 0.000000000000000000, 0.000000000000000000, 1.000000000000000000 ) ) ;
#3580=CYLINDRICAL_SURFACE ( 'NONE', #7749, 2.844800000000091700 ) ;
#3582=CYLINDRICAL_SURFACE ( 'NONE', #13634, 2.844800000000001550 ) ;
#3584=CARTESIAN_POINT ( 'NONE',  ( 147.5628652634462128, -3543.485052021266711, 2259.991528816362461 ) ) ;
#3591=CARTESIAN_POINT ( 'NONE',  ( 14.60426581554083825, -3657.391551304373479, 2248.126455225663904 ) ) ;
#3593=DIRECTION ( 'NONE',  ( 0.000000000000000000, 0.000000000000000000, -1.000000000000000000 ) ) ;
#3594=EDGE_LOOP ( 'NONE', ( #12986, #3899, #22604, #15326 ) ) ;
#3595=VECTOR ( 'NONE', #1333, 1000.000000000000000 ) ;
#3596=CARTESIAN_POINT ( 'NONE',  ( 10.01417881486321271, -3543.678681369438891, 2255.408746714403605 ) ) ;
#3599=DIRECTION ( 'NONE',  ( 0.000000000000000000, 0.000000000000000000, 1.000000000000000000 ) ) ;
#3601=DIRECTION ( 'NONE',  ( -0.7249994335945011414, -6.625572310377011455E-14, -0.6887494619146010688 ) ) ;
#3602=AXIS2_PLACEMENT_3D ( 'NONE', #10731, #12488, #1706 ) ;
#3608=DIRECTION ( 'NONE',  ( 0.000000000000000000, 0.000000000000000000, -1.000000000000000000 ) ) ;
#3611=VERTEX_POINT ( 'NONE', #5934 ) ;
#3612=DIRECTION ( 'NONE',  ( 0.000000000000000000, 0.000000000000000000, 1.000000000000000000 ) ) ;
#3613=AXIS2_PLACEMENT_3D ( 'NONE', #17482, #17597, #8703 ) ;
#3614=VERTEX_POINT ( 'NONE', #21705 ) ;
#3616=FACE_OUTER_BOUND ( 'NONE', #20784, .T. ) ;
#3617=AXIS2_PLACEMENT_3D ( 'NONE', #6325, #8424, #12168 ) ;
#3618=AXIS2_PLACEMENT_3D ( 'NONE', #18906, #17025, #2617 ) ;
#3620=VERTEX_POINT ( 'NONE', #10806 ) ;
#3622=CARTESIAN_POINT ( 'NONE',  ( 137.5384828158008759, -3581.344674309946186, 2248.777575039056501 ) ) ;
#3624=DIRECTION ( 'NONE',  ( -1.000000000000000000, -2.186138625658999988E-13, 0.000000000000000000 ) ) ;
#3626=CARTESIAN_POINT ( 'NONE',  ( 151.4000000000000057, -3694.430000000000291, 2240.279999999999745 ) ) ;
#3634=CARTESIAN_POINT ( 'NONE',  ( 134.8493656935452520, -3576.472980476652083, 2245.844349661984779 ) ) ;
#3635=CIRCLE ( 'NONE', #12262, 2.844799999999994444 ) ;
#3644=DIRECTION ( 'NONE',  ( 0.000000000000000000, 0.000000000000000000, 1.000000000000000000 ) ) ;
#3657=CARTESIAN_POINT ( 'NONE',  ( 129.8447999999989975, -3670.300000000000182, 2259.837999999999738 ) ) ;
#3661=CARTESIAN_POINT ( 'NONE',  ( 137.7873330486999919, -3657.399152860999493, 2246.630000000000109 ) ) ;
#3663=B_SPLINE_CURVE_WITH_KNOTS ( 'NONE', 3,
 ( #3114, #1710, #8629, #1357, #22790, #7110 ),
 .UNSPECIFIED., .F., .F.,
 ( 4, 1, 1, 4 ),
 ( 0.000000000000000000, 0.3333333333333000081, 0.6666666666667000474, 1.000000000000000000 ),
 .UNSPECIFIED. ) ;
#3665=CARTESIAN_POINT ( 'NONE',  ( 137.5048382467581973, -3661.314614866817010, 2249.983038987777491 ) ) ;
#3669=VERTEX_POINT ( 'NONE', #15854 ) ;
#3671=VERTEX_POINT ( 'NONE', #9050 ) ;
#3672=EDGE_LOOP ( 'NONE', ( #21112, #2496 ) ) ;
#3677=EDGE_CURVE ( 'NONE', #21672, #10931, #1790, .T. ) ;
#3680=CARTESIAN_POINT ( 'NONE',  ( 1.270000000000000018, -3694.430000000000291, 2239.009999999999764 ) ) ;
#3682=CARTESIAN_POINT ( 'NONE',  ( 7.387125747139000609, -3581.600847139000052, 2246.630000000000109 ) ) ;
#3683=DIRECTION ( 'NONE',  ( 0.000000000000000000, 1.000000000000000000, 0.000000000000000000 ) ) ;
#3686=CARTESIAN_POINT ( 'NONE',  ( 131.7910775263680705, -3543.423052263211048, 2259.876519366634511 ) ) ;
#3690=ORIENTED_EDGE ( 'NONE', *, *, #12800, .T. ) ;
#3692=FACE_OUTER_BOUND ( 'NONE', #7113, .T. ) ;
#3694=CARTESIAN_POINT ( 'NONE',  ( 145.3474457849973192, -3578.572730242030048, 2244.547227117760031 ) ) ;
#3697=CARTESIAN_POINT ( 'NONE',  ( 147.5856715291725720, -3543.452888078975775, 2259.934476224082118 ) ) ;
#3699=DIRECTION ( 'NONE',  ( -0.000000000000000000, 1.000000000000000000, 0.000000000000000000 ) ) ;
#3701=CARTESIAN_POINT ( 'NONE',  ( 151.4000000000000057, -3660.140000000000327, 2244.518167364599321 ) ) ;
#3703=FACE_OUTER_BOUND ( 'NONE', #14086, .T. ) ;
#3704=CARTESIAN_POINT ( 'NONE',  ( 142.4278116317892113, -3543.579977979913565, 2255.303812752575141 ) ) ;
#3705=DIRECTION ( 'NONE',  ( 1.224646799147353207E-16, 1.000000000000000000, -0.000000000000000000 ) ) ;
#3706=CARTESIAN_POINT ( 'NONE',  ( 7.700590725981468765, -3576.724945326997840, 2245.509351448440157 ) ) ;
#3707=ORIENTED_EDGE ( 'NONE', *, *, #17142, .F. ) ;
#3708=DIRECTION ( 'NONE',  ( 0.000000000000000000, 0.000000000000000000, 1.000000000000000000 ) ) ;
#3718=DIRECTION ( 'NONE',  ( -1.000000000000000000, 0.000000000000000000, 0.000000000000000000 ) ) ;
#3720=ORIENTED_EDGE ( 'NONE', *, *, #3134, .F. ) ;
#3724=DIRECTION ( 'NONE',  ( 0.000000000000000000, 0.000000000000000000, 1.000000000000000000 ) ) ;
#3725=B_SPLINE_CURVE_WITH_KNOTS ( 'NONE', 3,
 ( #34, #17601, #12685, #14215, #18071, #152, #21598, #12568, #5310, #9173, #274, #1552, #8706, #22984, #19603, #16314, #15855, #7298, #7074, #6956, #14100, #10807, #8938, #14451 ),
 .UNSPECIFIED., .F., .F.,
 ( 4, 2, 2, 1, 1, 1, 2, 2, 2, 2, 1, 2, 2, 4 ),
 ( 0.000000000000000000, 0.1249999999958202324, 0.1874999999936646511, 0.2187499999925868743, 0.2343749999925359984, 0.2421874999925105743, 0.2460937499923391558, 0.2499999999921677096, 0.3749999999942763562, 0.4374999999955747620, 0.4687499999961892705, 0.4843749999962707609, 0.4999999999963522512, 1.000000000000000000 ),
 .UNSPECIFIED. ) ;
#3726=VECTOR ( 'NONE', #14539, 1000.000000000000000 ) ;
#3728=CARTESIAN_POINT ( 'NONE',  ( 25.39999999999999858, -3619.500000000000000, 2259.837999999999738 ) ) ;
#3729=CARTESIAN_POINT ( 'NONE',  ( 1.270000000000000018, -3660.140000000000327, 2247.392000000000280 ) ) ;
#3731=CIRCLE ( 'NONE', #21691, 1.269999999999882334 ) ;
#3732=ORIENTED_EDGE ( 'NONE', *, *, #1841, .T. ) ;
#3733=ORIENTED_EDGE ( 'NONE', *, *, #15826, .T. ) ;
#3734=CARTESIAN_POINT ( 'NONE',  ( 137.4641237087990930, -3581.254761593761941, 2248.929472245830311 ) ) ;
#3735=VERTEX_POINT ( 'NONE', #19484 ) ;
#3736=DIRECTION ( 'NONE',  ( 0.000000000000000000, -1.000000000000000000, 0.000000000000000000 ) ) ;
#3738=CARTESIAN_POINT ( 'NONE',  ( 92.50679999999999836, -3594.099999999999909, 2260.600000000000364 ) ) ;
#3743=CARTESIAN_POINT ( 'NONE',  ( 140.5358672174552339, -3576.775707768860229, 2249.328148595326638 ) ) ;
#3745=CARTESIAN_POINT ( 'NONE',  ( 134.7245833821262977, -3576.682656229064833, 2245.560154887602948 ) ) ;
#3746=CARTESIAN_POINT ( 'NONE',  ( 101.5999999999999943, -3670.300000000000182, 2239.771999999999935 ) ) ;
#3750=LINE ( 'NONE', #9038, #7618 ) ;
#3751=EDGE_LOOP ( 'NONE', ( #1917, #10305, #3998, #14179 ) ) ;
#3752=DIRECTION ( 'NONE',  ( 0.000000000000000000, 0.000000000000000000, -1.000000000000000000 ) ) ;
#3754=AXIS2_PLACEMENT_3D ( 'NONE', #325, #9459, #11214 ) ;
#3765=EDGE_CURVE ( 'NONE', #10812, #159, #11871, .T. ) ;
#3767=CARTESIAN_POINT ( 'NONE',  ( 15.24000000000000021, -3544.570000000000164, 2254.503999999999905 ) ) ;
#3768=ORIENTED_EDGE ( 'NONE', *, *, #13381, .F. ) ;
#3770=EDGE_CURVE ( 'NONE', #3611, #8104, #9631, .T. ) ;
#3771=EDGE_CURVE ( 'NONE', #2160, #2800, #10569, .T. ) ;
#3772=CARTESIAN_POINT ( 'NONE',  ( 137.5597418815846993, -3657.630783818591681, 2248.732918511922435 ) ) ;
#3775=CARTESIAN_POINT ( 'NONE',  ( 140.4840675020349750, -3662.239671886142332, 2249.311457353029709 ) ) ;
#3776=EDGE_CURVE ( 'NONE', #7043, #20273, #293, .T. ) ;
#3780=LINE ( 'NONE', #17853, #10301 ) ;
#3785=CARTESIAN_POINT ( 'NONE',  ( 127.0000000000000000, -3578.860000000000127, 2250.236800000000130 ) ) ;
#3786=CIRCLE ( 'NONE', #9421, 1.269999999999882334 ) ;
#3787=CARTESIAN_POINT ( 'NONE',  ( 50.79999999999999716, -3568.700000000000273, 2239.771999999999935 ) ) ;
#3789=ADVANCED_FACE ( 'NONE', ( #11377 ), #12633, .T. ) ;
#3792=DIRECTION ( 'NONE',  ( 0.000000000000000000, 0.000000000000000000, 1.000000000000000000 ) ) ;
#3796=ORIENTED_EDGE ( 'NONE', *, *, #22442, .T. ) ;
#3798=ORIENTED_EDGE ( 'NONE', *, *, #16236, .F. ) ;
#3803=CARTESIAN_POINT ( 'NONE',  ( 8.027948531603557925, -3662.797778259959614, 2246.366055962258542 ) ) ;
#3805=AXIS2_PLACEMENT_3D ( 'NONE', #20772, #4601, #4953 ) ;
#3806=FACE_OUTER_BOUND ( 'NONE', #5199, .T. ) ;
#3807=CIRCLE ( 'NONE', #11651, 3.606799999998994366 ) ;
#3811=CARTESIAN_POINT ( 'NONE',  ( 18.14025602003983906, -3657.753732795579708, 2245.841877976950400 ) ) ;
#3813=DIRECTION ( 'NONE',  ( -1.000000000000000000, 0.000000000000000000, 0.000000000000000000 ) ) ;
#3817=AXIS2_PLACEMENT_3D ( 'NONE', #18692, #4296, #20461 ) ;
#3820=CARTESIAN_POINT ( 'NONE',  ( 142.2399999999999807, -3544.490134411880717, 2255.773999999999432 ) ) ;
#3821=CARTESIAN_POINT ( 'NONE',  ( 137.0230491797765637, -3695.298184790851792, 2255.430966980177800 ) ) ;
#3825=ORIENTED_EDGE ( 'NONE', *, *, #8014, .F. ) ;
#3827=AXIS2_PLACEMENT_3D ( 'NONE', #16734, #13103, #9806 ) ;
#3833=AXIS2_PLACEMENT_3D ( 'NONE', #14709, #5811, #5462 ) ;
#3836=ADVANCED_FACE ( 'NONE', ( #15022 ), #16425, .T. ) ;
#3837=ADVANCED_FACE ( 'NONE', ( #13250 ), #9274, .T. ) ;
#3838=ORIENTED_EDGE ( 'NONE', *, *, #18375, .F. ) ;
#3839=DIRECTION ( 'NONE',  ( 1.000000000000000000, 0.000000000000000000, 0.000000000000000000 ) ) ;
#3841=AXIS2_PLACEMENT_3D ( 'NONE', #22084, #7807, #2744 ) ;
#3842=LINE ( 'NONE', #16383, #18171 ) ;
#3843=AXIS2_PLACEMENT_3D ( 'NONE', #756, #19013, #6056 ) ;
#3846=EDGE_CURVE ( 'NONE', #1882, #923, #17866, .T. ) ;
#3850=CARTESIAN_POINT ( 'NONE',  ( 142.7013569010373146, -3695.699999999983902, 2254.618513953578713 ) ) ;
#3851=DIRECTION ( 'NONE',  ( -1.000000000000000000, 0.000000000000000000, 0.000000000000000000 ) ) ;
#3856=CARTESIAN_POINT ( 'NONE',  ( 137.8408795312830932, -3581.648507417375640, 2247.961733200111667 ) ) ;
#3859=DIRECTION ( 'NONE',  ( -0.000000000000000000, -1.000000000000000000, -0.000000000000000000 ) ) ;
#3861=CIRCLE ( 'NONE', #2380, 2.844800000000001550 ) ;
#3862=CARTESIAN_POINT ( 'NONE',  ( 76.20000000000000284, -3670.300000000000182, 2261.869999999999891 ) ) ;
#3866=CARTESIAN_POINT ( 'NONE',  ( 104.4447999999999865, -3619.500000000000000, 2259.837999999999738 ) ) ;
#3867=ORIENTED_EDGE ( 'NONE', *, *, #7657, .T. ) ;
#3869=CARTESIAN_POINT ( 'NONE',  ( 134.6728313949629126, -3576.776753335464946, 2245.454731746178368 ) ) ;
#3870=VECTOR ( 'NONE', #3593, 1000.000000000000000 ) ;
#3871=ORIENTED_EDGE ( 'NONE', *, *, #2237, .T. ) ;
#3875=DIRECTION ( 'NONE',  ( 1.000000000000000000, 0.000000000000000000, 0.000000000000000000 ) ) ;
#3878=ORIENTED_EDGE ( 'NONE', *, *, #13239, .F. ) ;
#3882=FACE_OUTER_BOUND ( 'NONE', #20720, .T. ) ;
#3884=CARTESIAN_POINT ( 'NONE',  ( 141.6126318482000102, -3581.600863517000107, 2246.630000000000109 ) ) ;
#3885=ORIENTED_EDGE ( 'NONE', *, *, #3295, .F. ) ;
#3887=TOROIDAL_SURFACE ( 'NONE', #874, 4.114799999999999791, 1.270000000000000018 ) ;
#3891=CARTESIAN_POINT ( 'NONE',  ( 5.080000000000000071, -3694.430000000000291, 2260.600000000000364 ) ) ;
#3893=CARTESIAN_POINT ( 'NONE',  ( 18.12625886363281680, -3581.288617098281520, 2245.910525600300844 ) ) ;
#3894=CARTESIAN_POINT ( 'NONE',  ( 137.6837585684422436, -3657.497605245348495, 2248.447085333438281 ) ) ;
#3896=ORIENTED_EDGE ( 'NONE', *, *, #1346, .F. ) ;
#3897=CARTESIAN_POINT ( 'NONE',  ( 140.4495444393403716, -3662.249331053435071, 2249.300837621843584 ) ) ;
#3899=ORIENTED_EDGE ( 'NONE', *, *, #23035, .F. ) ;
#3903=CARTESIAN_POINT ( 'NONE',  ( 9.880094305751999428, -3579.102405584999815, 2250.228735751999920 ) ) ;
#3907=ORIENTED_EDGE ( 'NONE', *, *, #12800, .F. ) ;
#3910=ADVANCED_FACE ( 'NONE', ( #1288 ), #20869, .T. ) ;
#3911=ORIENTED_EDGE ( 'NONE', *, *, #10259, .T. ) ;
#3913=( NAMED_UNIT ( * ) SI_UNIT ( $, .STERADIAN. ) SOLID_ANGLE_UNIT ( ) );
#3914=DIRECTION ( 'NONE',  ( 0.000000000000000000, -1.000000000000000000, 0.000000000000000000 ) ) ;
#3919=AXIS2_PLACEMENT_3D ( 'NONE', #13904, #14144, #3460 ) ;
#3920=CARTESIAN_POINT ( 'NONE',  ( 1.270000000000000018, -3578.860000000000127, 2247.392000000000280 ) ) ;
#3921=CARTESIAN_POINT ( 'NONE',  ( 8.088613972621001125, -3662.880847139000252, 2246.630000000000109 ) ) ;
#3924=ORIENTED_EDGE ( 'NONE', *, *, #1965, .T. ) ;
#3925=CARTESIAN_POINT ( 'NONE',  ( 25.39999999999999858, -3568.700000000000273, 2259.837999999999738 ) ) ;
#3927=DIRECTION ( 'NONE',  ( 0.000000000000000000, 0.000000000000000000, -1.000000000000000000 ) ) ;
#3928=DIRECTION ( 'NONE',  ( -1.000000000000000000, 0.000000000000000000, 0.000000000000000000 ) ) ;
#3929=CARTESIAN_POINT ( 'NONE',  ( 18.06698106831952089, -3657.540322655302134, 2246.234995830579010 ) ) ;
#3934=DIRECTION ( 'NONE',  ( 0.000000000000000000, 0.000000000000000000, 1.000000000000000000 ) ) ;
#3935=EDGE_CURVE ( 'NONE', #2255, #11877, #11139, .T. ) ;
#3936=DIRECTION ( 'NONE',  ( 0.000000000000000000, 0.000000000000000000, -1.000000000000000000 ) ) ;
#3937=AXIS2_PLACEMENT_3D ( 'NONE', #6911, #14181, #5033 ) ;
#3938=EDGE_CURVE ( 'NONE', #22780, #23086, #16172, .T. ) ;
#3939=DIRECTION ( 'NONE',  ( 0.000000000000000000, 0.000000000000000000, -1.000000000000000000 ) ) ;
#3940=CIRCLE ( 'NONE', #579, 2.844799999999994444 ) ;
#3941=CARTESIAN_POINT ( 'NONE',  ( 142.2559700947606416, -3544.251379751714467, 2255.734053407719330 ) ) ;
#3943=CARTESIAN_POINT ( 'NONE',  ( 7.365006562230047571, -3577.445405246308383, 2244.922385902951191 ) ) ;
#3944=ORIENTED_EDGE ( 'NONE', *, *, #8005, .T. ) ;
#3947=DIRECTION ( 'NONE',  ( -1.000000000000000000, 0.000000000000000000, 0.000000000000000000 ) ) ;
#3950=CARTESIAN_POINT ( 'NONE',  ( 0.000000000000000000, -3544.570000000000164, 2259.329999999999927 ) ) ;
#3951=DIRECTION ( 'NONE',  ( 1.000000000000000000, 0.000000000000000000, 0.000000000000000000 ) ) ;
#3952=EDGE_CURVE ( 'NONE', #6059, #18860, #10007, .T. ) ;
#3955=CARTESIAN_POINT ( 'NONE',  ( 134.8602052428276181, -3662.544438751693178, 2245.871466275956209 ) ) ;
#3961=DIRECTION ( 'NONE',  ( 0.000000000000000000, -1.000000000000000000, 0.000000000000000000 ) ) ;
#3963=CARTESIAN_POINT ( 'NONE',  ( 7.387125747152000876, -3657.399152860999493, 2246.630000000000109 ) ) ;
#3964=EDGE_CURVE ( 'NONE', #17959, #8199, #2168, .T. ) ;
#3965=ORIENTED_EDGE ( 'NONE', *, *, #12435, .F. ) ;
#3966=CARTESIAN_POINT ( 'NONE',  ( 142.2559348849416381, -3694.748620251596094, 2255.734039348222268 ) ) ;
#3967=DIRECTION ( 'NONE',  ( 1.000000000000000000, 0.000000000000000000, 0.000000000000000000 ) ) ;
#3969=CIRCLE ( 'NONE', #17420, 2.844799999998995244 ) ;
#3975=ORIENTED_EDGE ( 'NONE', *, *, #17116, .F. ) ;
#3976=DIRECTION ( 'NONE',  ( 0.000000000000000000, 0.000000000000000000, 1.000000000000000000 ) ) ;
#3980=DIRECTION ( 'NONE',  ( -1.000000000000000000, 0.000000000000000000, 0.000000000000000000 ) ) ;
#3982=B_SPLINE_CURVE_WITH_KNOTS ( 'NONE', 3,
 ( #3661, #19729, #21712, #19606, #15972, #2149, #19487, #7186, #7420, #5557, #10810, #18075, #5663, #12802, #19957, #9054, #3894, #10698, #7076, #12689, #14456, #21254, #11042, #155, #18191, #3772, #9296, #19837, #10926, #5313, #2026, #22987, #6960, #14105, #5198, #10583, #17847, #37, #21484, #12457, #17720, #1668, #5430, #8827, #23106, #16088, #14219, #14340, #3540, #13039, #7527, #719, #16773 ),
 .UNSPECIFIED., .F., .F.,
 ( 4, 2, 2, 2, 2, 1, 2, 2, 2, 2, 1, 1, 1, 2, 2, 2, 2, 2, 2, 1, 1, 2, 2, 2, 2, 1, 2, 2, 2, 4 ),
 ( 0.000000000000000000, 0.1249999999841666931, 0.1874999999764063452, 0.2499999999686460250, 0.3124999999608856771, 0.3437499999571574927, 0.3593749999553250141, 0.3749999999534924799, 0.4374999999467432121, 0.4687499999434819875, 0.4843749999417981122, 0.4921874999409536211, 0.4960937499405312923, 0.4980468749403176298, 0.4999999999401039119, 0.5312499999398715422, 0.5624999999396390615, 0.5937499999394066919, 0.6093749999393713868, 0.6171874999394474370, 0.6210937499395690065, 0.6230468749397405359, 0.6249999999399119543, 0.6874999999489770364, 0.7187499999536707262, 0.7343749999559984198, 0.7421874999571623777, 0.7499999999583262245, 0.8749999999791631122, 1.000000000000000000 ),
 .UNSPECIFIED. ) ;
#3983=DIRECTION ( 'NONE',  ( -1.000000000000000000, 0.000000000000000000, 0.000000000000000000 ) ) ;
#3984=CARTESIAN_POINT ( 'NONE',  ( 114.2999999999999972, -3594.099999999999909, 2259.837999999999738 ) ) ;
#3985=CARTESIAN_POINT ( 'NONE',  ( 140.5955809558492149, -3576.794761112849756, 2249.348465679632682 ) ) ;
#3987=CARTESIAN_POINT ( 'NONE',  ( 134.4913178369996842, -3577.143244214250444, 2245.123591688256056 ) ) ;
#3988=EDGE_CURVE ( 'NONE', #21259, #20612, #15361, .T. ) ;
#3993=EDGE_LOOP ( 'NONE', ( #3965, #18312, #10822, #19610 ) ) ;
#3997=CIRCLE ( 'NONE', #7001, 3.606800000000000228 ) ;
#3998=ORIENTED_EDGE ( 'NONE', *, *, #3083, .T. ) ;
#4004=CARTESIAN_POINT ( 'NONE',  ( 10.71531464684066393, -3577.456266983200749, 2249.866613545771088 ) ) ;
#4006=FACE_OUTER_BOUND ( 'NONE', #21444, .T. ) ;
#4008=CIRCLE ( 'NONE', #22742, 2.844800000000091700 ) ;
#4009=DIRECTION ( 'NONE',  ( 0.000000000000000000, 0.000000000000000000, -1.000000000000000000 ) ) ;
#4014=EDGE_LOOP ( 'NONE', ( #2973, #10326, #10370, #21609 ) ) ;
#4015=DIRECTION ( 'NONE',  ( 0.000000000000000000, 0.000000000000000000, -1.000000000000000000 ) ) ;
#4020=CARTESIAN_POINT ( 'NONE',  ( 137.3526213507248315, -3661.114307651350828, 2250.065742440782742 ) ) ;
#4022=VERTEX_POINT ( 'NONE', #20984 ) ;
#4024=AXIS2_PLACEMENT_3D ( 'NONE', #19454, #18992, #22953 ) ;
#4025=DIRECTION ( 'NONE',  ( 0.000000000000000000, -1.000000000000000000, 0.000000000000000000 ) ) ;
#4029=DIRECTION ( 'NONE',  ( 0.000000000000000000, 0.000000000000000000, -1.000000000000000000 ) ) ;
#4032=CARTESIAN_POINT ( 'NONE',  ( 38.10000000000000142, -3594.099999999999909, 2259.837999999999738 ) ) ;
#4033=AXIS2_PLACEMENT_3D ( 'NONE', #5781, #18299, #14678 ) ;
#4034=DIRECTION ( 'NONE',  ( 0.000000000000000000, -1.000000000000000000, 0.000000000000000000 ) ) ;
#4035=LINE ( 'NONE', #20094, #21831 ) ;
#4038=CARTESIAN_POINT ( 'NONE',  ( 114.2999999999999972, -3594.099999999999909, 2239.771999999999935 ) ) ;
#4039=ORIENTED_EDGE ( 'NONE', *, *, #11851, .T. ) ;
#4042=CARTESIAN_POINT ( 'NONE',  ( 7.719554562072720394, -3662.307856581991018, 2245.543048782076312 ) ) ;
#4043=ORIENTED_EDGE ( 'NONE', *, *, #13116, .T. ) ;
#4044=FACE_OUTER_BOUND ( 'NONE', #21478, .T. ) ;
#4045=AXIS2_PLACEMENT_3D ( 'NONE', #19867, #19986, #5927 ) ;
#4047=DIRECTION ( 'NONE',  ( 1.000000000000000000, 0.000000000000000000, 0.000000000000000000 ) ) ;
#4049=CARTESIAN_POINT ( 'NONE',  ( 18.20822205038428621, -3657.980541937662565, 2245.538019395683932 ) ) ;
#4051=CARTESIAN_POINT ( 'NONE',  ( 147.4346999979424595, -3695.234698870522152, 2260.312749946543590 ) ) ;
#4053=DIRECTION ( 'NONE',  ( 0.000000000000000000, 0.000000000000000000, 1.000000000000000000 ) ) ;
#4055=CARTESIAN_POINT ( 'NONE',  ( 142.3295600303597723, -3543.848287275569874, 2255.549808268773177 ) ) ;
#4057=CARTESIAN_POINT ( 'NONE',  ( 7.608775882559566384, -3576.898905879581889, 2245.331008237134029 ) ) ;
#4061=ORIENTED_EDGE ( 'NONE', *, *, #2237, .F. ) ;
#4062=DIRECTION ( 'NONE',  ( -1.224646799147353207E-16, 1.000000000000000000, 0.000000000000000000 ) ) ;
#4063=CARTESIAN_POINT ( 'NONE',  ( 129.8447999999989975, -3568.700000000000273, 2261.869999999999891 ) ) ;
#4067=EDGE_CURVE ( 'NONE', #15488, #11524, #17485, .T. ) ;
#4068=ORIENTED_EDGE ( 'NONE', *, *, #7235, .T. ) ;
#4069=CARTESIAN_POINT ( 'NONE',  ( 135.0283457588961653, -3662.798513796493353, 2246.367958887603891 ) ) ;
#4072=FACE_OUTER_BOUND ( 'NONE', #17930, .T. ) ;
#4075=DIRECTION ( 'NONE',  ( 0.000000000000000000, 0.000000000000000000, -1.000000000000000000 ) ) ;
#4077=CARTESIAN_POINT ( 'NONE',  ( 35.56000000000000227, -3694.430000000000291, 2247.392000000000280 ) ) ;
#4081=CARTESIAN_POINT ( 'NONE',  ( 63.50000000000000000, -3644.899999999999636, 2259.837999999999738 ) ) ;
#4083=CARTESIAN_POINT ( 'NONE',  ( 38.10000000000000142, -3644.899999999999636, 2259.837999999999738 ) ) ;
#4085=EDGE_CURVE ( 'NONE', #13188, #13105, #6668, .T. ) ;
#4086=ORIENTED_EDGE ( 'NONE', *, *, #7098, .F. ) ;
#4091=CARTESIAN_POINT ( 'NONE',  ( 145.2535822323377204, -3580.844011437738573, 2245.352786166252372 ) ) ;
#4093=CARTESIAN_POINT ( 'NONE',  ( 145.4120474421716835, -3579.283774594628539, 2244.576911952362025 ) ) ;
#4094=FACE_OUTER_BOUND ( 'NONE', #2155, .T. ) ;
#4095=CARTESIAN_POINT ( 'NONE',  ( 131.7757523116999891, -3544.570000000000164, 2260.600000000000364 ) ) ;
#4096=ADVANCED_FACE ( 'NONE', ( #3510 ), #10662, .F. ) ;
#4098=CARTESIAN_POINT ( 'NONE',  ( 142.3952936667693905, -3578.572481595138925, 2250.225737411198679 ) ) ;
#4099=ORIENTED_EDGE ( 'NONE', *, *, #3935, .F. ) ;
#4100=CIRCLE ( 'NONE', #17927, 3.606800000000000228 ) ;
#4102=VERTEX_POINT ( 'NONE', #3738 ) ;
#4103=CARTESIAN_POINT ( 'NONE',  ( 15.24000000000000021, -3544.570000000000164, 2255.774000000000342 ) ) ;
#4108=APPLICATION_CONTEXT ( 'configuration controlled 3d designs of mechanical parts and assemblies' ) ;
#4114=CARTESIAN_POINT ( 'NONE',  ( 12.05677975596295148, -3576.723661194017041, 2249.270583004743003 ) ) ;
#4116=DIRECTION ( 'NONE',  ( 0.000000000000000000, -1.000000000000000000, 0.000000000000000000 ) ) ;
#4120=CARTESIAN_POINT ( 'NONE',  ( 20.37131446257999912, -3694.758336080999925, 2260.557504193999648 ) ) ;
#4126=VERTEX_POINT ( 'NONE', #12313 ) ;
#4127=VERTEX_POINT ( 'NONE', #7049 ) ;
#4128=CARTESIAN_POINT ( 'NONE',  ( 137.3063811338797962, -3661.044633701663770, 2250.090170880306232 ) ) ;
#4131=EDGE_CURVE ( 'NONE', #10003, #20430, #17528, .T. ) ;
#4134=CARTESIAN_POINT ( 'NONE',  ( 29.00679999999900005, -3619.500000000000000, 2260.600000000000364 ) ) ;
#4140=EDGE_CURVE ( 'NONE', #287, #16201, #10095, .T. ) ;
#4143=CARTESIAN_POINT ( 'NONE',  ( 7.108545037236568831, -3658.323337185065611, 2245.202519759302504 ) ) ;
#4144=FACE_BOUND ( 'NONE', #18395, .T. ) ;
#4146=CARTESIAN_POINT ( 'NONE',  ( 127.0000000000000000, -3670.300000000000182, 2260.600000000000364 ) ) ;
#4147=EDGE_CURVE ( 'NONE', #5084, #21589, #14226, .T. ) ;
#4150=CARTESIAN_POINT ( 'NONE',  ( 25.39999999999999858, -3578.860000000000127, 2244.547199999999975 ) ) ;
#4151=CARTESIAN_POINT ( 'NONE',  ( 142.3647906480871654, -3658.508756101628933, 2249.722899581812726 ) ) ;
#4152=CARTESIAN_POINT ( 'NONE',  ( 7.261600995315486529, -3661.299381583153718, 2244.776454689257207 ) ) ;
#4161=TOROIDAL_SURFACE ( 'NONE', #7528, 3.606799999999999784, 0.7620000000000000107 ) ;
#4162=CARTESIAN_POINT ( 'NONE',  ( 18.34551793137252673, -3658.616110195214333, 2244.989057792325184 ) ) ;
#4163=VERTEX_POINT ( 'NONE', #22955 ) ;
#4164=CARTESIAN_POINT ( 'NONE',  ( 147.4837490350197982, -3695.367664692139897, 2260.189857417176881 ) ) ;
#4168=CARTESIAN_POINT ( 'NONE',  ( 142.3769508200778375, -3543.701815209601591, 2255.430966980605717 ) ) ;
#4171=CARTESIAN_POINT ( 'NONE',  ( 7.176225798281845591, -3578.028891693621517, 2244.671246062090177 ) ) ;
#4172=ORIENTED_EDGE ( 'NONE', *, *, #9441, .F. ) ;
#4174=VERTEX_POINT ( 'NONE', #14303 ) ;
#4175=CARTESIAN_POINT ( 'NONE',  ( 145.0670228868914933, -3657.540459061100591, 2246.234687787927669 ) ) ;
#4176=VECTOR ( 'NONE', #1227, 1000.000000000000000 ) ;
#4180=ORIENTED_EDGE ( 'NONE', *, *, #22002, .F. ) ;
#4183=LINE ( 'NONE', #670, #2770 ) ;
#4185=CARTESIAN_POINT ( 'NONE',  ( 15.21739391844383960, -3660.839252834448416, 2250.153081304058560 ) ) ;
#4187=CARTESIAN_POINT ( 'NONE',  ( 54.40679999999999694, -3670.300000000000182, 2259.837999999999738 ) ) ;
#4188=ORIENTED_EDGE ( 'NONE', *, *, #4067, .F. ) ;
#4190=AXIS2_PLACEMENT_3D ( 'NONE', #4831, #6490, #2961 ) ;
#4191=CARTESIAN_POINT ( 'NONE',  ( 116.8400000000000034, -3670.300000000000182, 2250.236800000000130 ) ) ;
#4193=ADVANCED_FACE ( 'NONE', ( #12422 ), #21335, .T. ) ;
#4194=ORIENTED_EDGE ( 'NONE', *, *, #409, .T. ) ;
#4195=DIRECTION ( 'NONE',  ( -1.000000000000000000, 0.000000000000000000, 0.000000000000000000 ) ) ;
#4197=EDGE_CURVE ( 'NONE', #16752, #11962, #5621, .T. ) ;
#4198=ORIENTED_EDGE ( 'NONE', *, *, #17352, .T. ) ;
#4199=ORIENTED_EDGE ( 'NONE', *, *, #5148, .T. ) ;
#4200=EDGE_CURVE ( 'NONE', #4775, #22886, #19572, .T. ) ;
#4203=CARTESIAN_POINT ( 'NONE',  ( 145.2205435179829749, -3580.973142349780119, 2245.487016221928570 ) ) ;
#4205=AXIS2_PLACEMENT_3D ( 'NONE', #15656, #17751, #16001 ) ;
#4207=EDGE_CURVE ( 'NONE', #13662, #12207, #11225, .T. ) ;
#4208=CARTESIAN_POINT ( 'NONE',  ( 17.73574364357449085, -3662.207325212531487, 2245.437750342633080 ) ) ;
#4213=CIRCLE ( 'NONE', #19927, 1.269999999999882334 ) ;
#4214=CARTESIAN_POINT ( 'NONE',  ( 140.8264938607258614, -3576.881393884998488, 2249.436472243866319 ) ) ;
#4216=CARTESIAN_POINT ( 'NONE',  ( 60.65520000000000067, -3644.899999999999636, 2261.869999999999891 ) ) ;
#4220=CARTESIAN_POINT ( 'NONE',  ( 15.57690423030046745, -3543.373434453245409, 2254.929879518507278 ) ) ;
#4222=ORIENTED_EDGE ( 'NONE', *, *, #13000, .T. ) ;
#4224=ORIENTED_EDGE ( 'NONE', *, *, #827, .T. ) ;
#4228=ORIENTED_EDGE ( 'NONE', *, *, #1640, .F. ) ;
#4229=EDGE_CURVE ( 'NONE', #10620, #13850, #7386, .T. ) ;
#4231=DIRECTION ( 'NONE',  ( 0.000000000000000000, 0.000000000000000000, -1.000000000000000000 ) ) ;
#4232=CARTESIAN_POINT ( 'NONE',  ( 11.49846512652514363, -3576.916035655123324, 2249.469127929353363 ) ) ;
#4233=CARTESIAN_POINT ( 'NONE',  ( 141.9145117060755297, -3581.280835468015539, 2248.886214331544579 ) ) ;
#4235=DIRECTION ( 'NONE',  ( 1.000000000000000000, 0.000000000000000000, 0.000000000000000000 ) ) ;
#4238=CARTESIAN_POINT ( 'NONE',  ( 79.80679999999999552, -3568.700000000000273, 2239.771999999999935 ) ) ;
#4239=DIRECTION ( 'NONE',  ( 0.000000000000000000, 1.000000000000000000, 0.000000000000000000 ) ) ;
#4240=ORIENTED_EDGE ( 'NONE', *, *, #8538, .F. ) ;
#4244=EDGE_CURVE ( 'NONE', #749, #4022, #6735, .T. ) ;
#4245=ORIENTED_EDGE ( 'NONE', *, *, #17133, .F. ) ;
#4247=CARTESIAN_POINT ( 'NONE',  ( 142.0581284917780067, -3661.097254891949433, 2250.071354168025209 ) ) ;
#4249=VERTEX_POINT ( 'NONE', #16508 ) ;
#4254=FACE_OUTER_BOUND ( 'NONE', #19590, .T. ) ;
#4256=ORIENTED_EDGE ( 'NONE', *, *, #7221, .F. ) ;
#4258=( NAMED_UNIT ( * ) PLANE_ANGLE_UNIT ( ) SI_UNIT ( $, .RADIAN. ) );
#4260=B_SPLINE_CURVE_WITH_KNOTS ( 'NONE', 3,
 ( #4526, #18479, #13434, #4418, #4185, #18702, #9908, #7823, #15202, #883, #11789, #10034, #13201, #8050, #8170, #6306, #775, #11662, #7708, #20244, #9690, #14972, #18821, #2765, #17057, #11446, #1008, #14864, #20693, #11330, #22440, #6415, #4640, #2435, #4306, #674, #18943, #17176, #9578, #16724, #22104, #20357, #18596, #12029, #14024, #3347, #17289, #10500, #22791, #10616, #14147, #8751, #21057, #22564, #4876, #23028, #17641, #10149, #1591, #22908, #8523, #20936, #1241, #15545, #10384, #12140, #7002, #6885, #5002, #19410, #15897, #13792, #19179, #22683, #6656, #12267, #13907, #3001, #21175, #15430, #5124, #21293, #3115, #5235, #12376, #15780, #1472, #10264, #17524, #19524, #8630, #3464 ),
 .UNSPECIFIED., .F., .F.,
 ( 4, 2, 2, 2, 1, 1, 2, 2, 2, 2, 1, 2, 2, 2, 2, 1, 2, 2, 2, 2, 2, 2, 2, 2, 2, 2, 2, 2, 1, 2, 2, 2, 2, 1, 1, 2, 2, 2, 1, 2, 2, 1, 2, 2, 2, 2, 1, 2, 2, 2, 4 ),
 ( 0.000000000000000000, 0.06250000000004160561, 0.1250000000000832112, 0.1562500000001531830, 0.1718750000002726430, 0.1796875000003080869, 0.1835937500003257672, 0.1875000000003434752, 0.2187500000002969291, 0.2343750000002473299, 0.2421875000001830203, 0.2460937500001633693, 0.2500000000001437184, 0.2656250000001137979, 0.2812500000000838773, 0.2968750000000539013, 0.3046875000000662248, 0.3125000000000784928, 0.3437500000001323386, 0.3593750000001595946, 0.3671875000002268741, 0.3750000000002942091, 0.4062500000004605760, 0.4375000000006269429, 0.5000000000010219603, 0.5312500000012198020, 0.5625000000014177548, 0.5937500000016155965, 0.6093750000017141844, 0.6171875000017874591, 0.6250000000018607338, 0.6562500000022088997, 0.6718750000024367175, 0.6796875000025764946, 0.6835937500026186830, 0.6855468750026141311, 0.6875000000026094682, 0.7031250000027079450, 0.7109375000027615688, 0.7148437500027633451, 0.7187500000027652325, 0.7343750000026652014, 0.7421875000025792701, 0.7500000000024933389, 0.7812500000021941338, 0.7968750000020254909, 0.8046875000019169111, 0.8085937500018625101, 0.8125000000018082202, 0.8750000000012380097, 1.000000000000000000 ),
 .UNSPECIFIED. ) ;
#4263=EDGE_CURVE ( 'NONE', #21351, #12349, #2603, .T. ) ;
#4264=ADVANCED_FACE ( 'NONE', ( #20044 ), #15712, .T. ) ;
#4266=DIRECTION ( 'NONE',  ( -1.000000000000000000, 0.000000000000000000, 0.000000000000000000 ) ) ;
#4268=ADVANCED_FACE ( 'NONE', ( #5754 ), #21790, .F. ) ;
#4270=CIRCLE ( 'NONE', #11012, 4.114799999999974034 ) ;
#4272=CIRCLE ( 'NONE', #17354, 2.844799999999009010 ) ;
#4275=EDGE_CURVE ( 'NONE', #6642, #15313, #11238, .T. ) ;
#4277=EDGE_LOOP ( 'NONE', ( #4388, #19502 ) ) ;
#4279=DIRECTION ( 'NONE',  ( 0.000000000000000000, 0.000000000000000000, -1.000000000000000000 ) ) ;
#4285=CYLINDRICAL_SURFACE ( 'NONE', #8576, 2.844799999999994444 ) ;
#4290=ORIENTED_EDGE ( 'NONE', *, *, #17425, .T. ) ;
#4295=CARTESIAN_POINT ( 'NONE',  ( 145.0394780070161005, -3657.466321062724546, 2246.411837555674538 ) ) ;
#4296=DIRECTION ( 'NONE',  ( 1.000000000000000000, 0.000000000000000000, 0.000000000000000000 ) ) ;
#4298=ORIENTED_EDGE ( 'NONE', *, *, #19987, .F. ) ;
#4301=CARTESIAN_POINT ( 'NONE',  ( 111.4552000000009997, -3594.099999999999909, 2239.771999999999935 ) ) ;
#4302=B_SPLINE_CURVE_WITH_KNOTS ( 'NONE', 3,
 ( #13606, #14914, #6008, #20625, #9737, #13141, #20514, #18752, #20748, #826, #20298, #4693, #22262, #18874, #9511, #11380, #6124, #18528, #4461, #18417, #4355, #2701, #13251 ),
 .UNSPECIFIED., .F., .F.,
 ( 4, 2, 2, 1, 1, 2, 2, 2, 2, 1, 2, 2, 4 ),
 ( 0.000000000000000000, 0.1250000000057876759, 0.1875000000086804175, 0.2187500000100172926, 0.2343750000102403086, 0.2421875000102004238, 0.2500000000101605391, 0.3750000000068593464, 0.4375000000056980531, 0.4687500000047965520, 0.4843750000046709858, 0.5000000000045454751, 1.000000000000000000 ),
 .UNSPECIFIED. ) ;
#4303=ORIENTED_EDGE ( 'NONE', *, *, #17422, .T. ) ;
#4305=AXIS2_PLACEMENT_3D ( 'NONE', #71, #23136, #9211 ) ;
#4306=CARTESIAN_POINT ( 'NONE',  ( 13.66119911539924026, -3662.182772986108375, 2249.372110354217966 ) ) ;
#4313=CYLINDRICAL_SURFACE ( 'NONE', #20920, 2.844799999998995244 ) ;
#4315=EDGE_LOOP ( 'NONE', ( #16089, #3871, #9853, #19218 ) ) ;
#4319=ORIENTED_EDGE ( 'NONE', *, *, #20548, .T. ) ;
#4323=CIRCLE ( 'NONE', #2454, 2.844799999998998796 ) ;
#4324=CARTESIAN_POINT ( 'NONE',  ( 145.3852444848333789, -3578.912497749951399, 2244.547653759440436 ) ) ;
#4325=DIRECTION ( 'NONE',  ( -1.000000000000000000, 0.000000000000000000, 0.000000000000000000 ) ) ;
#4326=AXIS2_PLACEMENT_3D ( 'NONE', #15834, #10670, #17818 ) ;
#4330=CARTESIAN_POINT ( 'NONE',  ( 50.79999999999999716, -3619.500000000000000, 2239.009999999999764 ) ) ;
#4332=DIRECTION ( 'NONE',  ( 0.000000000000000000, 0.000000000000000000, -1.000000000000000000 ) ) ;
#4334=ORIENTED_EDGE ( 'NONE', *, *, #1942, .F. ) ;
#4335=AXIS2_PLACEMENT_3D ( 'NONE', #14029, #10744, #8982 ) ;
#4336=DIRECTION ( 'NONE',  ( -1.000000000000000000, 0.000000000000000000, 0.000000000000000000 ) ) ;
#4337=CARTESIAN_POINT ( 'NONE',  ( 15.48293133199724103, -3543.482543407366393, 2255.165289490807481 ) ) ;
#4340=CIRCLE ( 'NONE', #2470, 2.844800000000091700 ) ;
#4342=EDGE_LOOP ( 'NONE', ( #21033, #12869 ) ) ;
#4344=CIRCLE ( 'NONE', #11833, 3.606799999999001027 ) ;
#4345=VERTEX_POINT ( 'NONE', #2115 ) ;
#4347=CARTESIAN_POINT ( 'NONE',  ( 11.91900528410963211, -3576.759436215039386, 2249.310481143603283 ) ) ;
#4348=CARTESIAN_POINT ( 'NONE',  ( 141.8830647757983741, -3581.319234992912698, 2248.822303562533762 ) ) ;
#4353=DIRECTION ( 'NONE',  ( -1.224646799147353207E-16, 1.000000000000000000, 0.000000000000000000 ) ) ;
#4355=CARTESIAN_POINT ( 'NONE',  ( 20.42964990730697039, -3543.731305792769490, 2260.325288752524102 ) ) ;
#4359=EDGE_CURVE ( 'NONE', #17172, #13234, #13100, .T. ) ;
#4361=B_SPLINE_CURVE_WITH_KNOTS ( 'NONE', 3,
 ( #10940, #169, #7318, #17859 ),
 .UNSPECIFIED., .F., .F.,
 ( 4, 4 ),
 ( 0.000000000000000000, 1.000000000000000000 ),
 .UNSPECIFIED. ) ;
#4364=EDGE_CURVE ( 'NONE', #5314, #15707, #11132, .T. ) ;
#4370=CARTESIAN_POINT ( 'NONE',  ( 139.6999999999999886, -3659.504999999999654, 2239.771999999999935 ) ) ;
#4371=EDGE_CURVE ( 'NONE', #20621, #9389, #9974, .T. ) ;
#4381=DIRECTION ( 'NONE',  ( 0.000000000000000000, 0.000000000000000000, -1.000000000000000000 ) ) ;
#4383=ORIENTED_EDGE ( 'NONE', *, *, #11771, .T. ) ;
#4384=CARTESIAN_POINT ( 'NONE',  ( 136.8622934043370094, -3543.413280444360680, 2255.028323493608241 ) ) ;
#4385=EDGE_CURVE ( 'NONE', #21408, #11171, #12346, .T. ) ;
#4388=ORIENTED_EDGE ( 'NONE', *, *, #19258, .F. ) ;
#4392=ADVANCED_FACE ( 'NONE', ( #6203 ), #15339, .T. ) ;
#4395=ORIENTED_EDGE ( 'NONE', *, *, #17604, .T. ) ;
#4396=ORIENTED_EDGE ( 'NONE', *, *, #8889, .F. ) ;
#4398=AXIS2_PLACEMENT_3D ( 'NONE', #5164, #17213, #3389 ) ;
#4402=CARTESIAN_POINT ( 'NONE',  ( 73.35520000000001062, -3670.300000000000182, 2259.837999999999738 ) ) ;
#4404=ORIENTED_EDGE ( 'NONE', *, *, #17016, .T. ) ;
#4406=AXIS2_PLACEMENT_3D ( 'NONE', #11623, #1079, #13627 ) ;
#4407=CARTESIAN_POINT ( 'NONE',  ( 21.79320000000099711, -3619.500000000000000, 2260.600000000000364 ) ) ;
#4408=EDGE_CURVE ( 'NONE', #7794, #15892, #8973, .T. ) ;
#4412=ORIENTED_EDGE ( 'NONE', *, *, #5876, .T. ) ;
#4414=PLANE ( 'NONE',  #19629 ) ;
#4415=CARTESIAN_POINT ( 'NONE',  ( 134.9433685273030221, -3576.326160261962286, 2246.096241041220765 ) ) ;
#4416=VERTEX_POINT ( 'NONE', #22582 ) ;
#4418=CARTESIAN_POINT ( 'NONE',  ( 15.28666681192564525, -3660.698594568427779, 2250.184763937277239 ) ) ;
#4419=CIRCLE ( 'NONE', #11521, 3.606799999998994366 ) ;
#4420=ADVANCED_FACE ( 'NONE', ( #15219 ), #17947, .T. ) ;
#4426=DIRECTION ( 'NONE',  ( 0.000000000000000000, 0.000000000000000000, 1.000000000000000000 ) ) ;
#4429=ORIENTED_EDGE ( 'NONE', *, *, #14013, .F. ) ;
#4433=CARTESIAN_POINT ( 'NONE',  ( 145.2640895604332911, -3580.799603742848831, 2245.310931595014154 ) ) ;
#4435=EDGE_CURVE ( 'NONE', #17227, #15832, #11929, .T. ) ;
#4437=CARTESIAN_POINT ( 'NONE',  ( 18.29809890354264112, -3660.655555570265278, 2244.593310214874236 ) ) ;
#4441=DIRECTION ( 'NONE',  ( -1.000000000000000000, 0.000000000000000000, 0.000000000000000000 ) ) ;
#4442=ORIENTED_EDGE ( 'NONE', *, *, #14855, .F. ) ;
#4445=FACE_OUTER_BOUND ( 'NONE', #18036, .T. ) ;
#4452=VERTEX_POINT ( 'NONE', #8419 ) ;
#4454=CARTESIAN_POINT ( 'NONE',  ( 11.26161571375768133, -3577.038842554089115, 2249.578370015894961 ) ) ;
#4461=CARTESIAN_POINT ( 'NONE',  ( 20.52512745630702184, -3543.549679414229558, 2260.086245106032948 ) ) ;
#4462=AXIS2_PLACEMENT_3D ( 'NONE', #7470, #18129, #2088 ) ;
#4463=CARTESIAN_POINT ( 'NONE',  ( 136.9269754645999910, -3578.860002036999958, 2250.236803302000226 ) ) ;
#4464=VERTEX_POINT ( 'NONE', #13575 ) ;
#4465=CARTESIAN_POINT ( 'NONE',  ( 116.8400000000002734, -3670.300000000000182, 2244.547199999999975 ) ) ;
#4466=ORIENTED_EDGE ( 'NONE', *, *, #10291, .F. ) ;
#4468=ORIENTED_EDGE ( 'NONE', *, *, #2834, .T. ) ;
#4470=DIRECTION ( 'NONE',  ( 0.000000000000000000, 0.000000000000000000, 1.000000000000000000 ) ) ;
#4471=EDGE_LOOP ( 'NONE', ( #4404, #20592 ) ) ;
#4473=CARTESIAN_POINT ( 'NONE',  ( 67.10679999999999268, -3644.899999999999636, 2259.837999999999738 ) ) ;
#4475=ORIENTED_EDGE ( 'NONE', *, *, #7426, .F. ) ;
#4476=CARTESIAN_POINT ( 'NONE',  ( 0.000000000000000000, -3694.430000000000291, 2254.503999999999905 ) ) ;
#4477=ADVANCED_FACE ( 'NONE', ( #9816 ), #8304, .F. ) ;
#4482=DIRECTION ( 'NONE',  ( 1.000000000000000000, 0.000000000000000000, 0.000000000000000000 ) ) ;
#4486=DIRECTION ( 'NONE',  ( 0.000000000000000000, 0.000000000000000000, -1.000000000000000000 ) ) ;
#4487=LINE ( 'NONE', #22066, #22536 ) ;
#4488=DIRECTION ( 'NONE',  ( 0.000000000000000000, 0.000000000000000000, -1.000000000000000000 ) ) ;
#4489=EDGE_CURVE ( 'NONE', #15062, #4703, #11973, .T. ) ;
#4491=CARTESIAN_POINT ( 'NONE',  ( 136.6529205195000145, -3543.299999999999727, 2254.503999999999905 ) ) ;
#4494=ADVANCED_FACE ( 'NONE', ( #8651 ), #15797, .F. ) ;
#4496=EDGE_LOOP ( 'NONE', ( #20471, #13892, #2244, #17277 ) ) ;
#4498=CARTESIAN_POINT ( 'NONE',  ( 18.37220258132071393, -3658.807050315976994, 2244.878795110561441 ) ) ;
#4500=ORIENTED_EDGE ( 'NONE', *, *, #11923, .T. ) ;
#4501=DIRECTION ( 'NONE',  ( 1.000000000000000000, 0.000000000000000000, 0.000000000000000000 ) ) ;
#4502=FACE_OUTER_BOUND ( 'NONE', #6101, .T. ) ;
#4503=CARTESIAN_POINT ( 'NONE',  ( 130.6067999999989979, -3619.500000000000000, 2259.837999999999738 ) ) ;
#4504=CARTESIAN_POINT ( 'NONE',  ( 25.39999999999999858, -3660.140000000000327, 2250.236800000000130 ) ) ;
#4513=DIRECTION ( 'NONE',  ( 0.000000000000000000, 0.000000000000000000, 1.000000000000000000 ) ) ;
#4516=DIRECTION ( 'NONE',  ( 0.000000000000000000, 0.000000000000000000, 1.000000000000000000 ) ) ;
#4520=AXIS2_PLACEMENT_3D ( 'NONE', #2297, #14842, #3813 ) ;
#4521=EDGE_CURVE ( 'NONE', #19192, #10469, #17589, .T. ) ;
#4523=CARTESIAN_POINT ( 'NONE',  ( 144.9020910522499435, -3661.871258547513662, 2245.134603803046048 ) ) ;
#4526=CARTESIAN_POINT ( 'NONE',  ( 15.47291618100999955, -3660.140271294999820, 2250.236802488000194 ) ) ;
#4529=B_SPLINE_CURVE_WITH_KNOTS ( 'NONE', 3,
 ( #21356, #6718, #19475, #12212 ),
 .UNSPECIFIED., .F., .F.,
 ( 4, 4 ),
 ( 0.000000000000000000, 1.000000000000000000 ),
 .UNSPECIFIED. ) ;
#4530=CYLINDRICAL_SURFACE ( 'NONE', #9556, 2.844800000000001550 ) ;
#4532=DIRECTION ( 'NONE',  ( 0.000000000000000000, 0.000000000000000000, -1.000000000000000000 ) ) ;
#4533=CARTESIAN_POINT ( 'NONE',  ( 35.56000000000000227, -3670.300000000000182, 2250.236800000000130 ) ) ;
#4541=EDGE_CURVE ( 'NONE', #10440, #4464, #1874, .T. ) ;
#4543=CARTESIAN_POINT ( 'NONE',  ( 18.21995551375025357, -3660.985253975473825, 2244.675656256517868 ) ) ;
#4545=CARTESIAN_POINT ( 'NONE',  ( 57.14999999999999858, -3695.699999999999818, 2247.392000000000280 ) ) ;
#4548=ORIENTED_EDGE ( 'NONE', *, *, #13941, .F. ) ;
#4549=CIRCLE ( 'NONE', #1939, 2.844800000000091700 ) ;
#4553=DIRECTION ( 'NONE',  ( 0.6723379328173905156, 0.7402443543147344540, 0.000000000000000000 ) ) ;
#4554=CARTESIAN_POINT ( 'NONE',  ( 10.76878381091101389, -3657.415877871818793, 2248.216115161493235 ) ) ;
#4555=EDGE_CURVE ( 'NONE', #19652, #2680, #14619, .T. ) ;
#4558=ADVANCED_FACE ( 'NONE', ( #21312 ), #16478, .T. ) ;
#4565=AXIS2_PLACEMENT_3D ( 'NONE', #19402, #13897, #10139 ) ;
#4568=DIRECTION ( 'NONE',  ( 1.224646799147353207E-16, 1.000000000000000000, -0.000000000000000000 ) ) ;
#4570=CARTESIAN_POINT ( 'NONE',  ( 141.5925613388025397, -3581.618976631144051, 2248.085587691497039 ) ) ;
#4572=EDGE_LOOP ( 'NONE', ( #19850, #22853, #13047, #14458 ) ) ;
#4579=CARTESIAN_POINT ( 'NONE',  ( 134.3272858694121510, -3657.550344535092336, 2246.178645530484573 ) ) ;
#4580=ORIENTED_EDGE ( 'NONE', *, *, #12641, .F. ) ;
#4583=EDGE_LOOP ( 'NONE', ( #12321, #14783, #9126, #4412 ) ) ;
#4588=ORIENTED_EDGE ( 'NONE', *, *, #16015, .T. ) ;
#4589=ORIENTED_EDGE ( 'NONE', *, *, #2542, .F. ) ;
#4591=DIRECTION ( 'NONE',  ( 0.000000000000000000, 0.000000000000000000, -1.000000000000000000 ) ) ;
#4593=CARTESIAN_POINT ( 'NONE',  ( 7.138340810734780995, -3658.190072843201960, 2245.320604752622785 ) ) ;
#4600=DIRECTION ( 'NONE',  ( 1.000000000000000000, 0.000000000000000000, 0.000000000000000000 ) ) ;
#4601=DIRECTION ( 'NONE',  ( 0.000000000000000000, 0.000000000000000000, -1.000000000000000000 ) ) ;
#4602=DIRECTION ( 'NONE',  ( 0.000000000000000000, -1.000000000000000000, 0.000000000000000000 ) ) ;
#4605=AXIS2_PLACEMENT_3D ( 'NONE', #19354, #1176, #3171 ) ;
#4606=DIRECTION ( 'NONE',  ( 0.000000000000000000, 0.000000000000000000, 1.000000000000000000 ) ) ;
#4608=VERTEX_POINT ( 'NONE', #8996 ) ;
#4613=FACE_OUTER_BOUND ( 'NONE', #2979, .T. ) ;
#4614=EDGE_CURVE ( 'NONE', #444, #16167, #9005, .T. ) ;
#4617=ORIENTED_EDGE ( 'NONE', *, *, #6507, .T. ) ;
#4621=ORIENTED_EDGE ( 'NONE', *, *, #10817, .F. ) ;
#4622=CIRCLE ( 'NONE', #17719, 2.844799999998903761 ) ;
#4623=DIRECTION ( 'NONE',  ( -1.000000000000000000, 0.000000000000000000, 0.000000000000000000 ) ) ;
#4625=CARTESIAN_POINT ( 'NONE',  ( 151.1299999999999955, -3694.430000000000291, 2259.329999999999927 ) ) ;
#4626=CARTESIAN_POINT ( 'NONE',  ( 20.67261935617544211, -3695.639689706588797, 2259.716784108924458 ) ) ;
#4631=CARTESIAN_POINT ( 'NONE',  ( 9.935234496185218589, -3580.171483082290251, 2249.918062184726750 ) ) ;
#4634=DIRECTION ( 'NONE',  ( -1.000000000000000000, 0.000000000000000000, 0.000000000000000000 ) ) ;
#4636=CARTESIAN_POINT ( 'NONE',  ( 151.1299999999999955, -3660.140000000000327, 2250.236800000000130 ) ) ;
#4637=CARTESIAN_POINT ( 'NONE',  ( 144.7317021135920356, -3662.214841093968516, 2245.445731933329625 ) ) ;
#4639=EDGE_CURVE ( 'NONE', #10769, #10464, #667, .T. ) ;
#4640=CARTESIAN_POINT ( 'NONE',  ( 13.81460452052465548, -3662.123667865505922, 2249.431728352276878 ) ) ;
#4641=ADVANCED_FACE ( 'NONE', ( #22097 ), #14858, .F. ) ;
#4645=TOROIDAL_SURFACE ( 'NONE', #3158, 3.606799999999999784, 0.7620000000000000107 ) ;
#4646=CARTESIAN_POINT ( 'NONE',  ( 114.2999999999999972, -3644.899999999999636, 2260.600000000000364 ) ) ;
#4647=CIRCLE ( 'NONE', #2825, 2.844799999998995244 ) ;
#4652=EDGE_LOOP ( 'NONE', ( #5581, #20762, #10951, #12533 ) ) ;
#4656=ORIENTED_EDGE ( 'NONE', *, *, #13738, .F. ) ;
#4657=CARTESIAN_POINT ( 'NONE',  ( 9.802483769510930145, -3543.356150272095874, 2254.879165045093032 ) ) ;
#4660=DIRECTION ( 'NONE',  ( -1.000000000000000000, 0.000000000000000000, 0.000000000000000000 ) ) ;
#4664=AXIS2_PLACEMENT_3D ( 'NONE', #7673, #18566, #16801 ) ;
#4672=ORIENTED_EDGE ( 'NONE', *, *, #20736, .F. ) ;
#4674=CARTESIAN_POINT ( 'NONE',  ( 147.3199999999999932, -3694.509865589844594, 2260.599999999999454 ) ) ;
#4676=EDGE_LOOP ( 'NONE', ( #1747, #16232, #4198, #18671 ) ) ;
#4678=ORIENTED_EDGE ( 'NONE', *, *, #16727, .F. ) ;
#4679=DIRECTION ( 'NONE',  ( 0.000000000000000000, 0.000000000000000000, -1.000000000000000000 ) ) ;
#4680=CIRCLE ( 'NONE', #1314, 3.606799999999993567 ) ;
#4681=CIRCLE ( 'NONE', #12935, 1.269999999999882334 ) ;
#4688=CARTESIAN_POINT ( 'NONE',  ( 141.5487975361088218, -3581.657297964314694, 2247.911507805317342 ) ) ;
#4689=VERTEX_POINT ( 'NONE', #14514 ) ;
#4693=CARTESIAN_POINT ( 'NONE',  ( 20.63610976348933690, -3543.391099285847304, 2259.808358094443065 ) ) ;
#4694=ADVANCED_FACE ( 'NONE', ( #7364 ), #16713, .F. ) ;
#4695=CARTESIAN_POINT ( 'NONE',  ( 134.1088469025876861, -3658.321902597664575, 2245.203711442572057 ) ) ;
#4696=B_SPLINE_CURVE_WITH_KNOTS ( 'NONE', 3,
 ( #8525, #23030, #6657, #10619, #5354, #17526, #19062, #15782, #19300, #3003, #13908, #13793, #1473, #20938, #12030, #10265, #1360, #15668, #5004, #3584, #3697, #7675, #10851, #16578, #423, #12956, #21748, #1947, #18339, #12494, #2295 ),
 .UNSPECIFIED., .F., .F.,
 ( 4, 2, 2, 2, 2, 2, 1, 2, 2, 2, 2, 1, 1, 2, 2, 2, 4 ),
 ( 0.000000000000000000, 0.1250000000025272839, 0.1875000000034570125, 0.2500000000043867687, 0.3750000000065028538, 0.4375000000078326234, 0.4687500000080585538, 0.4843750000083739127, 0.5000000000086892715, 0.6250000000084229290, 0.6875000000085297325, 0.7187500000089692698, 0.7343750000091889829, 0.7421875000094193542, 0.7500000000096496144, 0.8750000000048248072, 1.000000000000000000 ),
 .UNSPECIFIED. ) ;
#4697=AXIS2_PLACEMENT_3D ( 'NONE', #8811, #23085, #20146 ) ;
#4698=ORIENTED_EDGE ( 'NONE', *, *, #8999, .F. ) ;
#4702=AXIS2_PLACEMENT_3D ( 'NONE', #1977, #5505, #19791 ) ;
#4703=VERTEX_POINT ( 'NONE', #20238 ) ;
#4704=DIRECTION ( 'NONE',  ( -1.000000000000000000, 0.000000000000000000, 0.000000000000000000 ) ) ;
#4707=CARTESIAN_POINT ( 'NONE',  ( 88.90000000000000568, -3644.899999999999636, 2239.009999999999764 ) ) ;
#4712=VERTEX_POINT ( 'NONE', #7815 ) ;
#4716=DIRECTION ( 'NONE',  ( 0.000000000000000000, 0.000000000000000000, -1.000000000000000000 ) ) ;
#4721=AXIS2_PLACEMENT_3D ( 'NONE', #4476, #11617, #20641 ) ;
#4724=DIRECTION ( 'NONE',  ( -1.000000000000000000, 0.000000000000000000, 0.000000000000000000 ) ) ;
#4725=AXIS2_PLACEMENT_3D ( 'NONE', #1586, #21168, #1466 ) ;
#4727=CARTESIAN_POINT ( 'NONE',  ( 142.2098376044692714, -3658.165498732453216, 2249.440698602000793 ) ) ;
#4728=CARTESIAN_POINT ( 'NONE',  ( 18.41499991942999870, -3579.495498070999474, 2244.618783703000190 ) ) ;
#4730=EDGE_LOOP ( 'NONE', ( #17184, #2219, #1973, #1560 ) ) ;
#4733=CARTESIAN_POINT ( 'NONE',  ( 4.767598319208563140, -3695.602652332028356, 2259.817658126045899 ) ) ;
#4734=VECTOR ( 'NONE', #22632, 1000.000000000000000 ) ;
#4736=ORIENTED_EDGE ( 'NONE', *, *, #4067, .T. ) ;
#4741=DIRECTION ( 'NONE',  ( 0.6887494619146540265, 0.000000000000000000, -0.7249994335944508483 ) ) ;
#4747=CARTESIAN_POINT ( 'NONE',  ( 17.79584664100706703, -3576.912150935504087, 2245.312549109999054 ) ) ;
#4748=CARTESIAN_POINT ( 'NONE',  ( 20.56205275154204415, -3695.513274360283958, 2259.993648869947265 ) ) ;
#4749=ORIENTED_EDGE ( 'NONE', *, *, #16887, .F. ) ;
#4754=CARTESIAN_POINT ( 'NONE',  ( 10.90284348872566333, -3581.700236517450776, 2247.212196148407202 ) ) ;
#4759=AXIS2_PLACEMENT_3D ( 'NONE', #10760, #1854, #8998 ) ;
#4763=FACE_OUTER_BOUND ( 'NONE', #18761, .T. ) ;
#4766=ORIENTED_EDGE ( 'NONE', *, *, #2958, .T. ) ;
#4774=ORIENTED_EDGE ( 'NONE', *, *, #5980, .F. ) ;
#4775=VERTEX_POINT ( 'NONE', #21876 ) ;
#4777=EDGE_CURVE ( 'NONE', #14341, #6224, #17984, .T. ) ;
#4778=CARTESIAN_POINT ( 'NONE',  ( 114.2999999999999972, -3644.899999999999636, 2239.771999999999935 ) ) ;
#4780=ORIENTED_EDGE ( 'NONE', *, *, #1169, .F. ) ;
#4785=DIRECTION ( 'NONE',  ( -1.000000000000000000, 0.000000000000000000, 0.000000000000000000 ) ) ;
#4786=DIRECTION ( 'NONE',  ( 0.000000000000000000, 0.000000000000000000, -1.000000000000000000 ) ) ;
#4787=CARTESIAN_POINT ( 'NONE',  ( 131.5729205195000020, -3695.699999999999818, 2259.329999999999927 ) ) ;
#4788=DIRECTION ( 'NONE',  ( 0.000000000000000000, 0.000000000000000000, -1.000000000000000000 ) ) ;
#4789=AXIS2_PLACEMENT_3D ( 'NONE', #8016, #8241, #11874 ) ;
#4793=CARTESIAN_POINT ( 'NONE',  ( 35.56000000000000227, -3544.570000000000164, 2247.392000000000280 ) ) ;
#4794=ORIENTED_EDGE ( 'NONE', *, *, #3134, .T. ) ;
#4795=DIRECTION ( 'NONE',  ( 0.000000000000000000, 0.000000000000000000, 1.000000000000000000 ) ) ;
#4796=CARTESIAN_POINT ( 'NONE',  ( 10.28963435466927834, -3657.994130827179561, 2249.259658297236001 ) ) ;
#4797=EDGE_CURVE ( 'NONE', #7082, #4608, #16849, .T. ) ;
#4798=ORIENTED_EDGE ( 'NONE', *, *, #5704, .T. ) ;
#4800=DIRECTION ( 'NONE',  ( 0.000000000000000000, 0.000000000000000000, 1.000000000000000000 ) ) ;
#4801=ORIENTED_EDGE ( 'NONE', *, *, #19684, .T. ) ;
#4802=DIRECTION ( 'NONE',  ( 0.000000000000000000, -1.000000000000000000, 0.000000000000000000 ) ) ;
#4804=FACE_OUTER_BOUND ( 'NONE', #20439, .T. ) ;
#4805=EDGE_LOOP ( 'NONE', ( #17235, #2738 ) ) ;
#4806=CARTESIAN_POINT ( 'NONE',  ( 131.8914011584156469, -3695.418298523433350, 2260.127650043255471 ) ) ;
#4808=ADVANCED_FACE ( 'NONE', ( #12744 ), #19900, .F. ) ;
#4810=CARTESIAN_POINT ( 'NONE',  ( 151.4000000000000057, -3695.670967364599164, 2259.329999999999927 ) ) ;
#4811=CARTESIAN_POINT ( 'NONE',  ( 59.89320000000000022, -3594.099999999999909, 2259.837999999999738 ) ) ;
#4815=EDGE_LOOP ( 'NONE', ( #2450, #16060, #21882, #9635 ) ) ;
#4816=AXIS2_PLACEMENT_3D ( 'NONE', #22570, #17181, #11918 ) ;
#4818=CARTESIAN_POINT ( 'NONE',  ( 12.69999999999999929, -3659.504999999999654, 2239.771999999999935 ) ) ;
#4821=CARTESIAN_POINT ( 'NONE',  ( 20.59150420445999785, -3544.527728344000025, 2260.600000000000364 ) ) ;
#4825=LINE ( 'NONE', #22630, #11449 ) ;
#4827=CARTESIAN_POINT ( 'NONE',  ( 53.64479999999999649, -3568.700000000000273, 2261.869999999999891 ) ) ;
#4830=DIRECTION ( 'NONE',  ( -0.000000000000000000, -1.000000000000000000, -0.000000000000000000 ) ) ;
#4831=CARTESIAN_POINT ( 'NONE',  ( 21.79320000000099711, -3670.300000000000182, 2259.837999999999738 ) ) ;
#4832=FACE_OUTER_BOUND ( 'NONE', #2346, .T. ) ;
#4835=CARTESIAN_POINT ( 'NONE',  ( 141.6735277291679154, -3657.455622841492641, 2248.335144904084700 ) ) ;
#4838=ORIENTED_EDGE ( 'NONE', *, *, #17606, .T. ) ;
#4839=CARTESIAN_POINT ( 'NONE',  ( 136.8553092860665856, -3543.405519448711857, 2255.010836426657079 ) ) ;
#4840=EDGE_CURVE ( 'NONE', #21716, #14725, #15327, .T. ) ;
#4842=DIRECTION ( 'NONE',  ( 0.000000000000000000, 0.000000000000000000, -1.000000000000000000 ) ) ;
#4845=ORIENTED_EDGE ( 'NONE', *, *, #8095, .T. ) ;
#4848=CARTESIAN_POINT ( 'NONE',  ( 4.707879222708684530, -3543.344914980570593, 2259.667286593787139 ) ) ;
#4849=DIRECTION ( 'NONE',  ( -1.000000000000000000, 0.000000000000000000, 0.000000000000000000 ) ) ;
#4850=CIRCLE ( 'NONE', #8592, 2.844800000000091700 ) ;
#4851=CARTESIAN_POINT ( 'NONE',  ( 131.7757523116999891, -3694.430000000000291, 2260.600000000000364 ) ) ;
#4852=EDGE_CURVE ( 'NONE', #15774, #1541, #1089, .T. ) ;
#4856=CARTESIAN_POINT ( 'NONE',  ( 95.25000000000031264, -3568.700000000000273, 2250.236800000000130 ) ) ;
#4858=CARTESIAN_POINT ( 'NONE',  ( 151.4000000000000057, -3695.699999999999818, 2260.570967364599255 ) ) ;
#4859=CARTESIAN_POINT ( 'NONE',  ( 142.5448000000000093, -3659.504999999999654, 2256.063560000000052 ) ) ;
#4860=ORIENTED_EDGE ( 'NONE', *, *, #1417, .T. ) ;
#4864=ORIENTED_EDGE ( 'NONE', *, *, #11251, .F. ) ;
#4865=DIRECTION ( 'NONE',  ( 1.000000000000000000, 0.000000000000000000, 0.000000000000000000 ) ) ;
#4874=CARTESIAN_POINT ( 'NONE',  ( 144.9127847416437191, -3661.847664638717106, 2245.116748441303116 ) ) ;
#4875=DIRECTION ( 'NONE',  ( 0.000000000000000000, 0.000000000000000000, 1.000000000000000000 ) ) ;
#4876=CARTESIAN_POINT ( 'NONE',  ( 11.92076576356236295, -3662.241062566742585, 2249.309941814265585 ) ) ;
#4878=EDGE_LOOP ( 'NONE', ( #18927, #13957 ) ) ;
#4884=CARTESIAN_POINT ( 'NONE',  ( 116.8400000000000034, -3544.570000000000164, 2250.236800000000130 ) ) ;
#4895=CIRCLE ( 'NONE', #10518, 2.844800000000001550 ) ;
#4897=DIRECTION ( 'NONE',  ( 0.000000000000000000, 0.000000000000000000, 1.000000000000000000 ) ) ;
#4904=VERTEX_POINT ( 'NONE', #7927 ) ;
#4906=LINE ( 'NONE', #15693, #10700 ) ;
#4908=DIRECTION ( 'NONE',  ( 0.000000000000000000, 0.000000000000000000, -1.000000000000000000 ) ) ;
#4909=EDGE_LOOP ( 'NONE', ( #11353, #10116, #19494, #15122 ) ) ;
#4910=EDGE_CURVE ( 'NONE', #21090, #13352, #19056, .T. ) ;
#4912=CARTESIAN_POINT ( 'NONE',  ( 147.3321676912462124, -3694.709202396953970, 2260.569587683029113 ) ) ;
#4914=ORIENTED_EDGE ( 'NONE', *, *, #22442, .F. ) ;
#4915=AXIS2_PLACEMENT_3D ( 'NONE', #18542, #6364, #16782 ) ;
#4917=DIRECTION ( 'NONE',  ( 0.000000000000000000, 0.000000000000000000, -1.000000000000000000 ) ) ;
#4926=CARTESIAN_POINT ( 'NONE',  ( 14.94291645695195925, -3581.245342914359753, 2248.943312577677716 ) ) ;
#4928=CARTESIAN_POINT ( 'NONE',  ( 134.0255062626791869, -3658.825944694054215, 2244.868864689911788 ) ) ;
#4930=FACE_OUTER_BOUND ( 'NONE', #5659, .T. ) ;
#4931=ORIENTED_EDGE ( 'NONE', *, *, #4371, .T. ) ;
#4933=EDGE_CURVE ( 'NONE', #4608, #12839, #14213, .T. ) ;
#4935=ORIENTED_EDGE ( 'NONE', *, *, #4797, .T. ) ;
#4937=EDGE_CURVE ( 'NONE', #22994, #12111, #7751, .T. ) ;
#4940=VERTEX_POINT ( 'NONE', #22206 ) ;
#4941=FACE_OUTER_BOUND ( 'NONE', #23065, .T. ) ;
#4943=CARTESIAN_POINT ( 'NONE',  ( 133.9850000806000310, -3659.610054942478655, 2244.594903130879629 ) ) ;
#4944=AXIS2_PLACEMENT_3D ( 'NONE', #14913, #1023, #13573 ) ;
#4946=CIRCLE ( 'NONE', #16176, 2.844800000000001550 ) ;
#4948=CARTESIAN_POINT ( 'NONE',  ( 15.47291618100999955, -3660.140271294999820, 2250.236802488000194 ) ) ;
#4952=CARTESIAN_POINT ( 'NONE',  ( 9.855390812759999619, -3579.528596999999991, 2250.157115725000040 ) ) ;
#4953=DIRECTION ( 'NONE',  ( -1.000000000000000000, 0.000000000000000000, 0.000000000000000000 ) ) ;
#4957=CARTESIAN_POINT ( 'NONE',  ( 141.8180919227771994, -3657.605902934063579, 2248.684766514065359 ) ) ;
#4958=CIRCLE ( 'NONE', #3079, 0.7619999999999294005 ) ;
#4960=TOROIDAL_SURFACE ( 'NONE', #3841, 4.114799999999999791, 1.270000000000000018 ) ;
#4961=CARTESIAN_POINT ( 'NONE',  ( 35.25520000000000209, -3644.899999999999636, 2259.837999999999738 ) ) ;
#4967=ORIENTED_EDGE ( 'NONE', *, *, #7445, .T. ) ;
#4970=DIRECTION ( 'NONE',  ( 0.7249994335944036639, 0.000000000000000000, 0.6887494619147036534 ) ) ;
#4971=AXIS2_PLACEMENT_3D ( 'NONE', #11295, #637, #4381 ) ;
#4974=ORIENTED_EDGE ( 'NONE', *, *, #3409, .T. ) ;
#4981=ORIENTED_EDGE ( 'NONE', *, *, #8301, .T. ) ;
#4983=AXIS2_PLACEMENT_3D ( 'NONE', #14956, #6166, #11097 ) ;
#4984=EDGE_LOOP ( 'NONE', ( #3439, #3907, #19440, #13566, #2737, #13587, #4396, #10941, #11277, #7859 ) ) ;
#4985=CARTESIAN_POINT ( 'NONE',  ( 50.79999999999999716, -3619.500000000000000, 2239.771999999999935 ) ) ;
#4987=EDGE_CURVE ( 'NONE', #10571, #473, #17186, .T. ) ;
#4989=CARTESIAN_POINT ( 'NONE',  ( 10.31443137789909237, -3581.044692580274841, 2249.214089242949285 ) ) ;
#4990=ORIENTED_EDGE ( 'NONE', *, *, #18452, .T. ) ;
#4991=DIRECTION ( 'NONE',  ( 0.000000000000000000, 0.000000000000000000, -1.000000000000000000 ) ) ;
#4995=FACE_BOUND ( 'NONE', #15659, .T. ) ;
#4996=EDGE_CURVE ( 'NONE', #10545, #1677, #11566, .T. ) ;
#4998=CARTESIAN_POINT ( 'NONE',  ( 20.09942059832000183, -3694.430000000000291, 2260.390449568000349 ) ) ;
#5000=TOROIDAL_SURFACE ( 'NONE', #15857, 3.606799999998999695, 0.7620000000000000107 ) ;
#5001=DIRECTION ( 'NONE',  ( 0.000000000000000000, 0.000000000000000000, 1.000000000000000000 ) ) ;
#5002=CARTESIAN_POINT ( 'NONE',  ( 11.29225843401678198, -3661.977178471061961, 2249.564116967847440 ) ) ;
#5004=CARTESIAN_POINT ( 'NONE',  ( 147.5484590635937820, -3543.507962131723616, 2260.027583316409618 ) ) ;
#5010=CARTESIAN_POINT ( 'NONE',  ( 14.95049008878873131, -3657.764820619780494, 2248.957728567762842 ) ) ;
#5011=LINE ( 'NONE', #12153, #12811 ) ;
#5013=CIRCLE ( 'NONE', #15850, 3.606799999999993567 ) ;
#5014=ORIENTED_EDGE ( 'NONE', *, *, #13406, .F. ) ;
#5015=EDGE_LOOP ( 'NONE', ( #8119, #1278, #899, #5458 ) ) ;
#5022=CARTESIAN_POINT ( 'NONE',  ( 132.3005794017000198, -3694.430000000000291, 2260.390449568000349 ) ) ;
#5024=DIRECTION ( 'NONE',  ( -1.000000000000000000, 0.000000000000000000, 0.000000000000000000 ) ) ;
#5026=DIRECTION ( 'NONE',  ( 0.000000000000000000, 0.000000000000000000, 1.000000000000000000 ) ) ;
#5028=TOROIDAL_SURFACE ( 'NONE', #20006, 3.606799999999999784, 0.7620000000000000107 ) ;
#5029=DIRECTION ( 'NONE',  ( -0.7249994335945011414, 0.000000000000000000, -0.6887494619146010688 ) ) ;
#5030=DIRECTION ( 'NONE',  ( 0.000000000000000000, 0.000000000000000000, 1.000000000000000000 ) ) ;
#5031=AXIS2_PLACEMENT_3D ( 'NONE', #195, #18114, #11090 ) ;
#5033=DIRECTION ( 'NONE',  ( 1.000000000000000000, 0.000000000000000000, 0.000000000000000000 ) ) ;
#5034=CARTESIAN_POINT ( 'NONE',  ( 10.58528415310206938, -3657.602126776196656, 2248.677371791971382 ) ) ;
#5036=CARTESIAN_POINT ( 'NONE',  ( 132.2269032045000188, -3694.556024844999683, 2260.454626673999883 ) ) ;
#5037=ORIENTED_EDGE ( 'NONE', *, *, #21895, .T. ) ;
#5039=DIRECTION ( 'NONE',  ( 0.000000000000000000, -1.000000000000000000, 0.000000000000000000 ) ) ;
#5041=CARTESIAN_POINT ( 'NONE',  ( 136.8551999999999964, -3579.495007806000103, 2250.165025852999861 ) ) ;
#5043=CARTESIAN_POINT ( 'NONE',  ( 131.6470296295221090, -3695.700000000016189, 2259.515609107377259 ) ) ;
#5044=CIRCLE ( 'NONE', #3919, 0.7619999999999987894 ) ;
#5046=AXIS2_PLACEMENT_3D ( 'NONE', #18, #1883, #7167 ) ;
#5047=CIRCLE ( 'NONE', #13262, 3.606799999999993567 ) ;
#5050=CARTESIAN_POINT ( 'NONE',  ( 134.1731578100668401, -3658.050678563296970, 2245.461022134579252 ) ) ;
#5054=DIRECTION ( 'NONE',  ( 1.000000000000000000, 0.000000000000000000, 0.000000000000000000 ) ) ;
#5055=ORIENTED_EDGE ( 'NONE', *, *, #15049, .F. ) ;
#5059=CIRCLE ( 'NONE', #17386, 2.844800000000094364 ) ;
#5060=CARTESIAN_POINT ( 'NONE',  ( 86.05520000000001346, -3594.099999999999909, 2239.771999999999935 ) ) ;
#5061=CIRCLE ( 'NONE', #16661, 2.844800000000091700 ) ;
#5062=ORIENTED_EDGE ( 'NONE', *, *, #19543, .T. ) ;
#5064=FACE_OUTER_BOUND ( 'NONE', #15399, .T. ) ;
#5066=ORIENTED_EDGE ( 'NONE', *, *, #10438, .F. ) ;
#5068=CARTESIAN_POINT ( 'NONE',  ( 139.6999999999999886, -3659.504999999999654, 2246.630000000000109 ) ) ;
#5069=CYLINDRICAL_SURFACE ( 'NONE', #20591, 5.715000000000999947 ) ;
#5070=DIRECTION ( 'NONE',  ( 0.000000000000000000, 0.000000000000000000, -1.000000000000000000 ) ) ;
#5071=FACE_OUTER_BOUND ( 'NONE', #5776, .T. ) ;
#5073=EDGE_CURVE ( 'NONE', #7277, #473, #2591, .T. ) ;
#5075=CARTESIAN_POINT ( 'NONE',  ( 35.56000000000000227, -3543.300000000000182, 2243.277199999999993 ) ) ;
#5077=ADVANCED_FACE ( 'NONE', ( #15889 ), #17875, .F. ) ;
#5079=AXIS2_PLACEMENT_3D ( 'NONE', #4077, #16608, #14865 ) ;
#5081=EDGE_CURVE ( 'NONE', #18860, #6059, #4100, .T. ) ;
#5082=CARTESIAN_POINT ( 'NONE',  ( 141.5504581569688298, -3657.343157095971037, 2247.943075285883879 ) ) ;
#5084=VERTEX_POINT ( 'NONE', #5113 ) ;
#5086=DIRECTION ( 'NONE',  ( 0.000000000000000000, 0.000000000000000000, -1.000000000000000000 ) ) ;
#5090=VERTEX_POINT ( 'NONE', #1349 ) ;
#5093=ORIENTED_EDGE ( 'NONE', *, *, #14142, .T. ) ;
#5094=CARTESIAN_POINT ( 'NONE',  ( 4.769683475340658951, -3543.399485435076713, 2259.822725891639948 ) ) ;
#5095=ADVANCED_FACE ( 'NONE', ( #17754 ), #12739, .T. ) ;
#5097=CARTESIAN_POINT ( 'NONE',  ( 95.25000000000000000, -3694.430000000000291, 2247.392000000000280 ) ) ;
#5099=CARTESIAN_POINT ( 'NONE',  ( 127.0000000000000000, -3670.300000000000182, 2261.869999999999891 ) ) ;
#5108=EDGE_LOOP ( 'NONE', ( #14151, #8117 ) ) ;
#5110=FACE_OUTER_BOUND ( 'NONE', #4572, .T. ) ;
#5112=CARTESIAN_POINT ( 'NONE',  ( 10.55027246081846215, -3581.358398341555585, 2248.752751047937636 ) ) ;
#5113=CARTESIAN_POINT ( 'NONE',  ( 97.99320000000000164, -3670.300000000000182, 2260.600000000000364 ) ) ;
#5114=ORIENTED_EDGE ( 'NONE', *, *, #14409, .T. ) ;
#5115=CARTESIAN_POINT ( 'NONE',  ( 57.14999999999999858, -3670.300000000000182, 2250.236800000000130 ) ) ;
#5116=ADVANCED_FACE ( 'NONE', ( #23132 ), #12485, .T. ) ;
#5117=CIRCLE ( 'NONE', #20815, 0.7619999999999294005 ) ;
#5118=EDGE_CURVE ( 'NONE', #9059, #10931, #10828, .T. ) ;
#5119=ADVANCED_FACE ( 'NONE', ( #21512 ), #5463, .F. ) ;
#5123=AXIS2_PLACEMENT_3D ( 'NONE', #21633, #12835, #413 ) ;
#5124=CARTESIAN_POINT ( 'NONE',  ( 10.70420337415141887, -3661.532743059901350, 2249.872907817715713 ) ) ;
#5125=ORIENTED_EDGE ( 'NONE', *, *, #1353, .T. ) ;
#5130=CYLINDRICAL_SURFACE ( 'NONE', #4816, 2.844799999999994444 ) ;
#5131=CARTESIAN_POINT ( 'NONE',  ( 14.82996365613828260, -3657.619199960707647, 2248.710555545362240 ) ) ;
#5133=CIRCLE ( 'NONE', #10407, 1.269999999999882334 ) ;
#5138=CARTESIAN_POINT ( 'NONE',  ( 110.6932000000009992, -3594.099999999999909, 2239.771999999999935 ) ) ;
#5139=VECTOR ( 'NONE', #17197, 1000.000000000000000 ) ;
#5142=AXIS2_PLACEMENT_3D ( 'NONE', #10847, #18107, #14718 ) ;
#5145=CARTESIAN_POINT ( 'NONE',  ( 127.0000000000000000, -3619.500000000000000, 2259.837999999999738 ) ) ;
#5146=EDGE_CURVE ( 'NONE', #10072, #22625, #16130, .T. ) ;
#5148=EDGE_CURVE ( 'NONE', #20964, #7890, #2181, .T. ) ;
#5152=DIRECTION ( 'NONE',  ( 0.000000000000000000, 0.000000000000000000, -1.000000000000000000 ) ) ;
#5153=CIRCLE ( 'NONE', #8140, 0.7619999999999987894 ) ;
#5157=CARTESIAN_POINT ( 'NONE',  ( 4.572920519510000226, -3543.299999999999727, 2259.329999999999927 ) ) ;
#5159=ORIENTED_EDGE ( 'NONE', *, *, #12145, .T. ) ;
#5160=CARTESIAN_POINT ( 'NONE',  ( 134.3755117000944210, -3581.571545880567555, 2246.524605944011000 ) ) ;
#5162=EDGE_CURVE ( 'NONE', #553, #17865, #5175, .T. ) ;
#5163=VERTEX_POINT ( 'NONE', #18445 ) ;
#5164=CARTESIAN_POINT ( 'NONE',  ( 139.6999999999999886, -3659.504999999999654, 2246.630000000000109 ) ) ;
#5167=DIRECTION ( 'NONE',  ( -1.000000000000000000, 0.000000000000000000, 0.000000000000000000 ) ) ;
#5168=VERTEX_POINT ( 'NONE', #9538 ) ;
#5173=CARTESIAN_POINT ( 'NONE',  ( 14.91976558997560431, -3581.274556505038163, 2248.897383337483916 ) ) ;
#5175=CIRCLE ( 'NONE', #4045, 2.844799999998995244 ) ;
#5177=DIRECTION ( 'NONE',  ( -1.000000000000000000, 0.000000000000000000, 0.000000000000000000 ) ) ;
#5178=ORIENTED_EDGE ( 'NONE', *, *, #12435, .T. ) ;
#5179=CARTESIAN_POINT ( 'NONE',  ( 15.40196735877819734, -3695.360820976567993, 2255.368368629970519 ) ) ;
#5181=ORIENTED_EDGE ( 'NONE', *, *, #13966, .F. ) ;
#5183=AXIS2_PLACEMENT_3D ( 'NONE', #10694, #22867, #17717 ) ;
#5185=EDGE_LOOP ( 'NONE', ( #3720, #8055, #19612, #11085 ) ) ;
#5188=DIRECTION ( 'NONE',  ( 0.000000000000000000, 1.000000000000000000, 0.000000000000000000 ) ) ;
#5189=CYLINDRICAL_SURFACE ( 'NONE', #14418, 2.844800000000091700 ) ;
#5191=FACE_OUTER_BOUND ( 'NONE', #2439, .T. ) ;
#5195=CARTESIAN_POINT ( 'NONE',  ( 25.39999999999999858, -3670.300000000000182, 2239.771999999999935 ) ) ;
#5198=CARTESIAN_POINT ( 'NONE',  ( 137.3031193615345558, -3657.972810158548327, 2249.234928345508706 ) ) ;
#5199=EDGE_LOOP ( 'NONE', ( #4864, #4698, #4588, #13448 ) ) ;
#5200=VECTOR ( 'NONE', #10827, 1000.000000000000000 ) ;
#5201=CARTESIAN_POINT ( 'NONE',  ( 134.0203227398999957, -3578.860230781999689, 2244.548186305999934 ) ) ;
#5203=EDGE_CURVE ( 'NONE', #8201, #19707, #20872, .T. ) ;
#5208=EDGE_CURVE ( 'NONE', #22764, #20229, #18258, .T. ) ;
#5210=ORIENTED_EDGE ( 'NONE', *, *, #16807, .T. ) ;
#5211=CARTESIAN_POINT ( 'NONE',  ( 5.079999999832377711, -3544.253380988285699, 2260.599999999823467 ) ) ;
#5212=EDGE_CURVE ( 'NONE', #4163, #15095, #22067, .T. ) ;
#5214=CYLINDRICAL_SURFACE ( 'NONE', #12540, 1.269999999999882334 ) ;
#5219=DIRECTION ( 'NONE',  ( 0.000000000000000000, 1.000000000000000000, 0.000000000000000000 ) ) ;
#5220=DIRECTION ( 'NONE',  ( 0.000000000000000000, 0.000000000000000000, -1.000000000000000000 ) ) ;
#5223=VERTEX_POINT ( 'NONE', #2055 ) ;
#5225=EDGE_CURVE ( 'NONE', #13878, #18081, #9644, .T. ) ;
#5226=CARTESIAN_POINT ( 'NONE',  ( 131.8914032746874341, -3543.581701476120543, 2260.127649197567735 ) ) ;
#5227=CARTESIAN_POINT ( 'NONE',  ( 10.82796438153653007, -3581.637321854239872, 2248.014231754040338 ) ) ;
#5230=EDGE_LOOP ( 'NONE', ( #15752, #18091, #17816, #17255 ) ) ;
#5233=FACE_BOUND ( 'NONE', #21994, .T. ) ;
#5234=DIRECTION ( 'NONE',  ( 0.000000000000000000, 1.000000000000000000, 0.000000000000000000 ) ) ;
#5235=CARTESIAN_POINT ( 'NONE',  ( 10.60701338793428050, -3661.431926821307570, 2249.926631412048664 ) ) ;
#5236=CARTESIAN_POINT ( 'NONE',  ( 88.90000000000000568, -3594.099999999999909, 2239.771999999999935 ) ) ;
#5237=EDGE_LOOP ( 'NONE', ( #2360, #21059 ) ) ;
#5242=DIRECTION ( 'NONE',  ( -1.000000000000000000, 0.000000000000000000, 0.000000000000000000 ) ) ;
#5243=CARTESIAN_POINT ( 'NONE',  ( 15.08392934718898459, -3657.952714460870993, 2249.210978331739170 ) ) ;
#5244=CARTESIAN_POINT ( 'NONE',  ( 137.1599999999999966, -3694.430000000000291, 2255.774000000000342 ) ) ;
#5246=CYLINDRICAL_SURFACE ( 'NONE', #1899, 2.844800000000091700 ) ;
#5248=CARTESIAN_POINT ( 'NONE',  ( 132.0879339926999876, -3544.241663918999620, 2260.533847755999886 ) ) ;
#5250=DIRECTION ( 'NONE',  ( 0.000000000000000000, 0.000000000000000000, -1.000000000000000000 ) ) ;
#5253=DIRECTION ( 'NONE',  ( 0.000000000000000000, 0.000000000000000000, -1.000000000000000000 ) ) ;
#5258=ORIENTED_EDGE ( 'NONE', *, *, #13572, .F. ) ;
#5259=AXIS2_PLACEMENT_3D ( 'NONE', #22813, #10869, #5498 ) ;
#5260=CARTESIAN_POINT ( 'NONE',  ( 151.1299999999999955, -3544.570000000000164, 2260.600000000000364 ) ) ;
#5263=FACE_OUTER_BOUND ( 'NONE', #5230, .T. ) ;
#5266=CARTESIAN_POINT ( 'NONE',  ( 35.56000000000000227, -3694.430000000000291, 2250.236800000000130 ) ) ;
#5267=DIRECTION ( 'NONE',  ( 1.000000000000000000, 0.000000000000000000, 0.000000000000000000 ) ) ;
#5268=ORIENTED_EDGE ( 'NONE', *, *, #8131, .T. ) ;
#5272=EDGE_CURVE ( 'NONE', #1840, #6749, #22405, .T. ) ;
#5273=CARTESIAN_POINT ( 'NONE',  ( 15.44319999999931525, -3580.373257047475363, 2255.967040000000907 ) ) ;
#5274=ORIENTED_EDGE ( 'NONE', *, *, #620, .F. ) ;
#5275=DIRECTION ( 'NONE',  ( 0.000000000000000000, 0.000000000000000000, -1.000000000000000000 ) ) ;
#5278=DIRECTION ( 'NONE',  ( 0.000000000000000000, 0.000000000000000000, -1.000000000000000000 ) ) ;
#5280=CARTESIAN_POINT ( 'NONE',  ( 6.985000002048999512, -3579.494756921999851, 2244.617465693000213 ) ) ;
#5281=ADVANCED_FACE ( 'NONE', ( #9760 ), #11522, .F. ) ;
#5283=DIRECTION ( 'NONE',  ( 0.000000000000000000, 0.000000000000000000, 1.000000000000000000 ) ) ;
#5284=CARTESIAN_POINT ( 'NONE',  ( 101.5999999999999943, -3619.500000000000000, 2239.771999999999935 ) ) ;
#5286=ORIENTED_EDGE ( 'NONE', *, *, #19519, .F. ) ;
#5288=EDGE_CURVE ( 'NONE', #12668, #22201, #19012, .T. ) ;
#5289=VECTOR ( 'NONE', #20912, 1000.000000000000000 ) ;
#5290=ADVANCED_FACE ( 'NONE', ( #8243 ), #19763, .T. ) ;
#5293=CARTESIAN_POINT ( 'NONE',  ( 38.10000000000000142, -3594.099999999999909, 2239.771999999999935 ) ) ;
#5294=LINE ( 'NONE', #19586, #1629 ) ;
#5297=ORIENTED_EDGE ( 'NONE', *, *, #2510, .F. ) ;
#5299=CARTESIAN_POINT ( 'NONE',  ( 1.270000000000000018, -3695.699999999999818, 2259.329999999999927 ) ) ;
#5300=VERTEX_POINT ( 'NONE', #11406 ) ;
#5310=CARTESIAN_POINT ( 'NONE',  ( 9.847653496145797547, -3695.602652332805974, 2254.991636092922818 ) ) ;
#5313=CARTESIAN_POINT ( 'NONE',  ( 137.4007074334733716, -3657.828996996126989, 2249.052647309616987 ) ) ;
#5314=VERTEX_POINT ( 'NONE', #4728 ) ;
#5316=ORIENTED_EDGE ( 'NONE', *, *, #10557, .T. ) ;
#5318=ORIENTED_EDGE ( 'NONE', *, *, #11923, .F. ) ;
#5321=CARTESIAN_POINT ( 'NONE',  ( 151.1299999999999955, -3660.140000000000327, 2247.392000000000280 ) ) ;
#5322=ORIENTED_EDGE ( 'NONE', *, *, #9676, .T. ) ;
#5323=EDGE_LOOP ( 'NONE', ( #6809, #8816, #22785, #11701 ) ) ;
#5324=CARTESIAN_POINT ( 'NONE',  ( 4.722881977098646544, -3543.356150277230427, 2259.705006069447791 ) ) ;
#5326=DIRECTION ( 'NONE',  ( 0.000000000000000000, 0.000000000000000000, -1.000000000000000000 ) ) ;
#5330=FACE_BOUND ( 'NONE', #14463, .T. ) ;
#5338=DIRECTION ( 'NONE',  ( 0.7249994335945011414, 0.000000000000000000, 0.6887494619146010688 ) ) ;
#5339=AXIS2_PLACEMENT_3D ( 'NONE', #6547, #13919, #14162 ) ;
#5343=ADVANCED_FACE ( 'NONE', ( #15393 ), #5552, .T. ) ;
#5346=FACE_BOUND ( 'NONE', #18764, .T. ) ;
#5347=EDGE_CURVE ( 'NONE', #7639, #22341, #7413, .T. ) ;
#5349=CARTESIAN_POINT ( 'NONE',  ( 63.50000000000000000, -3644.899999999999636, 2239.771999999999935 ) ) ;
#5350=DIRECTION ( 'NONE',  ( 0.000000000000000000, 0.000000000000000000, -1.000000000000000000 ) ) ;
#5351=AXIS2_PLACEMENT_3D ( 'NONE', #14796, #16430, #610 ) ;
#5354=CARTESIAN_POINT ( 'NONE',  ( 147.3359348846743444, -3544.251379750038723, 2260.560039348503324 ) ) ;
#5355=VERTEX_POINT ( 'NONE', #6269 ) ;
#5358=CARTESIAN_POINT ( 'NONE',  ( 132.0583097651000060, -3694.797466901999996, 2260.545675974999995 ) ) ;
#5361=CARTESIAN_POINT ( 'NONE',  ( 15.01743630476217284, -3657.855092720787525, 2249.086948850284443 ) ) ;
#5362=CARTESIAN_POINT ( 'NONE',  ( 137.1478323087536637, -3694.709202396637011, 2255.743587683099577 ) ) ;
#5366=AXIS2_PLACEMENT_3D ( 'NONE', #15878, #14009, #17509 ) ;
#5370=AXIS2_PLACEMENT_3D ( 'NONE', #11688, #11575, #6559 ) ;
#5374=CARTESIAN_POINT ( 'NONE',  ( 34.49320000000000164, -3644.899999999999636, 2259.837999999999738 ) ) ;
#5376=DIRECTION ( 'NONE',  ( -1.000000000000000000, 0.000000000000000000, 0.000000000000000000 ) ) ;
#5378=CIRCLE ( 'NONE', #12481, 2.844799999998995244 ) ;
#5379=B_SPLINE_CURVE_WITH_KNOTS ( 'NONE', 3,
 ( #5244, #8760, #23038, #5362, #7351, #2079, #7013, #84, #9225, #14158, #318, #9110, #21301, #3473, #3821, #14503, #7236, #16365, #16248, #21646, #12386, #16021, #10625, #14382, #10975, #21414, #17771, #1727, #8877, #23147, #12625 ),
 .UNSPECIFIED., .F., .F.,
 ( 4, 2, 2, 2, 2, 2, 1, 2, 2, 2, 2, 1, 1, 2, 2, 2, 4 ),
 ( 0.000000000000000000, 0.1250000000013097856, 0.1875000000023017976, 0.2500000000032938097, 0.3750000000052778337, 0.4375000000059938166, 0.4687500000061067262, 0.4843750000063656858, 0.5000000000066245898, 0.6250000000102919895, 0.6875000000121920252, 0.7187500000131421540, 0.7343750000137396761, 0.7421875000141466838, 0.7500000000145535806, 0.8750000000072767348, 1.000000000000000000 ),
 .UNSPECIFIED. ) ;
#5382=ORIENTED_EDGE ( 'NONE', *, *, #9456, .T. ) ;
#5383=DIRECTION ( 'NONE',  ( 1.000000000000000000, -0.000000000000000000, 1.224646799147353207E-16 ) ) ;
#5385=VERTEX_POINT ( 'NONE', #17574 ) ;
#5386=LINE ( 'NONE', #10646, #558 ) ;
#5388=ORIENTED_EDGE ( 'NONE', *, *, #11492, .T. ) ;
#5391=EDGE_CURVE ( 'NONE', #17185, #9415, #20147, .T. ) ;
#5393=CARTESIAN_POINT ( 'NONE',  ( 137.3991818876238540, -3581.168941546183760, 2249.055578352219072 ) ) ;
#5394=ORIENTED_EDGE ( 'NONE', *, *, #115, .F. ) ;
#5397=DIRECTION ( 'NONE',  ( 0.000000000000000000, 0.000000000000000000, -1.000000000000000000 ) ) ;
#5398=DIRECTION ( 'NONE',  ( 0.000000000000000000, 0.000000000000000000, -1.000000000000000000 ) ) ;
#5402=DIRECTION ( 'NONE',  ( 0.000000000000000000, 1.000000000000000000, 0.000000000000000000 ) ) ;
#5403=DIRECTION ( 'NONE',  ( -1.000000000000000000, 0.000000000000000000, 0.000000000000000000 ) ) ;
#5405=CARTESIAN_POINT ( 'NONE',  ( 134.0238507593082034, -3578.829296296447410, 2244.547341334188332 ) ) ;
#5407=EDGE_CURVE ( 'NONE', #18712, #3088, #2126, .T. ) ;
#5408=DIRECTION ( 'NONE',  ( 0.000000000000000000, 0.000000000000000000, 1.000000000000000000 ) ) ;
#5411=CARTESIAN_POINT ( 'NONE',  ( 136.8552000000001669, -3659.053785370567766, 2256.063560000000052 ) ) ;
#5413=EDGE_LOOP ( 'NONE', ( #21957, #494, #10092, #20125 ) ) ;
#5414=CARTESIAN_POINT ( 'NONE',  ( 139.6999999999999886, -3579.494999999999891, 2246.630000000000109 ) ) ;
#5424=EDGE_CURVE ( 'NONE', #14745, #20703, #8911, .T. ) ;
#5426=DIRECTION ( 'NONE',  ( 0.000000000000000000, 0.000000000000000000, 1.000000000000000000 ) ) ;
#5429=CARTESIAN_POINT ( 'NONE',  ( 18.29115343677415950, -3580.678095346448117, 2245.203709729950333 ) ) ;
#5430=CARTESIAN_POINT ( 'NONE',  ( 137.1124960021244306, -3658.322399823277465, 2249.581012931923397 ) ) ;
#5431=CIRCLE ( 'NONE', #11826, 5.715000000000884484 ) ;
#5432=VERTEX_POINT ( 'NONE', #17922 ) ;
#5433=CIRCLE ( 'NONE', #20391, 0.7619999999999987894 ) ;
#5434=CIRCLE ( 'NONE', #12923, 1.269999999999882334 ) ;
#5436=EDGE_LOOP ( 'NONE', ( #22074, #228, #4838, #17802 ) ) ;
#5437=CIRCLE ( 'NONE', #21887, 3.606800000000000228 ) ;
#5438=ORIENTED_EDGE ( 'NONE', *, *, #4359, .F. ) ;
#5440=DIRECTION ( 'NONE',  ( 0.000000000000000000, 0.000000000000000000, 1.000000000000000000 ) ) ;
#5443=DIRECTION ( 'NONE',  ( 0.000000000000000000, 0.000000000000000000, 1.000000000000000000 ) ) ;
#5445=DIRECTION ( 'NONE',  ( 1.000000000000000000, 0.000000000000000000, 0.000000000000000000 ) ) ;
#5447=FACE_OUTER_BOUND ( 'NONE', #5185, .T. ) ;
#5450=DIRECTION ( 'NONE',  ( 1.000000000000000000, 0.000000000000000000, 0.000000000000000000 ) ) ;
#5452=AXIS2_PLACEMENT_3D ( 'NONE', #4818, #15372, #15614 ) ;
#5453=VECTOR ( 'NONE', #446, 1000.000000000000000 ) ;
#5458=ORIENTED_EDGE ( 'NONE', *, *, #3562, .F. ) ;
#5460=CARTESIAN_POINT ( 'NONE',  ( 57.14999999999999858, -3543.300000000000182, 2243.277199999999993 ) ) ;
#5462=DIRECTION ( 'NONE',  ( 0.000000000000000000, 0.000000000000000000, 1.000000000000000000 ) ) ;
#5463=CYLINDRICAL_SURFACE ( 'NONE', #1467, 2.844800000000001550 ) ;
#5464=EDGE_LOOP ( 'NONE', ( #9100, #15303, #6455, #14798 ) ) ;
#5466=B_SPLINE_CURVE_WITH_KNOTS ( 'NONE', 3,
 ( #12090, #10331, #10211, #15490, #4821, #17239 ),
 .UNSPECIFIED., .F., .F.,
 ( 4, 1, 1, 4 ),
 ( 0.000000000000000000, 0.3333333333333000081, 0.6666666666667000474, 1.000000000000000000 ),
 .UNSPECIFIED. ) ;
#5467=CIRCLE ( 'NONE', #15932, 3.606799999999001027 ) ;
#5469=CARTESIAN_POINT ( 'NONE',  ( 144.5623107343992331, -3576.491783798365759, 2245.815664034198562 ) ) ;
#5470=DIRECTION ( 'NONE',  ( 0.000000000000000000, 0.000000000000000000, 1.000000000000000000 ) ) ;
#5477=ORIENTED_EDGE ( 'NONE', *, *, #13738, .T. ) ;
#5478=DIRECTION ( 'NONE',  ( -0.8068916933244306700, 0.5906994119211842476, 0.000000000000000000 ) ) ;
#5485=CARTESIAN_POINT ( 'NONE',  ( 142.3802137133438350, -3543.693183278567176, 2255.422793245767480 ) ) ;
#5489=CARTESIAN_POINT ( 'NONE',  ( 7.518185888899349578, -3577.084101415800887, 2245.168125514048825 ) ) ;
#5491=CARTESIAN_POINT ( 'NONE',  ( 127.0000000000000000, -3619.500000000000000, 2239.009999999999764 ) ) ;
#5492=AXIS2_PLACEMENT_3D ( 'NONE', #11420, #6393, #4741 ) ;
#5494=AXIS2_PLACEMENT_3D ( 'NONE', #22304, #10467, #17369 ) ;
#5498=DIRECTION ( 'NONE',  ( 0.000000000000000000, 0.000000000000000000, -1.000000000000000000 ) ) ;
#5499=CARTESIAN_POINT ( 'NONE',  ( 16.87947181989943246, -3657.399155160218470, 2246.629991729495941 ) ) ;
#5500=AXIS2_PLACEMENT_3D ( 'NONE', #7791, #20330, #14938 ) ;
#5501=AXIS2_PLACEMENT_3D ( 'NONE', #20935, #4875, #23138 ) ;
#5504=ORIENTED_EDGE ( 'NONE', *, *, #9872, .T. ) ;
#5505=DIRECTION ( 'NONE',  ( 0.000000000000000000, 0.000000000000000000, -1.000000000000000000 ) ) ;
#5511=EDGE_CURVE ( 'NONE', #10080, #9478, #17810, .T. ) ;
#5512=ORIENTED_EDGE ( 'NONE', *, *, #14461, .F. ) ;
#5514=DIRECTION ( 'NONE',  ( 1.000000000000000000, 0.000000000000000000, 0.000000000000000000 ) ) ;
#5516=ORIENTED_EDGE ( 'NONE', *, *, #18567, .F. ) ;
#5517=ADVANCED_FACE ( 'NONE', ( #14307 ), #8795, .F. ) ;
#5518=AXIS2_PLACEMENT_3D ( 'NONE', #8977, #5470, #12615 ) ;
#5519=CARTESIAN_POINT ( 'NONE',  ( 137.2761739305270510, -3580.984189840409272, 2249.284302215166917 ) ) ;
#5521=ORIENTED_EDGE ( 'NONE', *, *, #3964, .T. ) ;
#5522=DIRECTION ( 'NONE',  ( 0.000000000000000000, 0.000000000000000000, -1.000000000000000000 ) ) ;
#5526=FACE_OUTER_BOUND ( 'NONE', #18737, .T. ) ;
#5527=CARTESIAN_POINT ( 'NONE',  ( 151.1299999999999955, -3660.140000000000327, 2247.392000000000280 ) ) ;
#5528=CIRCLE ( 'NONE', #14136, 1.269999999999993356 ) ;
#5530=CARTESIAN_POINT ( 'NONE',  ( 142.1475997075216924, -3578.044972006877742, 2250.117612943123277 ) ) ;
#5532=CARTESIAN_POINT ( 'NONE',  ( 134.8403290666279872, -3576.487559777513979, 2245.822145638164784 ) ) ;
#5533=AXIS2_PLACEMENT_3D ( 'NONE', #21770, #2429, #10990 ) ;
#5535=CARTESIAN_POINT ( 'NONE',  ( 136.8552000000001669, -3579.043785370568003, 2256.063560000000052 ) ) ;
#5536=VERTEX_POINT ( 'NONE', #12424 ) ;
#5552=TOROIDAL_SURFACE ( 'NONE', #11509, 4.114799999999999791, 1.270000000000000018 ) ;
#5554=CARTESIAN_POINT ( 'NONE',  ( 35.56000000000000227, -3544.570000000000164, 2247.392000000000280 ) ) ;
#5555=VERTEX_POINT ( 'NONE', #353 ) ;
#5556=CARTESIAN_POINT ( 'NONE',  ( 18.22683998609632283, -3580.949329761737772, 2245.461031140869636 ) ) ;
#5557=CARTESIAN_POINT ( 'NONE',  ( 137.8500712042239797, -3657.343683090691684, 2247.916757465596220 ) ) ;
#5558=ORIENTED_EDGE ( 'NONE', *, *, #3248, .F. ) ;
#5559=ORIENTED_EDGE ( 'NONE', *, *, #690, .F. ) ;
#5560=CARTESIAN_POINT ( 'NONE',  ( 139.4325675808238145, -3662.349857698640790, 2249.183484300852342 ) ) ;
#5564=CARTESIAN_POINT ( 'NONE',  ( 57.14999999999999858, -3670.300000000000182, 2247.392000000000280 ) ) ;
#5565=ORIENTED_EDGE ( 'NONE', *, *, #21012, .T. ) ;
#5569=DIRECTION ( 'NONE',  ( 0.000000000000000000, 0.000000000000000000, -1.000000000000000000 ) ) ;
#5571=EDGE_LOOP ( 'NONE', ( #305, #11250, #6356, #1585, #18887, #22121, #12980, #4194, #8219, #6390 ) ) ;
#5575=FACE_OUTER_BOUND ( 'NONE', #8891, .T. ) ;
#5577=EDGE_CURVE ( 'NONE', #12211, #10812, #13354, .T. ) ;
#5578=ORIENTED_EDGE ( 'NONE', *, *, #16821, .T. ) ;
#5579=CARTESIAN_POINT ( 'NONE',  ( 131.7018428614628931, -3543.338148339810232, 2259.652932710757341 ) ) ;
#5580=ADVANCED_FACE ( 'NONE', ( #14887 ), #985, .T. ) ;
#5581=ORIENTED_EDGE ( 'NONE', *, *, #4085, .F. ) ;
#5584=CARTESIAN_POINT ( 'NONE',  ( 7.881367952664562360, -3662.577932297246662, 2245.924867616539359 ) ) ;
#5585=EDGE_CURVE ( 'NONE', #10080, #22988, #12241, .T. ) ;
#5586=EDGE_LOOP ( 'NONE', ( #12495, #4334, #10300, #8317 ) ) ;
#5587=DIRECTION ( 'NONE',  ( -0.6887494619146010688, 0.000000000000000000, -0.7249994335945012525 ) ) ;
#5590=ADVANCED_FACE ( 'NONE', ( #9602 ), #22233, .F. ) ;
#5591=CARTESIAN_POINT ( 'NONE',  ( 35.56000000000000227, -3568.700000000000273, 2244.547199999999975 ) ) ;
#5592=EDGE_LOOP ( 'NONE', ( #20136, #2501, #2330, #14997 ) ) ;
#5595=VERTEX_POINT ( 'NONE', #465 ) ;
#5596=CARTESIAN_POINT ( 'NONE',  ( 129.8447999999989975, -3619.500000000000000, 2259.837999999999738 ) ) ;
#5602=CARTESIAN_POINT ( 'NONE',  ( 7.485436129649806425, -3577.156296306550303, 2245.113781002514770 ) ) ;
#5603=EDGE_LOOP ( 'NONE', ( #6962, #6406 ) ) ;
#5606=CARTESIAN_POINT ( 'NONE',  ( 9.989231719078535576, -3543.619369469922731, 2255.346378162066230 ) ) ;
#5610=DIRECTION ( 'NONE',  ( -1.000000000000000000, 0.000000000000000000, 0.000000000000000000 ) ) ;
#5611=AXIS2_PLACEMENT_3D ( 'NONE', #2606, #9751, #7545 ) ;
#5612=FACE_OUTER_BOUND ( 'NONE', #13407, .T. ) ;
#5613=ORIENTED_EDGE ( 'NONE', *, *, #20733, .F. ) ;
#5621=CIRCLE ( 'NONE', #13840, 2.844799999999961582 ) ;
#5622=ORIENTED_EDGE ( 'NONE', *, *, #10979, .T. ) ;
#5623=CARTESIAN_POINT ( 'NONE',  ( 142.5446907139761663, -3695.594480551361812, 2255.010836426532023 ) ) ;
#5626=ORIENTED_EDGE ( 'NONE', *, *, #12161, .T. ) ;
#5627=CARTESIAN_POINT ( 'NONE',  ( 137.9085718133126761, -3581.704955524434354, 2247.466441185878466 ) ) ;
#5637=EDGE_CURVE ( 'NONE', #4904, #14376, #17190, .T. ) ;
#5639=CARTESIAN_POINT ( 'NONE',  ( 141.2946836820506746, -3577.137378286903640, 2249.656812253273529 ) ) ;
#5640=ORIENTED_EDGE ( 'NONE', *, *, #18398, .F. ) ;
#5642=CARTESIAN_POINT ( 'NONE',  ( 134.7909367546303088, -3576.568141679416840, 2245.704773985674819 ) ) ;
#5643=EDGE_CURVE ( 'NONE', #21665, #14933, #11574, .T. ) ;
#5644=ORIENTED_EDGE ( 'NONE', *, *, #8538, .T. ) ;
#5657=DIRECTION ( 'NONE',  ( 0.000000000000000000, 0.000000000000000000, -1.000000000000000000 ) ) ;
#5659=EDGE_LOOP ( 'NONE', ( #6169, #21626, #5062, #18100 ) ) ;
#5660=CARTESIAN_POINT ( 'NONE',  ( 6.984999999999000231, -3579.494999999999891, 2239.771999999999935 ) ) ;
#5661=ORIENTED_EDGE ( 'NONE', *, *, #7003, .T. ) ;
#5663=CARTESIAN_POINT ( 'NONE',  ( 137.8060722392503124, -3657.382237692640956, 2248.090672303196698 ) ) ;
#5664=CIRCLE ( 'NONE', #18735, 0.7619999999999294005 ) ;
#5665=EDGE_CURVE ( 'NONE', #140, #22588, #10735, .T. ) ;
#5669=CARTESIAN_POINT ( 'NONE',  ( 137.5443672346975745, -3661.361536096956115, 2249.961261516084505 ) ) ;
#5670=ADVANCED_FACE ( 'NONE', ( #16623 ), #9254, .T. ) ;
#5671=ORIENTED_EDGE ( 'NONE', *, *, #11946, .T. ) ;
#5673=ORIENTED_EDGE ( 'NONE', *, *, #22385, .T. ) ;
#5677=CARTESIAN_POINT ( 'NONE',  ( 15.54479999999999862, -3659.504999999999654, 2256.063560000000052 ) ) ;
#5679=DIRECTION ( 'NONE',  ( -1.000000000000000000, 0.000000000000000000, 0.000000000000000000 ) ) ;
#5682=AXIS2_PLACEMENT_3D ( 'NONE', #6136, #18430, #9862 ) ;
#5685=FACE_BOUND ( 'NONE', #178, .T. ) ;
#5686=CARTESIAN_POINT ( 'NONE',  ( 7.161827360861991565, -3580.901497745790039, 2245.410526384100649 ) ) ;
#5690=CARTESIAN_POINT ( 'NONE',  ( 131.7495946018047164, -3543.379535511729046, 2259.772542604667706 ) ) ;
#5692=CARTESIAN_POINT ( 'NONE',  ( 114.2999999999999972, -3594.099999999999909, 2239.771999999999935 ) ) ;
#5693=DIRECTION ( 'NONE',  ( -1.000000000000000000, 0.000000000000000000, 0.000000000000000000 ) ) ;
#5695=ORIENTED_EDGE ( 'NONE', *, *, #1195, .T. ) ;
#5697=SPHERICAL_SURFACE ( 'NONE', #5123, 1.270000000000000018 ) ;
#5699=CIRCLE ( 'NONE', #89, 0.7619999999999987894 ) ;
#5704=EDGE_CURVE ( 'NONE', #15378, #6511, #23063, .T. ) ;
#5707=ORIENTED_EDGE ( 'NONE', *, *, #3137, .T. ) ;
#5708=CARTESIAN_POINT ( 'NONE',  ( 147.7417438321762404, -3695.684722677512127, 2259.544515782609324 ) ) ;
#5713=CARTESIAN_POINT ( 'NONE',  ( 142.2521676912461999, -3544.290797605575335, 2255.743587683598435 ) ) ;
#5717=AXIS2_PLACEMENT_3D ( 'NONE', #16083, #7183, #14336 ) ;
#5718=CARTESIAN_POINT ( 'NONE',  ( 7.139750157027973110, -3578.173783392149744, 2244.630952135868938 ) ) ;
#5719=ORIENTED_EDGE ( 'NONE', *, *, #15246, .F. ) ;
#5725=EDGE_CURVE ( 'NONE', #10346, #5746, #3023, .T. ) ;
#5726=CARTESIAN_POINT ( 'NONE',  ( 101.5999999999999943, -3568.700000000000273, 2239.009999999999764 ) ) ;
#5727=ADVANCED_FACE ( 'NONE', ( #22815 ), #10169, .F. ) ;
#5729=ORIENTED_EDGE ( 'NONE', *, *, #17685, .F. ) ;
#5731=CARTESIAN_POINT ( 'NONE',  ( 134.9402830941174898, -3662.669251256681946, 2246.087205945077585 ) ) ;
#5732=CARTESIAN_POINT ( 'NONE',  ( 25.39999999999999858, -3660.140000000000327, 2247.392000000000280 ) ) ;
#5736=CIRCLE ( 'NONE', #15453, 0.7619999999999987894 ) ;
#5737=EDGE_CURVE ( 'NONE', #4127, #16752, #14434, .T. ) ;
#5741=VECTOR ( 'NONE', #17274, 1000.000000000000000 ) ;
#5742=ORIENTED_EDGE ( 'NONE', *, *, #7816, .F. ) ;
#5743=CARTESIAN_POINT ( 'NONE',  ( 142.3294809625096775, -3695.151712724517893, 2255.549776698367168 ) ) ;
#5745=AXIS2_PLACEMENT_3D ( 'NONE', #22708, #4788, #6438 ) ;
#5746=VERTEX_POINT ( 'NONE', #16967 ) ;
#5747=CARTESIAN_POINT ( 'NONE',  ( 137.8998175441851686, -3581.697724730667233, 2247.187286018316172 ) ) ;
#5750=CARTESIAN_POINT ( 'NONE',  ( 145.4149999194000316, -3579.609095813974363, 2244.645121672132518 ) ) ;
#5754=FACE_OUTER_BOUND ( 'NONE', #10645, .T. ) ;
#5757=DIRECTION ( 'NONE',  ( 0.000000000000000000, 0.000000000000000000, -1.000000000000000000 ) ) ;
#5758=CARTESIAN_POINT ( 'NONE',  ( 137.9912716215963542, -3577.220450210613308, 2249.716878566800460 ) ) ;
#5759=EDGE_LOOP ( 'NONE', ( #21581, #14386, #3273, #19353 ) ) ;
#5761=CARTESIAN_POINT ( 'NONE',  ( 134.3629476791235504, -3577.447007153130926, 2244.917889002162610 ) ) ;
#5762=AXIS2_PLACEMENT_3D ( 'NONE', #12627, #18347, #14850 ) ;
#5767=VECTOR ( 'NONE', #7836, 1000.000000000000000 ) ;
#5768=CIRCLE ( 'NONE', #13611, 1.269999999999882334 ) ;
#5769=ORIENTED_EDGE ( 'NONE', *, *, #15533, .T. ) ;
#5773=CARTESIAN_POINT ( 'NONE',  ( 50.79999999999999716, -3568.700000000000273, 2259.837999999999738 ) ) ;
#5775=CARTESIAN_POINT ( 'NONE',  ( 50.79999999999999716, -3670.300000000000182, 2261.869999999999891 ) ) ;
#5776=EDGE_LOOP ( 'NONE', ( #10627, #9894 ) ) ;
#5777=CARTESIAN_POINT ( 'NONE',  ( 127.0000000000000000, -3670.300000000000182, 2259.837999999999738 ) ) ;
#5778=CIRCLE ( 'NONE', #1265, 2.844800000000091700 ) ;
#5781=CARTESIAN_POINT ( 'NONE',  ( 139.6999999999999886, -3579.494999999999891, 2239.771999999999935 ) ) ;
#5782=CARTESIAN_POINT ( 'NONE',  ( 9.923473159618289685, -3578.875297092680739, 2250.236699640666302 ) ) ;
#5783=ORIENTED_EDGE ( 'NONE', *, *, #15254, .T. ) ;
#5784=CARTESIAN_POINT ( 'NONE',  ( 18.26250405562707613, -3580.806353043069066, 2245.317242612439259 ) ) ;
#5785=DIRECTION ( 'NONE',  ( 0.000000000000000000, 0.000000000000000000, -1.000000000000000000 ) ) ;
#5787=CARTESIAN_POINT ( 'NONE',  ( 137.2524928180403947, -3660.955183479468360, 2250.117566548333343 ) ) ;
#5788=ORIENTED_EDGE ( 'NONE', *, *, #9373, .F. ) ;
#5792=CARTESIAN_POINT ( 'NONE',  ( 57.14999999999999858, -3694.430000000000291, 2247.392000000000280 ) ) ;
#5795=DIRECTION ( 'NONE',  ( -1.073225997510925892E-13, 0.000000000000000000, -1.000000000000000000 ) ) ;
#5797=CARTESIAN_POINT ( 'NONE',  ( 12.69999999999999929, -3659.504999999999654, 2246.630000000000109 ) ) ;
#5802=CARTESIAN_POINT ( 'NONE',  ( 7.149936657841415411, -3580.855533714582634, 2245.364243621501828 ) ) ;
#5803=ADVANCED_FACE ( 'NONE', ( #15335 ), #15970, .T. ) ;
#5806=EDGE_CURVE ( 'NONE', #12349, #6304, #5883, .T. ) ;
#5807=FACE_OUTER_BOUND ( 'NONE', #17476, .T. ) ;
#5809=VECTOR ( 'NONE', #14895, 1000.000000000000000 ) ;
#5810=CIRCLE ( 'NONE', #1673, 2.844800000000001550 ) ;
#5811=DIRECTION ( 'NONE',  ( 1.000000000000000000, -0.000000000000000000, -0.000000000000000000 ) ) ;
#5812=ORIENTED_EDGE ( 'NONE', *, *, #5208, .F. ) ;
#5813=CARTESIAN_POINT ( 'NONE',  ( 7.361549341673686797, -3661.582738350905856, 2244.919123108159965 ) ) ;
#5816=EDGE_CURVE ( 'NONE', #16978, #17829, #6631, .T. ) ;
#5822=ORIENTED_EDGE ( 'NONE', *, *, #4996, .F. ) ;
#5823=DIRECTION ( 'NONE',  ( -1.000000000000000000, 0.000000000000000000, 0.000000000000000000 ) ) ;
#5826=DIRECTION ( 'NONE',  ( 1.000000000000000000, 0.000000000000000000, 0.000000000000000000 ) ) ;
#5827=AXIS2_PLACEMENT_3D ( 'NONE', #18281, #21913, #7398 ) ;
#5832=DIRECTION ( 'NONE',  ( 0.000000000000000000, 0.000000000000000000, -1.000000000000000000 ) ) ;
#5834=CARTESIAN_POINT ( 'NONE',  ( 129.8447999999989975, -3670.300000000000182, 2239.771999999999935 ) ) ;
#5835=ORIENTED_EDGE ( 'NONE', *, *, #18028, .T. ) ;
#5839=VERTEX_POINT ( 'NONE', #4787 ) ;
#5840=CARTESIAN_POINT ( 'NONE',  ( 145.4114887792144373, -3659.274894571976347, 2244.679117411749758 ) ) ;
#5841=EDGE_CURVE ( 'NONE', #14892, #14824, #16035, .T. ) ;
#5845=AXIS2_PLACEMENT_3D ( 'NONE', #1951, #537, #3936 ) ;
#5846=ORIENTED_EDGE ( 'NONE', *, *, #15729, .F. ) ;
#5848=CYLINDRICAL_SURFACE ( 'NONE', #16737, 2.844800000000091700 ) ;
#5851=DIRECTION ( 'NONE',  ( 0.7249994335945985080, 0.000000000000000000, -0.6887494619144985952 ) ) ;
#5852=ORIENTED_EDGE ( 'NONE', *, *, #9548, .F. ) ;
#5853=DIRECTION ( 'NONE',  ( 0.000000000000000000, 0.000000000000000000, 1.000000000000000000 ) ) ;
#5854=EDGE_LOOP ( 'NONE', ( #20497, #17861, #8388, #18404, #20486, #17643 ) ) ;
#5855=EDGE_CURVE ( 'NONE', #8104, #4940, #14122, .T. ) ;
#5861=TOROIDAL_SURFACE ( 'NONE', #14078, 3.606799999999999784, 0.7620000000000000107 ) ;
#5862=ORIENTED_EDGE ( 'NONE', *, *, #12576, .F. ) ;
#5863=AXIS2_PLACEMENT_3D ( 'NONE', #1572, #3446, #19157 ) ;
#5864=DIRECTION ( 'NONE',  ( 0.000000000000000000, -1.000000000000000000, 0.000000000000000000 ) ) ;
#5868=EDGE_CURVE ( 'NONE', #12207, #13662, #12998, .T. ) ;
#5870=AXIS2_PLACEMENT_3D ( 'NONE', #15740, #9990, #18895 ) ;
#5871=ADVANCED_FACE ( 'NONE', ( #15799 ), #3487, .T. ) ;
#5872=CARTESIAN_POINT ( 'NONE',  ( 17.75414321264302231, -3662.172752710656368, 2245.401715040317413 ) ) ;
#5875=CARTESIAN_POINT ( 'NONE',  ( 142.4398810773762136, -3578.715266063343279, 2250.236799993183013 ) ) ;
#5876=EDGE_CURVE ( 'NONE', #21098, #4940, #3635, .T. ) ;
#5877=ORIENTED_EDGE ( 'NONE', *, *, #20733, .T. ) ;
#5883=CIRCLE ( 'NONE', #3617, 0.7619999999999294005 ) ;
#5885=ADVANCED_FACE ( 'NONE', ( #14281 ), #6276, .T. ) ;
#5886=ADVANCED_FACE ( 'NONE', ( #14047 ), #14396, .F. ) ;
#5889=CARTESIAN_POINT ( 'NONE',  ( 15.50028889993228987, -3658.999884688285874, 2249.998575292800069 ) ) ;
#5890=VERTEX_POINT ( 'NONE', #12515 ) ;
#5892=CARTESIAN_POINT ( 'NONE',  ( 13.53605320222184893, -3576.775764562235054, 2249.328209726781552 ) ) ;
#5893=PLANE ( 'NONE',  #2008 ) ;
#5894=ORIENTED_EDGE ( 'NONE', *, *, #898, .T. ) ;
#5895=AXIS2_PLACEMENT_3D ( 'NONE', #20871, #1289, #19696 ) ;
#5896=CYLINDRICAL_SURFACE ( 'NONE', #6272, 2.844800000000001550 ) ;
#5898=AXIS2_PLACEMENT_3D ( 'NONE', #20895, #22861, #1661 ) ;
#5902=CIRCLE ( 'NONE', #13359, 2.844800000000001550 ) ;
#5904=CARTESIAN_POINT ( 'NONE',  ( 140.9027360924337131, -3662.083407271924443, 2249.469647930371593 ) ) ;
#5905=ORIENTED_EDGE ( 'NONE', *, *, #11492, .F. ) ;
#5907=ORIENTED_EDGE ( 'NONE', *, *, #939, .F. ) ;
#5908=AXIS2_PLACEMENT_3D ( 'NONE', #17838, #1786, #8934 ) ;
#5913=CARTESIAN_POINT ( 'NONE',  ( 114.2999999999999972, -3594.099999999999909, 2261.869999999999891 ) ) ;
#5916=CARTESIAN_POINT ( 'NONE',  ( 7.053810164393185644, -3658.615721339214815, 2244.986590707419509 ) ) ;
#5918=FACE_BOUND ( 'NONE', #18357, .T. ) ;
#5919=CARTESIAN_POINT ( 'NONE',  ( 6.997747388991874651, -3579.940010871207051, 2244.748233079088095 ) ) ;
#5925=CARTESIAN_POINT ( 'NONE',  ( 142.4123320799332362, -3658.645882986786091, 2249.813345329157983 ) ) ;
#5927=DIRECTION ( 'NONE',  ( -1.000000000000000000, 0.000000000000000000, 0.000000000000000000 ) ) ;
#5929=DIRECTION ( 'NONE',  ( 0.000000000000000000, 1.000000000000000000, 0.000000000000000000 ) ) ;
#5931=EDGE_CURVE ( 'NONE', #18295, #4608, #218, .T. ) ;
#5932=EDGE_CURVE ( 'NONE', #6015, #11279, #22342, .T. ) ;
#5933=CARTESIAN_POINT ( 'NONE',  ( 17.31138602737999932, -3662.880847139000252, 2246.630000000000109 ) ) ;
#5934=CARTESIAN_POINT ( 'NONE',  ( 85.29320000000001301, -3594.099999999999909, 2239.009999999999764 ) ) ;
#5937=CARTESIAN_POINT ( 'NONE',  ( 0.000000000000000000, -3694.430000000000291, 2240.279999999999745 ) ) ;
#5939=DIRECTION ( 'NONE',  ( 1.000000000000000000, 0.000000000000000000, 0.000000000000000000 ) ) ;
#5942=CIRCLE ( 'NONE', #18220, 1.269999999999882334 ) ;
#5943=DIRECTION ( 'NONE',  ( 0.000000000000000000, 0.000000000000000000, -1.000000000000000000 ) ) ;
#5944=CARTESIAN_POINT ( 'NONE',  ( 142.4830070222579366, -3543.485052020446346, 2255.165585415843907 ) ) ;
#5950=DIRECTION ( 'NONE',  ( -1.000000000000000000, 0.000000000000000000, 0.000000000000000000 ) ) ;
#5951=CARTESIAN_POINT ( 'NONE',  ( 127.0000000000000000, -3619.500000000000000, 2261.869999999999891 ) ) ;
#5954=CARTESIAN_POINT ( 'NONE',  ( 151.4000000000000057, -3543.329032635400836, 2259.329999999999927 ) ) ;
#5955=EDGE_CURVE ( 'NONE', #14185, #16978, #9272, .T. ) ;
#5958=ORIENTED_EDGE ( 'NONE', *, *, #12746, .F. ) ;
#5959=EDGE_CURVE ( 'NONE', #7862, #4904, #15920, .T. ) ;
#5961=ADVANCED_FACE ( 'NONE', ( #5612 ), #15255, .T. ) ;
#5962=DIRECTION ( 'NONE',  ( 0.7249994335945011414, 0.000000000000000000, -0.6887494619146010688 ) ) ;
#5966=ORIENTED_EDGE ( 'NONE', *, *, #8742, .F. ) ;
#5967=DIRECTION ( 'NONE',  ( -1.000000000000000000, 0.000000000000000000, 0.000000000000000000 ) ) ;
#5976=CARTESIAN_POINT ( 'NONE',  ( 145.1262588623648639, -3581.288617102159606, 2245.910525606668671 ) ) ;
#5978=DIRECTION ( 'NONE',  ( -1.000000000000000000, 0.000000000000000000, 0.000000000000000000 ) ) ;
#5979=CARTESIAN_POINT ( 'NONE',  ( 12.69999999999999929, -3579.494999999999891, 2272.030000000000200 ) ) ;
#5980=EDGE_CURVE ( 'NONE', #444, #20696, #14512, .T. ) ;
#5981=CARTESIAN_POINT ( 'NONE',  ( 142.2033847376006861, -3578.142761313953997, 2250.145277428746340 ) ) ;
#5983=VECTOR ( 'NONE', #9600, 1000.000000000000000 ) ;
#5984=ORIENTED_EDGE ( 'NONE', *, *, #3127, .F. ) ;
#5985=DIRECTION ( 'NONE',  ( 1.000000000000000000, 0.000000000000000000, 0.000000000000000000 ) ) ;
#5990=CARTESIAN_POINT ( 'NONE',  ( 15.55031652512126250, -3543.399485434554663, 2254.996725890375274 ) ) ;
#5992=EDGE_CURVE ( 'NONE', #3669, #11744, #20130, .T. ) ;
#5994=CARTESIAN_POINT ( 'NONE',  ( 20.09942059832000183, -3544.570000000000164, 2260.390449568000349 ) ) ;
#5995=ORIENTED_EDGE ( 'NONE', *, *, #15180, .F. ) ;
#5997=CARTESIAN_POINT ( 'NONE',  ( 13.55725822396861524, -3576.782357048964968, 2249.335288272477101 ) ) ;
#5998=CARTESIAN_POINT ( 'NONE',  ( 142.2474702748325512, -3580.761556601727989, 2249.508564178021970 ) ) ;
#5999=EDGE_CURVE ( 'NONE', #12999, #5355, #10005, .T. ) ;
#6005=DIRECTION ( 'NONE',  ( 0.000000000000000000, 0.000000000000000000, 1.000000000000000000 ) ) ;
#6006=EDGE_LOOP ( 'NONE', ( #19604, #21145, #7257, #9959 ) ) ;
#6008=CARTESIAN_POINT ( 'NONE',  ( 20.75864668056231821, -3543.309784082139231, 2259.501798909290756 ) ) ;
#6012=EDGE_CURVE ( 'NONE', #7575, #22920, #22100, .T. ) ;
#6014=CARTESIAN_POINT ( 'NONE',  ( 141.8956724088833994, -3661.315849440774400, 2249.983377711600951 ) ) ;
#6015=VERTEX_POINT ( 'NONE', #5954 ) ;
#6019=LINE ( 'NONE', #8001, #6938 ) ;
#6023=CARTESIAN_POINT ( 'NONE',  ( 38.10000000000000142, -3644.899999999999636, 2239.009999999999764 ) ) ;
#6025=ORIENTED_EDGE ( 'NONE', *, *, #13883, .T. ) ;
#6026=CARTESIAN_POINT ( 'NONE',  ( 7.275104262493744756, -3657.707260169260735, 2245.917323013845817 ) ) ;
#6032=CARTESIAN_POINT ( 'NONE',  ( 95.25000000000000000, -3694.430000000000291, 2247.392000000000280 ) ) ;
#6033=DIRECTION ( 'NONE',  ( 0.000000000000000000, 0.000000000000000000, 1.000000000000000000 ) ) ;
#6040=ORIENTED_EDGE ( 'NONE', *, *, #3183, .F. ) ;
#6042=CARTESIAN_POINT ( 'NONE',  ( 110.6932000000009992, -3594.099999999999909, 2260.600000000000364 ) ) ;
#6048=B_SPLINE_CURVE_WITH_KNOTS ( 'NONE', 3,
 ( #7059, #5411, #14664, #20055 ),
 .UNSPECIFIED., .F., .F.,
 ( 4, 4 ),
 ( 0.000000000000000000, 1.000000000000000000 ),
 .UNSPECIFIED. ) ;
#6049=CYLINDRICAL_SURFACE ( 'NONE', #16864, 1.269999999999898099 ) ;
#6055=DIRECTION ( 'NONE',  ( 0.000000000000000000, -1.000000000000000000, 0.000000000000000000 ) ) ;
#6056=DIRECTION ( 'NONE',  ( 1.000000000000000000, 0.000000000000000000, 0.000000000000000000 ) ) ;
#6059=VERTEX_POINT ( 'NONE', #21877 ) ;
#6064=CIRCLE ( 'NONE', #19147, 3.606799999998994366 ) ;
#6069=DIRECTION ( 'NONE',  ( 0.000000000000000000, 0.000000000000000000, 1.000000000000000000 ) ) ;
#6071=DIRECTION ( 'NONE',  ( 1.000000000000000000, 0.000000000000000000, 0.000000000000000000 ) ) ;
#6072=CARTESIAN_POINT ( 'NONE',  ( 131.7757523116999891, -3695.699999999999818, 2259.837999999999738 ) ) ;
#6076=AXIS2_PLACEMENT_3D ( 'NONE', #14626, #2203, #21767 ) ;
#6082=CARTESIAN_POINT ( 'NONE',  ( 144.3113860274000047, -3662.880847139000252, 2246.630000000000109 ) ) ;
#6083=ORIENTED_EDGE ( 'NONE', *, *, #9997, .T. ) ;
#6084=ORIENTED_EDGE ( 'NONE', *, *, #7023, .F. ) ;
#6085=EDGE_CURVE ( 'NONE', #7043, #7639, #19368, .T. ) ;
#6089=CARTESIAN_POINT ( 'NONE',  ( 145.2719119545006947, -3580.765843483391563, 2245.279837210061032 ) ) ;
#6092=ADVANCED_FACE ( 'NONE', ( #552 ), #5848, .F. ) ;
#6094=FACE_OUTER_BOUND ( 'NONE', #6686, .T. ) ;
#6096=AXIS2_PLACEMENT_3D ( 'NONE', #10283, #6673, #19429 ) ;
#6097=CARTESIAN_POINT ( 'NONE',  ( 50.79999999999999716, -3670.300000000000182, 2239.771999999999935 ) ) ;
#6098=CARTESIAN_POINT ( 'NONE',  ( 72.59320000000001016, -3670.300000000000182, 2259.837999999999738 ) ) ;
#6100=CARTESIAN_POINT ( 'NONE',  ( 137.8823296110995216, -3577.304701220188235, 2249.774946555156021 ) ) ;
#6101=EDGE_LOOP ( 'NONE', ( #13264, #10913, #22715, #2650 ) ) ;
#6103=CARTESIAN_POINT ( 'NONE',  ( 1.270000000000000018, -3544.570000000000164, 2259.329999999999927 ) ) ;
#6108=AXIS2_PLACEMENT_3D ( 'NONE', #20186, #14915, #6127 ) ;
#6109=ORIENTED_EDGE ( 'NONE', *, *, #4408, .T. ) ;
#6111=ORIENTED_EDGE ( 'NONE', *, *, #548, .T. ) ;
#6113=AXIS2_PLACEMENT_3D ( 'NONE', #6514, #14954, #20671 ) ;
#6116=CARTESIAN_POINT ( 'NONE',  ( 35.56000000000000227, -3544.570000000000164, 2251.506800000000112 ) ) ;
#6117=CARTESIAN_POINT ( 'NONE',  ( 12.56749442210865197, -3576.650097218246174, 2249.183428692989310 ) ) ;
#6118=CARTESIAN_POINT ( 'NONE',  ( 142.5253973193343597, -3579.881039274069281, 2250.055385365074471 ) ) ;
#6122=EDGE_CURVE ( 'NONE', #9353, #3735, #21403, .T. ) ;
#6123=DIRECTION ( 'NONE',  ( -1.000000000000000000, 0.000000000000000000, 0.000000000000000000 ) ) ;
#6124=CARTESIAN_POINT ( 'NONE',  ( 20.53780452085382180, -3543.526739948642899, 2260.054530369292934 ) ) ;
#6125=AXIS2_PLACEMENT_3D ( 'NONE', #1525, #21452, #12316 ) ;
#6127=DIRECTION ( 'NONE',  ( 1.000000000000000000, 0.000000000000000000, 0.000000000000000000 ) ) ;
#6130=AXIS2_PLACEMENT_3D ( 'NONE', #18435, #16787, #8233 ) ;
#6134=ORIENTED_EDGE ( 'NONE', *, *, #1531, .T. ) ;
#6136=CARTESIAN_POINT ( 'NONE',  ( 101.5999999999999943, -3619.500000000000000, 2259.837999999999738 ) ) ;
#6139=ADVANCED_FACE ( 'NONE', ( #12023 ), #10378, .T. ) ;
#6142=CARTESIAN_POINT ( 'NONE',  ( 151.1299999999999955, -3660.140000000000327, 2243.277199999999993 ) ) ;
#6147=ADVANCED_FACE ( 'NONE', ( #1234 ), #13545, .F. ) ;
#6148=DIRECTION ( 'NONE',  ( 1.000000000000000000, 0.000000000000000000, -1.224646799147353207E-16 ) ) ;
#6150=B_SPLINE_CURVE_WITH_KNOTS ( 'NONE', 3,
 ( #919, #9719, #11940, #22136 ),
 .UNSPECIFIED., .F., .F.,
 ( 4, 4 ),
 ( 0.000000000000000000, 1.000000000000000000 ),
 .UNSPECIFIED. ) ;
#6152=VECTOR ( 'NONE', #8403, 1000.000000000000000 ) ;
#6158=ORIENTED_EDGE ( 'NONE', *, *, #1813, .F. ) ;
#6166=DIRECTION ( 'NONE',  ( -1.224646799147353207E-16, 1.000000000000000000, 0.000000000000000000 ) ) ;
#6168=FACE_OUTER_BOUND ( 'NONE', #20243, .T. ) ;
#6169=ORIENTED_EDGE ( 'NONE', *, *, #7501, .F. ) ;
#6171=AXIS2_PLACEMENT_3D ( 'NONE', #21860, #14374, #21405 ) ;
#6174=CARTESIAN_POINT ( 'NONE',  ( 145.0244890045273962, -3657.428455897194453, 2246.524599549557479 ) ) ;
#6175=CARTESIAN_POINT ( 'NONE',  ( 63.50000000000000000, -3644.899999999999636, 2239.009999999999764 ) ) ;
#6180=CIRCLE ( 'NONE', #5494, 3.606799999999993567 ) ;
#6182=CARTESIAN_POINT ( 'NONE',  ( 134.0203227398999957, -3578.860230781999689, 2244.548186305999934 ) ) ;
#6183=VERTEX_POINT ( 'NONE', #15195 ) ;
#6184=CARTESIAN_POINT ( 'NONE',  ( 130.6067999999989979, -3619.500000000000000, 2260.600000000000364 ) ) ;
#6191=DIRECTION ( 'NONE',  ( -1.000000000000000000, 0.000000000000000000, 0.000000000000000000 ) ) ;
#6194=CARTESIAN_POINT ( 'NONE',  ( 130.6067999999989979, -3568.700000000000273, 2260.600000000000364 ) ) ;
#6195=ORIENTED_EDGE ( 'NONE', *, *, #16299, .F. ) ;
#6197=AXIS2_PLACEMENT_3D ( 'NONE', #10821, #7312, #14921 ) ;
#6199=CARTESIAN_POINT ( 'NONE',  ( 145.0128742528999908, -3581.600847139000052, 2246.630000000000109 ) ) ;
#6200=AXIS2_PLACEMENT_3D ( 'NONE', #10905, #7742, #15001 ) ;
#6202=AXIS2_PLACEMENT_3D ( 'NONE', #226, #5853, #9354 ) ;
#6203=FACE_OUTER_BOUND ( 'NONE', #949, .T. ) ;
#6204=CARTESIAN_POINT ( 'NONE',  ( 17.98800820957344726, -3661.672316069987119, 2244.994777904991679 ) ) ;
#6212=DIRECTION ( 'NONE',  ( -1.000000000000000000, 0.000000000000000000, 0.000000000000000000 ) ) ;
#6214=CARTESIAN_POINT ( 'NONE',  ( 98.75520000000000209, -3568.700000000000273, 2261.869999999999891 ) ) ;
#6215=ORIENTED_EDGE ( 'NONE', *, *, #4987, .F. ) ;
#6216=EDGE_CURVE ( 'NONE', #22780, #3143, #20466, .T. ) ;
#6219=CARTESIAN_POINT ( 'NONE',  ( 15.38584772739802986, -3543.678681369468450, 2255.408757311840873 ) ) ;
#6221=EDGE_CURVE ( 'NONE', #6713, #15342, #12203, .T. ) ;
#6224=VERTEX_POINT ( 'NONE', #8043 ) ;
#6228=ORIENTED_EDGE ( 'NONE', *, *, #22096, .T. ) ;
#6229=DIRECTION ( 'NONE',  ( -1.000000000000000000, 0.000000000000000000, 0.000000000000000000 ) ) ;
#6230=CARTESIAN_POINT ( 'NONE',  ( 14.93501350881909850, -3577.734074929383951, 2250.004932963394367 ) ) ;
#6232=AXIS2_PLACEMENT_3D ( 'NONE', #19337, #10187, #8670 ) ;
#6233=EDGE_CURVE ( 'NONE', #14640, #15062, #8466, .T. ) ;
#6234=CARTESIAN_POINT ( 'NONE',  ( 141.9421027588409174, -3581.246006357328497, 2248.941170909273296 ) ) ;
#6238=DIRECTION ( 'NONE',  ( 0.000000000000000000, 0.000000000000000000, -1.000000000000000000 ) ) ;
#6240=ADVANCED_FACE ( 'NONE', ( #19173 ), #15571, .T. ) ;
#6243=AXIS2_PLACEMENT_3D ( 'NONE', #6329, #13701, #18728 ) ;
#6247=EDGE_LOOP ( 'NONE', ( #15121, #19869 ) ) ;
#6248=ORIENTED_EDGE ( 'NONE', *, *, #3343, .T. ) ;
#6251=EDGE_CURVE ( 'NONE', #9808, #8713, #4344, .T. ) ;
#6254=VERTEX_POINT ( 'NONE', #2885 ) ;
#6256=FACE_OUTER_BOUND ( 'NONE', #18103, .T. ) ;
#6257=EDGE_LOOP ( 'NONE', ( #11586, #13019, #16815, #22480 ) ) ;
#6261=AXIS2_PLACEMENT_3D ( 'NONE', #22127, #7494, #2340 ) ;
#6264=CIRCLE ( 'NONE', #11480, 0.7619999999999294005 ) ;
#6269=CARTESIAN_POINT ( 'NONE',  ( 111.4552000000009997, -3644.899999999999636, 2239.771999999999935 ) ) ;
#6271=CARTESIAN_POINT ( 'NONE',  ( 136.7387998463173062, -3543.315277319925826, 2254.718298687770584 ) ) ;
#6272=AXIS2_PLACEMENT_3D ( 'NONE', #7985, #2586, #16987 ) ;
#6274=EDGE_LOOP ( 'NONE', ( #16037, #17200, #20256, #19117 ) ) ;
#6276=TOROIDAL_SURFACE ( 'NONE', #291, 3.606799999998999695, 0.7620000000000000107 ) ;
#6280=ORIENTED_EDGE ( 'NONE', *, *, #4937, .T. ) ;
#6281=DIRECTION ( 'NONE',  ( 0.000000000000000000, 0.000000000000000000, 1.000000000000000000 ) ) ;
#6284=ADVANCED_FACE ( 'NONE', ( #2646, #6529, #20813, #11907, #10029, #22786, #8515, #15661, #13317, #17878, #19762, #3459, #17518, #19518, #13902, #21397, #5346, #10377, #1823, #21050, #21288, #4995, #3692 ), #15775, .T. ) ;
#6285=ADVANCED_FACE ( 'NONE', ( #8972 ), #20081, .T. ) ;
#6288=EDGE_CURVE ( 'NONE', #6818, #15892, #21199, .T. ) ;
#6289=CARTESIAN_POINT ( 'NONE',  ( 20.79047622000200946, -3695.700000000006639, 2259.421674269511641 ) ) ;
#6295=AXIS2_PLACEMENT_3D ( 'NONE', #23075, #7159, #21338 ) ;
#6300=CARTESIAN_POINT ( 'NONE',  ( 63.50000000000000000, -3644.899999999999636, 2239.771999999999935 ) ) ;
#6304=VERTEX_POINT ( 'NONE', #23134 ) ;
#6305=LINE ( 'NONE', #14970, #9956 ) ;
#6306=CARTESIAN_POINT ( 'NONE',  ( 14.63600372084860624, -3661.589906291256284, 2249.839665659381353 ) ) ;
#6307=CIRCLE ( 'NONE', #17140, 3.606799999998994366 ) ;
#6309=VERTEX_POINT ( 'NONE', #10842 ) ;
#6310=CARTESIAN_POINT ( 'NONE',  ( 35.56000000000000227, -3543.299999999999727, 2247.392000000000280 ) ) ;
#6312=EDGE_CURVE ( 'NONE', #14341, #9781, #6618, .T. ) ;
#6314=CARTESIAN_POINT ( 'NONE',  ( 85.29320000000001301, -3644.899999999999636, 2239.771999999999935 ) ) ;
#6316=ORIENTED_EDGE ( 'NONE', *, *, #5146, .F. ) ;
#6317=EDGE_LOOP ( 'NONE', ( #5504, #720 ) ) ;
#6322=CARTESIAN_POINT ( 'NONE',  ( 101.5999999999999943, -3568.700000000000273, 2259.837999999999738 ) ) ;
#6323=CARTESIAN_POINT ( 'NONE',  ( 17.92468170931930160, -3661.821022282586000, 2245.096946498718353 ) ) ;
#6325=CARTESIAN_POINT ( 'NONE',  ( 54.40679999999999694, -3619.500000000000000, 2259.837999999999738 ) ) ;
#6329=CARTESIAN_POINT ( 'NONE',  ( 114.2999999999999972, -3594.099999999999909, 2260.600000000000364 ) ) ;
#6330=FACE_OUTER_BOUND ( 'NONE', #7796, .T. ) ;
#6332=CARTESIAN_POINT ( 'NONE',  ( 127.0000000000000000, -3670.300000000000182, 2239.771999999999935 ) ) ;
#6333=CARTESIAN_POINT ( 'NONE',  ( 10.84178118933141377, -3657.349603116384515, 2246.808232705630871 ) ) ;
#6334=ORIENTED_EDGE ( 'NONE', *, *, #19767, .T. ) ;
#6340=TOROIDAL_SURFACE ( 'NONE', #7457, 3.606799999999999784, 0.7620000000000000107 ) ;
#6344=CARTESIAN_POINT ( 'NONE',  ( 13.90342121230041528, -3576.915831503414665, 2249.469455096983438 ) ) ;
#6346=CARTESIAN_POINT ( 'NONE',  ( 141.8951334675158478, -3581.304718316791423, 2248.847051393844140 ) ) ;
#6348=DIRECTION ( 'NONE',  ( 0.000000000000000000, 0.000000000000000000, -1.000000000000000000 ) ) ;
#6351=CARTESIAN_POINT ( 'NONE',  ( 9.855200000000680305, -3579.043785370519799, 2256.063559999999597 ) ) ;
#6352=LINE ( 'NONE', #13374, #22319 ) ;
#6354=EDGE_CURVE ( 'NONE', #20632, #15794, #14253, .T. ) ;
#6355=CARTESIAN_POINT ( 'NONE',  ( 134.0034857541872100, -3659.043311792284385, 2244.766319695583661 ) ) ;
#6356=ORIENTED_EDGE ( 'NONE', *, *, #13116, .F. ) ;
#6364=DIRECTION ( 'NONE',  ( 0.000000000000000000, 0.000000000000000000, 1.000000000000000000 ) ) ;
#6375=FACE_OUTER_BOUND ( 'NONE', #16099, .T. ) ;
#6377=DIRECTION ( 'NONE',  ( 0.000000000000000000, 0.000000000000000000, 1.000000000000000000 ) ) ;
#6380=CARTESIAN_POINT ( 'NONE',  ( 142.0115892277856631, -3657.846812289455102, 2249.075827970531918 ) ) ;
#6383=ORIENTED_EDGE ( 'NONE', *, *, #16561, .F. ) ;
#6384=CARTESIAN_POINT ( 'NONE',  ( 136.9315409364155869, -3543.507962132184730, 2255.201583317368204 ) ) ;
#6390=ORIENTED_EDGE ( 'NONE', *, *, #8058, .T. ) ;
#6392=CARTESIAN_POINT ( 'NONE',  ( 18.41499991942999870, -3579.284285772028397, 2244.570689628976652 ) ) ;
#6393=DIRECTION ( 'NONE',  ( 0.7249994335945011414, 0.000000000000000000, 0.6887494619146010688 ) ) ;
#6400=CARTESIAN_POINT ( 'NONE',  ( 105.2067999999999870, -3568.700000000000273, 2239.009999999999764 ) ) ;
#6403=ADVANCED_FACE ( 'NONE', ( #2180 ), #20106, .F. ) ;
#6405=CARTESIAN_POINT ( 'NONE',  ( 101.5999999999999943, -3670.300000000000182, 2239.009999999999764 ) ) ;
#6406=ORIENTED_EDGE ( 'NONE', *, *, #9516, .T. ) ;
#6409=CIRCLE ( 'NONE', #15384, 3.606800000000000228 ) ;
#6410=ADVANCED_FACE ( 'NONE', ( #3806 ), #1342, .T. ) ;
#6412=CARTESIAN_POINT ( 'NONE',  ( 144.5139337266538178, -3662.585492863386662, 2245.937534930569200 ) ) ;
#6415=CARTESIAN_POINT ( 'NONE',  ( 13.89599138193900707, -3662.087915362755666, 2249.466105491610051 ) ) ;
#6416=CARTESIAN_POINT ( 'NONE',  ( 25.39999999999999858, -3578.860000000000127, 2244.547199999999975 ) ) ;
#6419=ADVANCED_FACE ( 'NONE', ( #9326 ), #14714, .F. ) ;
#6422=CARTESIAN_POINT ( 'NONE',  ( 9.653865685812997199, -3581.600845684150045, 2246.629994766630261 ) ) ;
#6423=CARTESIAN_POINT ( 'NONE',  ( 15.54461496037964174, -3659.404891253186179, 2250.142101673399793 ) ) ;
#6426=AXIS2_PLACEMENT_3D ( 'NONE', #2083, #1962, #17897 ) ;
#6428=ORIENTED_EDGE ( 'NONE', *, *, #12670, .F. ) ;
#6434=DIRECTION ( 'NONE',  ( 0.000000000000000000, 0.000000000000000000, -1.000000000000000000 ) ) ;
#6435=DIRECTION ( 'NONE',  ( 0.000000000000000000, 0.000000000000000000, -1.000000000000000000 ) ) ;
#6438=DIRECTION ( 'NONE',  ( -1.000000000000000000, 0.000000000000000000, 0.000000000000000000 ) ) ;
#6439=ADVANCED_FACE ( 'NONE', ( #4044 ), #7449, .F. ) ;
#6443=CARTESIAN_POINT ( 'NONE',  ( 7.327249423652832050, -3657.550365826240522, 2246.178457032339793 ) ) ;
#6447=CARTESIAN_POINT ( 'NONE',  ( 47.95519999999999783, -3670.300000000000182, 2261.869999999999891 ) ) ;
#6448=CARTESIAN_POINT ( 'NONE',  ( 10.37279685983138400, -3657.868421124709130, 2249.105504558603570 ) ) ;
#6449=ORIENTED_EDGE ( 'NONE', *, *, #7240, .T. ) ;
#6450=ORIENTED_EDGE ( 'NONE', *, *, #20754, .F. ) ;
#6451=CARTESIAN_POINT ( 'NONE',  ( 134.0869790975583840, -3580.606330659021751, 2245.129232553249949 ) ) ;
#6455=ORIENTED_EDGE ( 'NONE', *, *, #19921, .T. ) ;
#6456=DIRECTION ( 'NONE',  ( 1.000000000000000000, 0.000000000000000000, 8.741913579725999495E-14 ) ) ;
#6457=CARTESIAN_POINT ( 'NONE',  ( 10.57279766787198838, -3577.605992114683886, 2249.945558813966727 ) ) ;
#6459=CARTESIAN_POINT ( 'NONE',  ( 141.8303725231117198, -3581.380460283721277, 2248.711714140399636 ) ) ;
#6460=AXIS2_PLACEMENT_3D ( 'NONE', #13832, #10189, #22603 ) ;
#6462=AXIS2_PLACEMENT_3D ( 'NONE', #3950, #14391, #14278 ) ;
#6467=CARTESIAN_POINT ( 'NONE',  ( 133.9850000806000025, -3659.390917837453344, 2244.645117375718655 ) ) ;
#6468=ORIENTED_EDGE ( 'NONE', *, *, #7737, .T. ) ;
#6469=CIRCLE ( 'NONE', #1590, 2.844799999999994444 ) ;
#6472=VERTEX_POINT ( 'NONE', #21857 ) ;
#6477=DIRECTION ( 'NONE',  ( 0.000000000000000000, -1.000000000000000000, 0.000000000000000000 ) ) ;
#6482=AXIS2_PLACEMENT_3D ( 'NONE', #15184, #18685, #2634 ) ;
#6487=TOROIDAL_SURFACE ( 'NONE', #130, 3.606799999998999695, 0.7620000000000000107 ) ;
#6489=DIRECTION ( 'NONE',  ( 0.000000000000000000, 1.000000000000000000, 0.000000000000000000 ) ) ;
#6490=DIRECTION ( 'NONE',  ( 1.224646799147353207E-16, 1.000000000000000000, -0.000000000000000000 ) ) ;
#6491=CARTESIAN_POINT ( 'NONE',  ( 28.24479999999899604, -3568.700000000000273, 2259.837999999999738 ) ) ;
#6494=CARTESIAN_POINT ( 'NONE',  ( 141.7685968712770261, -3657.550763801919857, 2248.576229848027651 ) ) ;
#6497=DIRECTION ( 'NONE',  ( 0.000000000000000000, 0.000000000000000000, -1.000000000000000000 ) ) ;
#6500=AXIS2_PLACEMENT_3D ( 'NONE', #20919, #10668, #12077 ) ;
#6503=ADVANCED_FACE ( 'NONE', ( #21962 ), #13065, .F. ) ;
#6504=ORIENTED_EDGE ( 'NONE', *, *, #14174, .T. ) ;
#6505=ORIENTED_EDGE ( 'NONE', *, *, #17551, .F. ) ;
#6506=CARTESIAN_POINT ( 'NONE',  ( 76.20000000000000284, -3670.300000000000182, 2239.009999999999764 ) ) ;
#6507=EDGE_CURVE ( 'NONE', #20457, #4775, #7365, .T. ) ;
#6510=EDGE_CURVE ( 'NONE', #9415, #17185, #13731, .T. ) ;
#6511=VERTEX_POINT ( 'NONE', #21742 ) ;
#6514=CARTESIAN_POINT ( 'NONE',  ( 114.2999999999999972, -3644.899999999999636, 2239.009999999999764 ) ) ;
#6520=EDGE_CURVE ( 'NONE', #19601, #9977, #2867, .T. ) ;
#6521=DIRECTION ( 'NONE',  ( 0.000000000000000000, 0.000000000000000000, -1.000000000000000000 ) ) ;
#6524=CARTESIAN_POINT ( 'NONE',  ( 10.59346086370990037, -3581.406909921530314, 2248.659345565240528 ) ) ;
#6525=ORIENTED_EDGE ( 'NONE', *, *, #16030, .F. ) ;
#6526=DIRECTION ( 'NONE',  ( 1.000000000000000000, 0.000000000000000000, 0.000000000000000000 ) ) ;
#6527=ADVANCED_FACE ( 'NONE', ( #22070 ), #5697, .T. ) ;
#6529=FACE_BOUND ( 'NONE', #18193, .T. ) ;
#6530=ADVANCED_FACE ( 'NONE', ( #11074 ), #22701, .T. ) ;
#6531=CARTESIAN_POINT ( 'NONE',  ( 38.10000000000000142, -3594.099999999999909, 2259.837999999999738 ) ) ;
#6532=CARTESIAN_POINT ( 'NONE',  ( 145.3468180090523845, -3660.390156501248839, 2244.556611876515490 ) ) ;
#6537=DIRECTION ( 'NONE',  ( 1.000000000000000000, 0.000000000000000000, 0.000000000000000000 ) ) ;
#6541=CARTESIAN_POINT ( 'NONE',  ( 57.14999999999999858, -3568.700000000000273, 2250.236800000000130 ) ) ;
#6543=CARTESIAN_POINT ( 'NONE',  ( 15.53944468019864722, -3659.305298452004081, 2250.113581315974443 ) ) ;
#6545=ORIENTED_EDGE ( 'NONE', *, *, #20342, .T. ) ;
#6546=ORIENTED_EDGE ( 'NONE', *, *, #17095, .T. ) ;
#6547=CARTESIAN_POINT ( 'NONE',  ( 50.79999999999999716, -3670.300000000000182, 2239.771999999999935 ) ) ;
#6548=ORIENTED_EDGE ( 'NONE', *, *, #21107, .F. ) ;
#6555=B_SPLINE_CURVE_WITH_KNOTS ( 'NONE', 3,
 ( #15875, #15521, #6982, #19393 ),
 .UNSPECIFIED., .F., .F.,
 ( 4, 4 ),
 ( 0.000000000000000000, 1.000000000000000000 ),
 .UNSPECIFIED. ) ;
#6558=VECTOR ( 'NONE', #1392, 1000.000000000000000 ) ;
#6559=DIRECTION ( 'NONE',  ( 9.756599977372053330E-14, 0.000000000000000000, -1.000000000000000000 ) ) ;
#6560=CIRCLE ( 'NONE', #11407, 0.7619999999999294005 ) ;
#6561=CARTESIAN_POINT ( 'NONE',  ( 137.6199520187697090, -3577.554138631957812, 2249.919443248165862 ) ) ;
#6564=DIRECTION ( 'NONE',  ( 0.000000000000000000, 0.000000000000000000, -1.000000000000000000 ) ) ;
#6567=FACE_OUTER_BOUND ( 'NONE', #19224, .T. ) ;
#6569=ORIENTED_EDGE ( 'NONE', *, *, #18147, .T. ) ;
#6571=TOROIDAL_SURFACE ( 'NONE', #20406, 3.606799999999999784, 0.7620000000000000107 ) ;
#6572=AXIS2_PLACEMENT_3D ( 'NONE', #13822, #8660, #1390 ) ;
#6574=AXIS2_PLACEMENT_3D ( 'NONE', #6310, #8286, #22446 ) ;
#6575=CARTESIAN_POINT ( 'NONE',  ( 35.25520000000000209, -3644.899999999999636, 2239.771999999999935 ) ) ;
#6577=CARTESIAN_POINT ( 'NONE',  ( 72.59320000000001016, -3670.300000000000182, 2239.009999999999764 ) ) ;
#6581=ORIENTED_EDGE ( 'NONE', *, *, #15729, .T. ) ;
#6582=CARTESIAN_POINT ( 'NONE',  ( 131.7716230377726561, -3695.598599741984799, 2259.827559975022723 ) ) ;
#6585=CARTESIAN_POINT ( 'NONE',  ( 14.50824192230427201, -3581.691173654184695, 2247.673267903098349 ) ) ;
#6587=CARTESIAN_POINT ( 'NONE',  ( 134.0238007392231623, -3658.840387854182609, 2244.861395050478677 ) ) ;
#6591=DIRECTION ( 'NONE',  ( 0.000000000000000000, 1.000000000000000000, 0.000000000000000000 ) ) ;
#6594=EDGE_CURVE ( 'NONE', #8860, #10297, #20780, .T. ) ;
#6596=AXIS2_PLACEMENT_3D ( 'NONE', #21206, #5152, #6684 ) ;
#6597=ORIENTED_EDGE ( 'NONE', *, *, #17435, .F. ) ;
#6600=CARTESIAN_POINT ( 'NONE',  ( 114.2999999999999972, -3644.899999999999636, 2259.837999999999738 ) ) ;
#6605=CARTESIAN_POINT ( 'NONE',  ( 133.9850000806000025, -3659.504501929000071, 2244.618659328000376 ) ) ;
#6606=ORIENTED_EDGE ( 'NONE', *, *, #15595, .F. ) ;
#6607=LINE ( 'NONE', #1657, #10972 ) ;
#6610=CIRCLE ( 'NONE', #14075, 0.7619999999999987894 ) ;
#6615=DIRECTION ( 'NONE',  ( 0.000000000000000000, 0.000000000000000000, 1.000000000000000000 ) ) ;
#6618=CIRCLE ( 'NONE', #21565, 3.606799999999001027 ) ;
#6619=CARTESIAN_POINT ( 'NONE',  ( 141.6144402965059896, -3657.400733319522260, 2248.159976633087354 ) ) ;
#6620=VECTOR ( 'NONE', #22330, 1000.000000000000000 ) ;
#6622=CARTESIAN_POINT ( 'NONE',  ( 137.0608862933557077, -3543.814512435404595, 2255.525687528578146 ) ) ;
#6624=CARTESIAN_POINT ( 'NONE',  ( 4.707381495575098995, -3695.655085019853232, 2259.667485322372613 ) ) ;
#6627=VERTEX_POINT ( 'NONE', #1202 ) ;
#6628=EDGE_LOOP ( 'NONE', ( #6910, #18605, #6109, #6855 ) ) ;
#6631=CIRCLE ( 'NONE', #9611, 2.844800000000001550 ) ;
#6633=ORIENTED_EDGE ( 'NONE', *, *, #4147, .T. ) ;
#6634=CARTESIAN_POINT ( 'NONE',  ( 21.79320000000099711, -3568.700000000000273, 2260.600000000000364 ) ) ;
#6637=CARTESIAN_POINT ( 'NONE',  ( 17.68024974314568354, -3576.692299003124390, 2245.542863885450970 ) ) ;
#6642=VERTEX_POINT ( 'NONE', #22183 ) ;
#6643=DIRECTION ( 'NONE',  ( -1.000000000000000000, 0.000000000000000000, 0.000000000000000000 ) ) ;
#6645=CARTESIAN_POINT ( 'NONE',  ( 10.34642913787651075, -3581.093266999223033, 2249.155114352099645 ) ) ;
#6646=ADVANCED_FACE ( 'NONE', ( #974 ), #15607, .T. ) ;
#6649=ORIENTED_EDGE ( 'NONE', *, *, #3183, .T. ) ;
#6650=CARTESIAN_POINT ( 'NONE',  ( 97.99320000000000164, -3568.700000000000273, 2259.837999999999738 ) ) ;
#6651=EDGE_CURVE ( 'NONE', #15032, #10096, #18275, .T. ) ;
#6654=CARTESIAN_POINT ( 'NONE',  ( 145.3761492408112872, -3660.170703703051913, 2244.547341334182875 ) ) ;
#6656=CARTESIAN_POINT ( 'NONE',  ( 11.08609301964814264, -3661.848501376024615, 2249.666901776545728 ) ) ;
#6657=CARTESIAN_POINT ( 'NONE',  ( 147.3229993024389728, -3544.409801988681920, 2260.592426251218058 ) ) ;
#6660=PLANE ( 'NONE',  #8825 ) ;
#6661=AXIS2_PLACEMENT_3D ( 'NONE', #10657, #3736, #5275 ) ;
#6662=CARTESIAN_POINT ( 'NONE',  ( 136.8791170170333089, -3659.931058367113565, 2250.236800312005471 ) ) ;
#6663=CARTESIAN_POINT ( 'NONE',  ( 14.51094036875449866, -3657.306545957249909, 2246.963123837074363 ) ) ;
#6665=VERTEX_POINT ( 'NONE', #11627 ) ;
#6667=AXIS2_PLACEMENT_3D ( 'NONE', #21736, #12832, #11070 ) ;
#6668=CIRCLE ( 'NONE', #21704, 1.240967364599221412 ) ;
#6670=ORIENTED_EDGE ( 'NONE', *, *, #5876, .F. ) ;
#6673=DIRECTION ( 'NONE',  ( 0.000000000000000000, 0.000000000000000000, 1.000000000000000000 ) ) ;
#6674=EDGE_CURVE ( 'NONE', #22687, #11227, #3997, .T. ) ;
#6675=CARTESIAN_POINT ( 'NONE',  ( 25.39999999999999858, -3670.300000000000182, 2239.771999999999935 ) ) ;
#6677=EDGE_CURVE ( 'NONE', #11227, #12638, #8485, .T. ) ;
#6680=CARTESIAN_POINT ( 'NONE',  ( 60.65520000000000067, -3594.099999999999909, 2259.837999999999738 ) ) ;
#6681=AXIS2_PLACEMENT_3D ( 'NONE', #17253, #1194, #21875 ) ;
#6682=CARTESIAN_POINT ( 'NONE',  ( 57.14999999999999858, -3670.300000000000182, 2247.392000000000280 ) ) ;
#6684=DIRECTION ( 'NONE',  ( -1.000000000000000000, 0.000000000000000000, 0.000000000000000000 ) ) ;
#6686=EDGE_LOOP ( 'NONE', ( #19813, #16796, #16391, #8720, #15678, #5613, #15869, #15023, #14698 ) ) ;
#6687=DIRECTION ( 'NONE',  ( 0.000000000000000000, 0.000000000000000000, -1.000000000000000000 ) ) ;
#6688=CARTESIAN_POINT ( 'NONE',  ( 10.29010022044823458, -3657.993389994380777, 2249.258804498657810 ) ) ;
#6691=CARTESIAN_POINT ( 'NONE',  ( 134.2892388165611521, -3581.334923857996728, 2245.989158447333466 ) ) ;
#6697=ORIENTED_EDGE ( 'NONE', *, *, #22559, .T. ) ;
#6698=CARTESIAN_POINT ( 'NONE',  ( 131.9612844717763664, -3695.249961889823680, 2260.302094140601184 ) ) ;
#6700=CARTESIAN_POINT ( 'NONE',  ( 9.855200000000998273, -3579.494999999999891, 2256.063560000000052 ) ) ;
#6701=CARTESIAN_POINT ( 'NONE',  ( 15.41923444567002655, -3580.331984414333419, 2249.826959883762356 ) ) ;
#6702=CARTESIAN_POINT ( 'NONE',  ( 0.000000000000000000, -3578.860000000000127, 2243.277199999999993 ) ) ;
#6713=VERTEX_POINT ( 'NONE', #3545 ) ;
#6714=DIRECTION ( 'NONE',  ( 1.000000000000000000, 0.000000000000000000, 0.000000000000000000 ) ) ;
#6718=CARTESIAN_POINT ( 'NONE',  ( 9.855200000000680305, -3659.053785370519563, 2256.063559999999597 ) ) ;
#6719=DIRECTION ( 'NONE',  ( 0.000000000000000000, 0.000000000000000000, -1.000000000000000000 ) ) ;
#6722=EDGE_CURVE ( 'NONE', #13045, #6818, #10232, .T. ) ;
#6725=FACE_OUTER_BOUND ( 'NONE', #19973, .T. ) ;
#6726=DIRECTION ( 'NONE',  ( 0.000000000000000000, 0.000000000000000000, -1.000000000000000000 ) ) ;
#6728=TOROIDAL_SURFACE ( 'NONE', #11552, 3.606799999998999695, 0.7620000000000000107 ) ;
#6729=CARTESIAN_POINT ( 'NONE',  ( 142.3063350412433863, -3658.362045441383543, 2249.614643222462746 ) ) ;
#6732=EDGE_CURVE ( 'NONE', #6472, #12668, #9971, .T. ) ;
#6735=CIRCLE ( 'NONE', #17573, 0.7619999999999987894 ) ;
#6738=ORIENTED_EDGE ( 'NONE', *, *, #21279, .F. ) ;
#6740=CARTESIAN_POINT ( 'NONE',  ( 25.39999999999999858, -3670.300000000000182, 2239.771999999999935 ) ) ;
#6741=CYLINDRICAL_SURFACE ( 'NONE', #8038, 2.844799999999994444 ) ;
#6742=CARTESIAN_POINT ( 'NONE',  ( 132.3005794017000198, -3544.570000000000164, 2260.390449568000349 ) ) ;
#6743=ORIENTED_EDGE ( 'NONE', *, *, #9705, .T. ) ;
#6744=DIRECTION ( 'NONE',  ( -1.000000000000000000, 0.000000000000000000, 0.000000000000000000 ) ) ;
#6746=FACE_OUTER_BOUND ( 'NONE', #14983, .T. ) ;
#6749=VERTEX_POINT ( 'NONE', #5201 ) ;
#6755=CARTESIAN_POINT ( 'NONE',  ( 10.84069775277338010, -3581.649407856291873, 2246.804666700250891 ) ) ;
#6756=DIRECTION ( 'NONE',  ( 0.000000000000000000, 0.000000000000000000, -1.000000000000000000 ) ) ;
#6758=B_SPLINE_CURVE_WITH_KNOTS ( 'NONE', 3,
 ( #7688, #14733, #21980, #7353, #20124, #5718, #13076, #10976, #4171, #14385, #11315, #21533, #12850, #3943, #2196, #1957, #18122, #203, #20007, #9226, #11098, #5602, #18465, #5489, #9340, #16475, #4057, #2418, #14505, #16706, #7574, #7237, #19779, #3706, #11205, #10860, #2080, #18010, #9112, #12734, #19889, #16366, #319, #20456, #16814, #15071 ),
 .UNSPECIFIED., .F., .F.,
 ( 4, 2, 2, 1, 2, 2, 2, 2, 1, 1, 1, 1, 2, 2, 2, 2, 2, 1, 2, 2, 2, 2, 1, 1, 2, 2, 4 ),
 ( 0.000000000000000000, 0.1250000000022165880, 0.1875000000033248126, 0.2187500000036660674, 0.2343750000038365700, 0.2500000000040070725, 0.3750000000057552296, 0.4375000000064863115, 0.4687500000069002026, 0.4843750000070696782, 0.4921875000073470119, 0.4960937500074050766, 0.4980468750074055206, 0.5000000000074059647, 0.5625000000084945384, 0.5937500000090564223, 0.6093750000094169117, 0.6171875000095971009, 0.6210937500096163078, 0.6250000000096355146, 0.6875000000104954934, 0.7187500000108046905, 0.7343750000108574261, 0.7421875000107768239, 0.7460937500105744302, 0.7500000000103719255, 1.000000000000000000 ),
 .UNSPECIFIED. ) ;
#6762=AXIS2_PLACEMENT_3D ( 'NONE', #10686, #9165, #2136 ) ;
#6764=CARTESIAN_POINT ( 'NONE',  ( 144.8796679668512297, -3661.919754677027413, 2245.172503498299648 ) ) ;
#6768=CARTESIAN_POINT ( 'NONE',  ( 151.4000000000000057, -3544.570000000000164, 2239.039032635400417 ) ) ;
#6769=VERTEX_POINT ( 'NONE', #10585 ) ;
#6776=VERTEX_POINT ( 'NONE', #14343 ) ;
#6778=VERTEX_POINT ( 'NONE', #4961 ) ;
#6779=ORIENTED_EDGE ( 'NONE', *, *, #8454, .T. ) ;
#6790=FACE_OUTER_BOUND ( 'NONE', #14550, .T. ) ;
#6796=DIRECTION ( 'NONE',  ( 0.7249994335945011414, 6.337882393832011514E-14, -0.6887494619146010688 ) ) ;
#6797=CARTESIAN_POINT ( 'NONE',  ( 10.83541561206130055, -3657.356279649904991, 2247.981293899261800 ) ) ;
#6802=CARTESIAN_POINT ( 'NONE',  ( 132.3005794017000198, -3694.430000000000291, 2260.390449568000349 ) ) ;
#6804=ORIENTED_EDGE ( 'NONE', *, *, #20754, .T. ) ;
#6806=CARTESIAN_POINT ( 'NONE',  ( 95.25000000000000000, -3544.570000000000164, 2247.392000000000280 ) ) ;
#6808=DIRECTION ( 'NONE',  ( -1.000000000000000000, 0.000000000000000000, 0.000000000000000000 ) ) ;
#6809=ORIENTED_EDGE ( 'NONE', *, *, #9579, .F. ) ;
#6814=CARTESIAN_POINT ( 'NONE',  ( 134.0389477936680294, -3658.715683113317937, 2244.927055122274851 ) ) ;
#6815=AXIS2_PLACEMENT_3D ( 'NONE', #17676, #1624, #15349 ) ;
#6816=EDGE_CURVE ( 'NONE', #2094, #17500, #18855, .T. ) ;
#6818=VERTEX_POINT ( 'NONE', #15140 ) ;
#6819=CARTESIAN_POINT ( 'NONE',  ( 15.28726622823146819, -3695.066554908766193, 2255.655515827249928 ) ) ;
#6821=ORIENTED_EDGE ( 'NONE', *, *, #18090, .F. ) ;
#6822=DIRECTION ( 'NONE',  ( 1.000000000000000000, 0.000000000000000000, 0.000000000000000000 ) ) ;
#6823=VECTOR ( 'NONE', #10956, 1000.000000000000000 ) ;
#6825=ORIENTED_EDGE ( 'NONE', *, *, #9965, .F. ) ;
#6826=ORIENTED_EDGE ( 'NONE', *, *, #10259, .F. ) ;
#6827=SPHERICAL_SURFACE ( 'NONE', #3050, 1.270000000000000018 ) ;
#6828=CIRCLE ( 'NONE', #15801, 2.844800000000091700 ) ;
#6830=CIRCLE ( 'NONE', #5717, 4.114799999999974034 ) ;
#6833=CIRCLE ( 'NONE', #3827, 3.606800000000000228 ) ;
#6834=DIRECTION ( 'NONE',  ( 0.000000000000000000, 0.000000000000000000, -1.000000000000000000 ) ) ;
#6839=EDGE_CURVE ( 'NONE', #6888, #6776, #8497, .T. ) ;
#6842=CARTESIAN_POINT ( 'NONE',  ( 145.4149999999999920, -3659.504999999999654, 2239.771999999999935 ) ) ;
#6843=CARTESIAN_POINT ( 'NONE',  ( 18.38430049721045023, -3580.087277414933851, 2244.825193658544322 ) ) ;
#6844=CIRCLE ( 'NONE', #8358, 2.844799999999994444 ) ;
#6845=CARTESIAN_POINT ( 'NONE',  ( 142.0919336763783463, -3657.965060599514345, 2249.225720191686378 ) ) ;
#6853=ADVANCED_FACE ( 'NONE', ( #11725 ), #22384, .T. ) ;
#6855=ORIENTED_EDGE ( 'NONE', *, *, #16169, .T. ) ;
#6856=ORIENTED_EDGE ( 'NONE', *, *, #3988, .F. ) ;
#6861=VERTEX_POINT ( 'NONE', #4465 ) ;
#6865=AXIS2_PLACEMENT_3D ( 'NONE', #3327, #5220, #8381 ) ;
#6866=CARTESIAN_POINT ( 'NONE',  ( 20.34169023495000062, -3694.797466901999996, 2260.545675974999995 ) ) ;
#6869=EDGE_CURVE ( 'NONE', #11706, #9059, #9855, .T. ) ;
#6871=CYLINDRICAL_SURFACE ( 'NONE', #18753, 2.844799999999994444 ) ;
#6873=ORIENTED_EDGE ( 'NONE', *, *, #17358, .T. ) ;
#6874=CARTESIAN_POINT ( 'NONE',  ( 127.0000000000000000, -3660.140000000000327, 2247.392000000000280 ) ) ;
#6876=AXIS2_PLACEMENT_3D ( 'NONE', #7161, #12545, #10785 ) ;
#6877=CARTESIAN_POINT ( 'NONE',  ( 25.39999999999999858, -3619.500000000000000, 2239.009999999999764 ) ) ;
#6878=CIRCLE ( 'NONE', #12101, 0.7619999999999987894 ) ;
#6880=CARTESIAN_POINT ( 'NONE',  ( 145.3795747169000094, -3578.859731361000286, 2244.547525601999951 ) ) ;
#6885=CARTESIAN_POINT ( 'NONE',  ( 11.35172555707717379, -3662.010415283757993, 2249.535724915129322 ) ) ;
#6886=AXIS2_PLACEMENT_3D ( 'NONE', #6912, #14377, #11699 ) ;
#6888=VERTEX_POINT ( 'NONE', #15482 ) ;
#6890=CARTESIAN_POINT ( 'NONE',  ( 25.39999999999999858, -3670.300000000000182, 2260.600000000000364 ) ) ;
#6891=CARTESIAN_POINT ( 'NONE',  ( 133.9850000019999925, -3579.494756921999851, 2244.617465693000213 ) ) ;
#6892=CARTESIAN_POINT ( 'NONE',  ( 15.36939286637828239, -3658.521437840668568, 2249.731612551223861 ) ) ;
#6895=ORIENTED_EDGE ( 'NONE', *, *, #19465, .F. ) ;
#6896=DIRECTION ( 'NONE',  ( 0.000000000000000000, 0.000000000000000000, -1.000000000000000000 ) ) ;
#6897=EDGE_LOOP ( 'NONE', ( #17896, #680, #20630, #14488 ) ) ;
#6900=CYLINDRICAL_SURFACE ( 'NONE', #10570, 2.844799999998995244 ) ;
#6901=CARTESIAN_POINT ( 'NONE',  ( 139.6999999999999886, -3579.494999999999891, 2246.630000000000109 ) ) ;
#6903=DIRECTION ( 'NONE',  ( -0.6887494619146540265, 0.000000000000000000, -0.7249994335944508483 ) ) ;
#6904=CARTESIAN_POINT ( 'NONE',  ( 17.45971744210237020, -3576.330750010172778, 2246.087203520595722 ) ) ;
#6907=AXIS2_PLACEMENT_3D ( 'NONE', #10555, #3514, #1291 ) ;
#6910=ORIENTED_EDGE ( 'NONE', *, *, #21012, .F. ) ;
#6911=CARTESIAN_POINT ( 'NONE',  ( 151.1299999999999955, -3544.570000000000164, 2240.279999999999745 ) ) ;
#6912=CARTESIAN_POINT ( 'NONE',  ( 25.39999999999999858, -3619.500000000000000, 2259.837999999999738 ) ) ;
#6913=ORIENTED_EDGE ( 'NONE', *, *, #7130, .T. ) ;
#6914=CARTESIAN_POINT ( 'NONE',  ( 134.3329781701244485, -3581.459545042529953, 2246.234697007345403 ) ) ;
#6915=ORIENTED_EDGE ( 'NONE', *, *, #7235, .F. ) ;
#6918=FACE_OUTER_BOUND ( 'NONE', #17028, .T. ) ;
#6919=ORIENTED_EDGE ( 'NONE', *, *, #20017, .T. ) ;
#6921=AXIS2_PLACEMENT_3D ( 'NONE', #6531, #12025, #3111 ) ;
#6926=DIRECTION ( 'NONE',  ( 0.000000000000000000, 0.000000000000000000, -1.000000000000000000 ) ) ;
#6927=CARTESIAN_POINT ( 'NONE',  ( 15.54480025890283912, -3579.679221764684371, 2250.122839540403220 ) ) ;
#6929=CARTESIAN_POINT ( 'NONE',  ( 151.1299999999999955, -3544.570000000000164, 2260.600000000000364 ) ) ;
#6933=ORIENTED_EDGE ( 'NONE', *, *, #2131, .T. ) ;
#6937=ORIENTED_EDGE ( 'NONE', *, *, #23112, .T. ) ;
#6938=VECTOR ( 'NONE', #2599, 1000.000000000000000 ) ;
#6939=DIRECTION ( 'NONE',  ( 0.000000000000000000, 0.000000000000000000, 1.000000000000000000 ) ) ;
#6942=CARTESIAN_POINT ( 'NONE',  ( 21.79320000000099711, -3670.300000000000182, 2260.600000000000364 ) ) ;
#6943=VECTOR ( 'NONE', #14667, 1000.000000000000000 ) ;
#6946=EDGE_LOOP ( 'NONE', ( #9523, #22595, #12694, #3543 ) ) ;
#6949=LINE ( 'NONE', #17478, #9821 ) ;
#6950=DIRECTION ( 'NONE',  ( 0.000000000000000000, 0.000000000000000000, -1.000000000000000000 ) ) ;
#6951=DIRECTION ( 'NONE',  ( -0.000000000000000000, -1.000000000000000000, -0.000000000000000000 ) ) ;
#6952=EDGE_CURVE ( 'NONE', #9982, #4022, #16306, .T. ) ;
#6956=CARTESIAN_POINT ( 'NONE',  ( 10.01182667074545840, -3695.327183877031530, 2255.402926848606057 ) ) ;
#6960=CARTESIAN_POINT ( 'NONE',  ( 137.3255051320594475, -3657.938320579140509, 2249.193689002128849 ) ) ;
#6962=ORIENTED_EDGE ( 'NONE', *, *, #634, .T. ) ;
#6973=ORIENTED_EDGE ( 'NONE', *, *, #3222, .F. ) ;
#6974=CARTESIAN_POINT ( 'NONE',  ( 142.5448000000000093, -3659.504999999999654, 2256.063560000000052 ) ) ;
#6977=DIRECTION ( 'NONE',  ( 1.000000000000000000, 0.000000000000000000, 0.000000000000000000 ) ) ;
#6978=AXIS2_PLACEMENT_3D ( 'NONE', #17642, #3465, #1592 ) ;
#6979=CARTESIAN_POINT ( 'NONE',  ( 136.8551999999999964, -3659.504999999999654, 2256.063560000000052 ) ) ;
#6981=AXIS2_PLACEMENT_3D ( 'NONE', #5979, #11465, #20596 ) ;
#6982=CARTESIAN_POINT ( 'NONE',  ( 136.8552000000001669, -3579.946214629432689, 2256.063560000000052 ) ) ;
#6983=FACE_BOUND ( 'NONE', #13974, .T. ) ;
#6991=FACE_OUTER_BOUND ( 'NONE', #18654, .T. ) ;
#6992=CARTESIAN_POINT ( 'NONE',  ( 10.73432012640060584, -3581.551840941039700, 2248.313564088525254 ) ) ;
#6993=DIRECTION ( 'NONE',  ( 0.000000000000000000, 0.000000000000000000, -1.000000000000000000 ) ) ;
#6998=CARTESIAN_POINT ( 'NONE',  ( 144.5542768966436711, -3576.478798223026388, 2245.835328353847217 ) ) ;
#6999=AXIS2_PLACEMENT_3D ( 'NONE', #9375, #20158, #3983 ) ;
#7000=CARTESIAN_POINT ( 'NONE',  ( 116.8400000000000034, -3544.570000000000164, 2247.392000000000280 ) ) ;
#7001=AXIS2_PLACEMENT_3D ( 'NONE', #9877, #8597, #13871 ) ;
#7002=CARTESIAN_POINT ( 'NONE',  ( 11.38813178685436256, -3662.029528285001106, 2249.518792719746671 ) ) ;
#7003=EDGE_CURVE ( 'NONE', #16212, #10141, #12134, .T. ) ;
#7007=ORIENTED_EDGE ( 'NONE', *, *, #21990, .T. ) ;
#7008=ADVANCED_FACE ( 'NONE', ( #3404 ), #20992, .F. ) ;
#7011=CARTESIAN_POINT ( 'NONE',  ( 141.6126943346999951, -3657.399161235000520, 2246.630000000000109 ) ) ;
#7012=CARTESIAN_POINT ( 'NONE',  ( 14.88809329571305540, -3657.686607509436271, 2248.833042055603983 ) ) ;
#7013=CARTESIAN_POINT ( 'NONE',  ( 137.1293686148364372, -3694.866442831601034, 2255.697303097024360 ) ) ;
#7017=CARTESIAN_POINT ( 'NONE',  ( 10.58927397074967125, -3577.587572210373310, 2249.936439182378308 ) ) ;
#7020=AXIS2_PLACEMENT_3D ( 'NONE', #21657, #9122, #5376 ) ;
#7021=DIRECTION ( 'NONE',  ( -1.000000000000000000, 0.000000000000000000, 0.000000000000000000 ) ) ;
#7023=EDGE_CURVE ( 'NONE', #5223, #6224, #10322, .T. ) ;
#7024=ADVANCED_FACE ( 'NONE', ( #3516 ), #21343, .T. ) ;
#7026=CARTESIAN_POINT ( 'NONE',  ( 137.7875023037999824, -3581.600928630999988, 2246.630000000000109 ) ) ;
#7029=DIRECTION ( 'NONE',  ( -0.8928571428573600643, 0.4503400076038009403, 0.000000000000000000 ) ) ;
#7031=ORIENTED_EDGE ( 'NONE', *, *, #2566, .F. ) ;
#7035=CARTESIAN_POINT ( 'NONE',  ( 35.56000000000000227, -3694.430000000000291, 2244.547199999999975 ) ) ;
#7037=DIRECTION ( 'NONE',  ( 0.000000000000000000, 0.000000000000000000, -1.000000000000000000 ) ) ;
#7039=AXIS2_PLACEMENT_3D ( 'NONE', #5195, #14335, #3425 ) ;
#7041=CARTESIAN_POINT ( 'NONE',  ( 142.2650752003752075, -3694.826579461697293, 2255.711168198594351 ) ) ;
#7042=CARTESIAN_POINT ( 'NONE',  ( 142.5354141679999884, -3659.800641111999539, 2250.222551630000453 ) ) ;
#7043=VERTEX_POINT ( 'NONE', #21231 ) ;
#7044=DIRECTION ( 'NONE',  ( -1.224646799147353207E-16, 1.000000000000000000, 0.000000000000000000 ) ) ;
#7046=CARTESIAN_POINT ( 'NONE',  ( 135.0886139726999886, -3576.119152860999748, 2246.630000000000109 ) ) ;
#7049=CARTESIAN_POINT ( 'NONE',  ( 15.54479999999999862, -3659.504999999999654, 2256.063560000000052 ) ) ;
#7050=CARTESIAN_POINT ( 'NONE',  ( 14.87406578659674494, -3581.330107240630696, 2248.804283326418044 ) ) ;
#7055=ORIENTED_EDGE ( 'NONE', *, *, #21693, .T. ) ;
#7056=CARTESIAN_POINT ( 'NONE',  ( 15.38582118512052510, -3695.321318630521546, 2255.408746714442714 ) ) ;
#7057=ORIENTED_EDGE ( 'NONE', *, *, #18375, .T. ) ;
#7058=CARTESIAN_POINT ( 'NONE',  ( 12.69999999999999929, -3579.494999999999891, 2246.630000000000109 ) ) ;
#7059=CARTESIAN_POINT ( 'NONE',  ( 136.8551999999999964, -3659.504999999999654, 2256.063560000000052 ) ) ;
#7062=FACE_OUTER_BOUND ( 'NONE', #17925, .T. ) ;
#7066=VERTEX_POINT ( 'NONE', #13959 ) ;
#7067=DIRECTION ( 'NONE',  ( 0.8068916933301631955, -0.5906994119133536225, 0.000000000000000000 ) ) ;
#7070=CARTESIAN_POINT ( 'NONE',  ( 1.270000000000000018, -3544.570000000000164, 2260.600000000000364 ) ) ;
#7074=CARTESIAN_POINT ( 'NONE',  ( 10.00637276908404161, -3695.340677396607134, 2255.389249077402383 ) ) ;
#7076=CARTESIAN_POINT ( 'NONE',  ( 137.6322476998775244, -3657.550994620480651, 2248.571276128920090 ) ) ;
#7077=ORIENTED_EDGE ( 'NONE', *, *, #3420, .F. ) ;
#7081=EDGE_LOOP ( 'NONE', ( #8950, #17446, #19795, #11793 ) ) ;
#7082=VERTEX_POINT ( 'NONE', #16406 ) ;
#7087=LINE ( 'NONE', #15987, #5289 ) ;
#7089=DIRECTION ( 'NONE',  ( 0.000000000000000000, 0.000000000000000000, -1.000000000000000000 ) ) ;
#7090=ORIENTED_EDGE ( 'NONE', *, *, #4131, .F. ) ;
#7093=FACE_BOUND ( 'NONE', #1675, .T. ) ;
#7094=TOROIDAL_SURFACE ( 'NONE', #347, 3.606799999999999784, 0.7620000000000000107 ) ;
#7098=EDGE_CURVE ( 'NONE', #6749, #9068, #2345, .T. ) ;
#7102=CARTESIAN_POINT ( 'NONE',  ( 38.10000000000000142, -3594.099999999999909, 2260.600000000000364 ) ) ;
#7103=VERTEX_POINT ( 'NONE', #19814 ) ;
#7108=FACE_BOUND ( 'NONE', #1988, .T. ) ;
#7110=CARTESIAN_POINT ( 'NONE',  ( 131.7757523116999891, -3694.430000000000291, 2260.600000000000364 ) ) ;
#7112=CARTESIAN_POINT ( 'NONE',  ( 15.54478274857000031, -3659.508323119057422, 2250.165783369506698 ) ) ;
#7113=EDGE_LOOP ( 'NONE', ( #13730, #15749, #22251, #311 ) ) ;
#7116=DIRECTION ( 'NONE',  ( 0.000000000000000000, 0.000000000000000000, -1.000000000000000000 ) ) ;
#7117=CARTESIAN_POINT ( 'NONE',  ( 15.29891559246383359, -3658.345264832731573, 2249.601063626551877 ) ) ;
#7118=CARTESIAN_POINT ( 'NONE',  ( 6.222999999999998977, -3659.504999999999654, 2239.009999999999764 ) ) ;
#7119=ORIENTED_EDGE ( 'NONE', *, *, #12108, .T. ) ;
#7120=CARTESIAN_POINT ( 'NONE',  ( 47.95519999999999783, -3619.500000000000000, 2261.869999999999891 ) ) ;
#7121=VERTEX_POINT ( 'NONE', #17926 ) ;
#7126=DIRECTION ( 'NONE',  ( -0.7249994335944036639, 0.000000000000000000, -0.6887494619147036534 ) ) ;
#7130=EDGE_CURVE ( 'NONE', #14558, #1923, #109, .T. ) ;
#7131=DIRECTION ( 'NONE',  ( 1.000000000000000000, 0.000000000000000000, 0.000000000000000000 ) ) ;
#7133=CARTESIAN_POINT ( 'NONE',  ( 88.90000000000000568, -3594.099999999999909, 2239.771999999999935 ) ) ;
#7134=DIRECTION ( 'NONE',  ( 0.000000000000000000, 0.000000000000000000, -1.000000000000000000 ) ) ;
#7138=EDGE_LOOP ( 'NONE', ( #4656, #9586, #11733, #457 ) ) ;
#7143=ORIENTED_EDGE ( 'NONE', *, *, #6288, .T. ) ;
#7146=B_SPLINE_CURVE_WITH_KNOTS ( 'NONE', 3,
 ( #1127, #13799, #6662, #10272 ),
 .UNSPECIFIED., .F., .F.,
 ( 4, 4 ),
 ( 0.000000000000000000, 1.000000000000000000 ),
 .UNSPECIFIED. ) ;
#7150=CARTESIAN_POINT ( 'NONE',  ( 137.2652732970130103, -3580.966343291408975, 2249.304226862355335 ) ) ;
#7154=EDGE_CURVE ( 'NONE', #1906, #20621, #18808, .T. ) ;
#7155=DIRECTION ( 'NONE',  ( 0.000000000000000000, 0.000000000000000000, 1.000000000000000000 ) ) ;
#7159=DIRECTION ( 'NONE',  ( 0.000000000000000000, 0.000000000000000000, -1.000000000000000000 ) ) ;
#7160=DIRECTION ( 'NONE',  ( -1.000000000000000000, 0.000000000000000000, 0.000000000000000000 ) ) ;
#7161=CARTESIAN_POINT ( 'NONE',  ( 50.79999999999999716, -3568.700000000000273, 2260.600000000000364 ) ) ;
#7162=ORIENTED_EDGE ( 'NONE', *, *, #2549, .T. ) ;
#7163=CARTESIAN_POINT ( 'NONE',  ( 134.2038178129721757, -3577.928751811623897, 2244.703885868194902 ) ) ;
#7164=VECTOR ( 'NONE', #15063, 1000.000000000000000 ) ;
#7167=DIRECTION ( 'NONE',  ( 1.000000000000000000, 0.000000000000000000, 0.000000000000000000 ) ) ;
#7177=CARTESIAN_POINT ( 'NONE',  ( 35.56000000000032202, -3670.300000000000182, 2244.547199999999975 ) ) ;
#7179=CARTESIAN_POINT ( 'NONE',  ( 38.10000000000000142, -3644.899999999999636, 2261.869999999999891 ) ) ;
#7181=AXIS2_PLACEMENT_3D ( 'NONE', #12815, #21838, #5795 ) ;
#7183=DIRECTION ( 'NONE',  ( 0.000000000000000000, 1.000000000000000000, 0.000000000000000000 ) ) ;
#7185=CARTESIAN_POINT ( 'NONE',  ( 18.19932492755376785, -3581.050454778146559, 2245.576347937810169 ) ) ;
#7186=CARTESIAN_POINT ( 'NONE',  ( 137.8886907543135294, -3657.311334042124145, 2247.705354153496955 ) ) ;
#7190=ORIENTED_EDGE ( 'NONE', *, *, #13086, .T. ) ;
#7195=DIRECTION ( 'NONE',  ( -0.8068916933244314471, 0.5906994119211830263, 0.000000000000000000 ) ) ;
#7197=VERTEX_POINT ( 'NONE', #16124 ) ;
#7200=LINE ( 'NONE', #3785, #9167 ) ;
#7201=LINE ( 'NONE', #14354, #5200 ) ;
#7203=DIRECTION ( 'NONE',  ( 1.000000000000000000, 0.000000000000000000, 0.000000000000000000 ) ) ;
#7204=FACE_BOUND ( 'NONE', #10927, .T. ) ;
#7209=ORIENTED_EDGE ( 'NONE', *, *, #20562, .T. ) ;
#7210=CARTESIAN_POINT ( 'NONE',  ( 0.000000000000000000, -3544.570000000000164, 2240.279999999999745 ) ) ;
#7211=VERTEX_POINT ( 'NONE', #72 ) ;
#7212=VECTOR ( 'NONE', #9810, 1000.000000000000000 ) ;
#7214=AXIS2_PLACEMENT_3D ( 'NONE', #19317, #22703, #10519 ) ;
#7216=DIRECTION ( 'NONE',  ( -0.8928571428573600643, 0.4503400076038009403, 0.000000000000000000 ) ) ;
#7217=CARTESIAN_POINT ( 'NONE',  ( 1.270000000000000018, -3544.570000000000164, 2240.279999999999745 ) ) ;
#7221=EDGE_CURVE ( 'NONE', #5432, #22780, #9323, .T. ) ;
#7224=DIRECTION ( 'NONE',  ( 0.000000000000000000, 0.000000000000000000, 1.000000000000000000 ) ) ;
#7225=TOROIDAL_SURFACE ( 'NONE', #3091, 3.606799999999999784, 0.7620000000000000107 ) ;
#7227=ADVANCED_FACE ( 'NONE', ( #1588, #5233, #8749, #7108, #1709 ), #15895, .T. ) ;
#7228=CARTESIAN_POINT ( 'NONE',  ( 139.6999999999999886, -3659.504999999999654, 2272.030000000000200 ) ) ;
#7229=VERTEX_POINT ( 'NONE', #17759 ) ;
#7233=CARTESIAN_POINT ( 'NONE',  ( 95.25000000000000000, -3568.700000000000273, 2247.392000000000280 ) ) ;
#7235=EDGE_CURVE ( 'NONE', #16346, #12999, #12613, .T. ) ;
#7236=CARTESIAN_POINT ( 'NONE',  ( 136.9962509646508408, -3695.367664692730159, 2255.363857416606152 ) ) ;
#7237=CARTESIAN_POINT ( 'NONE',  ( 7.657922162452776682, -3576.804516390709068, 2245.425293001298087 ) ) ;
#7239=DIRECTION ( 'NONE',  ( 1.000000000000000000, 0.000000000000000000, 0.000000000000000000 ) ) ;
#7240=EDGE_CURVE ( 'NONE', #4452, #15095, #8102, .T. ) ;
#7241=CARTESIAN_POINT ( 'NONE',  ( 10.00638266403440824, -3543.659322602310112, 2255.389245125443722 ) ) ;
#7244=EDGE_CURVE ( 'NONE', #14593, #21665, #1825, .T. ) ;
#7247=CARTESIAN_POINT ( 'NONE',  ( 18.01287425285000410, -3657.399152860999493, 2246.630000000000109 ) ) ;
#7248=TOROIDAL_SURFACE ( 'NONE', #21460, 3.606799999998999695, 0.7620000000000000107 ) ;
#7250=AXIS2_PLACEMENT_3D ( 'NONE', #21115, #3294, #17232 ) ;
#7251=ORIENTED_EDGE ( 'NONE', *, *, #9705, .F. ) ;
#7252=DIRECTION ( 'NONE',  ( 1.000000000000000000, 0.000000000000000000, 0.000000000000000000 ) ) ;
#7255=ADVANCED_FACE ( 'NONE', ( #6725 ), #15960, .T. ) ;
#7257=ORIENTED_EDGE ( 'NONE', *, *, #19810, .T. ) ;
#7258=AXIS2_PLACEMENT_3D ( 'NONE', #4625, #19160, #2983 ) ;
#7260=CARTESIAN_POINT ( 'NONE',  ( 127.0000000000000000, -3670.300000000000182, 2259.837999999999738 ) ) ;
#7261=DIRECTION ( 'NONE',  ( 1.000000000000000000, 0.000000000000000000, 0.000000000000000000 ) ) ;
#7262=ORIENTED_EDGE ( 'NONE', *, *, #9679, .F. ) ;
#7263=CARTESIAN_POINT ( 'NONE',  ( 137.7193482430640188, -3581.537511303820338, 2248.354490200028522 ) ) ;
#7265=CARTESIAN_POINT ( 'NONE',  ( 57.14999999999999858, -3568.700000000000273, 2247.392000000000280 ) ) ;
#7269=AXIS2_PLACEMENT_3D ( 'NONE', #5732, #7705, #9352 ) ;
#7273=CARTESIAN_POINT ( 'NONE',  ( 141.8684782314425661, -3577.653504331623481, 2249.968348377236453 ) ) ;
#7274=ORIENTED_EDGE ( 'NONE', *, *, #11726, .F. ) ;
#7275=CARTESIAN_POINT ( 'NONE',  ( 134.4883907600942052, -3577.149724370994591, 2245.118708806262930 ) ) ;
#7277=VERTEX_POINT ( 'NONE', #19137 ) ;
#7278=DIRECTION ( 'NONE',  ( 0.9296367896517967466, -0.3684771896955098547, 0.000000000000000000 ) ) ;
#7280=EDGE_CURVE ( 'NONE', #13787, #22588, #21203, .T. ) ;
#7282=ORIENTED_EDGE ( 'NONE', *, *, #14046, .F. ) ;
#7283=EDGE_CURVE ( 'NONE', #22625, #15231, #912, .T. ) ;
#7288=TOROIDAL_SURFACE ( 'NONE', #5046, 3.606799999999999784, 0.7620000000000000107 ) ;
#7292=AXIS2_PLACEMENT_3D ( 'NONE', #2408, #19152, #19036 ) ;
#7293=DIRECTION ( 'NONE',  ( 0.000000000000000000, 0.000000000000000000, -1.000000000000000000 ) ) ;
#7295=LINE ( 'NONE', #11157, #18238 ) ;
#7298=CARTESIAN_POINT ( 'NONE',  ( 9.998047855982495236, -3695.360820975178285, 2255.368362556688680 ) ) ;
#7305=TOROIDAL_SURFACE ( 'NONE', #8423, 3.606799999999999784, 0.7620000000000000107 ) ;
#7306=CARTESIAN_POINT ( 'NONE',  ( 138.1068462689100613, -3661.863663675439511, 2249.656022096149172 ) ) ;
#7308=EDGE_LOOP ( 'NONE', ( #10163, #21900 ) ) ;
#7310=ORIENTED_EDGE ( 'NONE', *, *, #14118, .F. ) ;
#7312=DIRECTION ( 'NONE',  ( 1.000000000000000000, 0.000000000000000000, -1.224646799147353207E-16 ) ) ;
#7313=VERTEX_POINT ( 'NONE', #4952 ) ;
#7314=EDGE_LOOP ( 'NONE', ( #17990, #11604 ) ) ;
#7317=CARTESIAN_POINT ( 'NONE',  ( 38.10000000000000142, -3594.099999999999909, 2239.771999999999935 ) ) ;
#7318=CARTESIAN_POINT ( 'NONE',  ( 9.855200000000680305, -3659.956214629480201, 2256.063559999999597 ) ) ;
#7323=TOROIDAL_SURFACE ( 'NONE', #16658, 4.114799999999999791, 1.270000000000000018 ) ;
#7324=TOROIDAL_SURFACE ( 'NONE', #5827, 3.606799999999999784, 0.7620000000000000107 ) ;
#7327=CIRCLE ( 'NONE', #10306, 3.606800000000000228 ) ;
#7330=FACE_OUTER_BOUND ( 'NONE', #17216, .T. ) ;
#7332=DIRECTION ( 'NONE',  ( 0.000000000000000000, 0.000000000000000000, 1.000000000000000000 ) ) ;
#7333=DIRECTION ( 'NONE',  ( 0.000000000000000000, 0.000000000000000000, -1.000000000000000000 ) ) ;
#7335=DIRECTION ( 'NONE',  ( -1.000000000000000000, 0.000000000000000000, 0.000000000000000000 ) ) ;
#7336=CIRCLE ( 'NONE', #234, 0.7619999999999987894 ) ;
#7340=CARTESIAN_POINT ( 'NONE',  ( 95.25000000000000000, -3568.700000000000273, 2247.392000000000280 ) ) ;
#7342=CARTESIAN_POINT ( 'NONE',  ( 18.12143270522780014, -3657.696842364385247, 2245.934643265300110 ) ) ;
#7344=CARTESIAN_POINT ( 'NONE',  ( 147.5630070217191587, -3695.514947978554574, 2259.991585417506030 ) ) ;
#7346=AXIS2_PLACEMENT_3D ( 'NONE', #306, #5929, #7557 ) ;
#7349=CARTESIAN_POINT ( 'NONE',  ( 104.4447999999999865, -3568.700000000000273, 2261.869999999999891 ) ) ;
#7350=DIRECTION ( 'NONE',  ( -1.000000000000000000, 0.000000000000000000, 0.000000000000000000 ) ) ;
#7351=CARTESIAN_POINT ( 'NONE',  ( 137.1440299052392788, -3694.748620250294152, 2255.734053407186821 ) ) ;
#7353=CARTESIAN_POINT ( 'NONE',  ( 7.099392720542782698, -3578.355474235146630, 2244.591332851781317 ) ) ;
#7354=EDGE_LOOP ( 'NONE', ( #10703, #16971, #17607, #13518 ) ) ;
#7356=ADVANCED_FACE ( 'NONE', ( #11872 ), #2960, .T. ) ;
#7362=CARTESIAN_POINT ( 'NONE',  ( 8.088613972650000150, -3576.119152860999748, 2246.630000000000109 ) ) ;
#7363=CIRCLE ( 'NONE', #15967, 2.844800000000001550 ) ;
#7364=FACE_OUTER_BOUND ( 'NONE', #15481, .T. ) ;
#7365=CIRCLE ( 'NONE', #7747, 0.7619999999999294005 ) ;
#7366=CARTESIAN_POINT ( 'NONE',  ( 104.4447999999999865, -3619.500000000000000, 2261.869999999999891 ) ) ;
#7370=CARTESIAN_POINT ( 'NONE',  ( 17.31138602737999932, -3662.880847139000252, 2246.630000000000109 ) ) ;
#7373=DIRECTION ( 'NONE',  ( -1.000000000000000000, 0.000000000000000000, 0.000000000000000000 ) ) ;
#7374=TOROIDAL_SURFACE ( 'NONE', #22321, 3.606799999998999695, 0.7620000000000000107 ) ;
#7376=CARTESIAN_POINT ( 'NONE',  ( 142.3712313342016671, -3695.282573427255556, 2255.445352725234443 ) ) ;
#7377=CARTESIAN_POINT ( 'NONE',  ( 50.79999999999999716, -3568.700000000000273, 2239.009999999999764 ) ) ;
#7378=EDGE_LOOP ( 'NONE', ( #3825, #9875, #9330, #6334, #1208, #12467, #6913, #6546, #240, #41 ) ) ;
#7379=EDGE_CURVE ( 'NONE', #18081, #19890, #13625, .T. ) ;
#7380=CARTESIAN_POINT ( 'NONE',  ( 137.0759654552891220, -3580.596807917107526, 2249.647026203515452 ) ) ;
#7381=ORIENTED_EDGE ( 'NONE', *, *, #5841, .T. ) ;
#7383=EDGE_CURVE ( 'NONE', #5536, #5355, #16686, .T. ) ;
#7386=LINE ( 'NONE', #15825, #3726 ) ;
#7391=AXIS2_PLACEMENT_3D ( 'NONE', #17806, #1870, #14300 ) ;
#7392=CARTESIAN_POINT ( 'NONE',  ( 139.0044331210974349, -3576.736148240796410, 2249.284738289012694 ) ) ;
#7395=CARTESIAN_POINT ( 'NONE',  ( 134.8618250315517457, -3576.452994732182106, 2245.875428656681379 ) ) ;
#7397=AXIS2_PLACEMENT_3D ( 'NONE', #12072, #20747, #22492 ) ;
#7398=DIRECTION ( 'NONE',  ( 1.000000000000000000, 0.000000000000000000, 0.000000000000000000 ) ) ;
#7399=ORIENTED_EDGE ( 'NONE', *, *, #10943, .T. ) ;
#7401=PLANE ( 'NONE',  #1612 ) ;
#7403=DIRECTION ( 'NONE',  ( 0.000000000000000000, 0.000000000000000000, -1.000000000000000000 ) ) ;
#7404=CARTESIAN_POINT ( 'NONE',  ( 47.95519999999999783, -3568.700000000000273, 2259.837999999999738 ) ) ;
#7413=CIRCLE ( 'NONE', #11159, 0.7619999999999294005 ) ;
#7415=CARTESIAN_POINT ( 'NONE',  ( 20.52663054042999846, -3694.556024844999683, 2260.595783923999988 ) ) ;
#7416=CYLINDRICAL_SURFACE ( 'NONE', #15054, 1.269999999999882334 ) ;
#7417=ORIENTED_EDGE ( 'NONE', *, *, #17236, .T. ) ;
#7419=ADVANCED_FACE ( 'NONE', ( #6375 ), #11985, .T. ) ;
#7420=CARTESIAN_POINT ( 'NONE',  ( 137.8759894827288690, -3657.321687586756980, 2247.788848385796882 ) ) ;
#7422=ORIENTED_EDGE ( 'NONE', *, *, #3359, .F. ) ;
#7423=CARTESIAN_POINT ( 'NONE',  ( 137.8845111942463859, -3661.695361931427669, 2249.774021930013532 ) ) ;
#7426=EDGE_CURVE ( 'NONE', #9059, #16839, #8361, .T. ) ;
#7427=ORIENTED_EDGE ( 'NONE', *, *, #22581, .F. ) ;
#7428=DIRECTION ( 'NONE',  ( 0.000000000000000000, 0.000000000000000000, -1.000000000000000000 ) ) ;
#7436=EDGE_CURVE ( 'NONE', #16534, #22243, #10729, .T. ) ;
#7437=CARTESIAN_POINT ( 'NONE',  ( 25.39999999999999858, -3660.140000000000327, 2244.547199999999975 ) ) ;
#7439=FACE_OUTER_BOUND ( 'NONE', #19422, .T. ) ;
#7441=CARTESIAN_POINT ( 'NONE',  ( 131.8826930129156096, -3543.564485452164263, 2260.105821329443188 ) ) ;
#7443=CIRCLE ( 'NONE', #1063, 2.873832635400752622 ) ;
#7445=EDGE_CURVE ( 'NONE', #11629, #12173, #4825, .T. ) ;
#7446=CARTESIAN_POINT ( 'NONE',  ( 8.062487613724396596, -3662.845158696698491, 2246.501631804077533 ) ) ;
#7449=PLANE ( 'NONE',  #260 ) ;
#7451=DIRECTION ( 'NONE',  ( 0.000000000000000000, 0.000000000000000000, 1.000000000000000000 ) ) ;
#7452=DIRECTION ( 'NONE',  ( 0.000000000000000000, 0.000000000000000000, -1.000000000000000000 ) ) ;
#7453=DIRECTION ( 'NONE',  ( 0.000000000000000000, 0.000000000000000000, -1.000000000000000000 ) ) ;
#7455=CARTESIAN_POINT ( 'NONE',  ( 38.10000000000000142, -3594.099999999999909, 2239.009999999999764 ) ) ;
#7456=LINE ( 'NONE', #18342, #21873 ) ;
#7457=AXIS2_PLACEMENT_3D ( 'NONE', #13529, #22889, #17037 ) ;
#7460=DIRECTION ( 'NONE',  ( 0.000000000000000000, 0.000000000000000000, -1.000000000000000000 ) ) ;
#7461=CARTESIAN_POINT ( 'NONE',  ( 142.4686189914979764, -3543.507962130772285, 2255.201647170270917 ) ) ;
#7462=DIRECTION ( 'NONE',  ( -1.000000000000000000, 0.000000000000000000, 0.000000000000000000 ) ) ;
#7467=LINE ( 'NONE', #12394, #21996 ) ;
#7470=CARTESIAN_POINT ( 'NONE',  ( 38.10000000000000142, -3644.899999999999636, 2261.869999999999891 ) ) ;
#7471=AXIS2_PLACEMENT_3D ( 'NONE', #7892, #16671, #4034 ) ;
#7473=DIRECTION ( 'NONE',  ( 1.000000000000000000, 0.000000000000000000, 0.000000000000000000 ) ) ;
#7481=AXIS2_PLACEMENT_3D ( 'NONE', #18967, #22464, #17311 ) ;
#7483=CARTESIAN_POINT ( 'NONE',  ( 142.2400000001210572, -3694.509865590614027, 2255.773999999871648 ) ) ;
#7484=CARTESIAN_POINT ( 'NONE',  ( 1.270000000000000018, -3578.860000000000127, 2247.392000000000280 ) ) ;
#7487=CARTESIAN_POINT ( 'NONE',  ( 137.2263574705312976, -3580.899882066081773, 2249.375081330945704 ) ) ;
#7488=ORIENTED_EDGE ( 'NONE', *, *, #8688, .T. ) ;
#7493=AXIS2_PLACEMENT_3D ( 'NONE', #21074, #16033, #14042 ) ;
#7494=DIRECTION ( 'NONE',  ( 0.000000000000000000, -1.000000000000000000, 0.000000000000000000 ) ) ;
#7495=DIRECTION ( 'NONE',  ( -0.000000000000000000, -1.000000000000000000, -0.000000000000000000 ) ) ;
#7497=CARTESIAN_POINT ( 'NONE',  ( 138.4977950649703473, -3576.916347349343141, 2249.469419588345772 ) ) ;
#7498=ORIENTED_EDGE ( 'NONE', *, *, #14013, .T. ) ;
#7501=EDGE_CURVE ( 'NONE', #17371, #2232, #18928, .T. ) ;
#7502=ORIENTED_EDGE ( 'NONE', *, *, #11710, .F. ) ;
#7509=EDGE_LOOP ( 'NONE', ( #16209, #5661, #16386, #10276 ) ) ;
#7513=CARTESIAN_POINT ( 'NONE',  ( 0.000000000000000000, -3694.430000000000291, 2259.329999999999927 ) ) ;
#7515=EDGE_CURVE ( 'NONE', #9827, #14706, #12680, .T. ) ;
#7517=CARTESIAN_POINT ( 'NONE',  ( 141.5301317845463132, -3581.673074589064527, 2246.966346727968357 ) ) ;
#7523=CARTESIAN_POINT ( 'NONE',  ( 34.49320000000000164, -3644.899999999999636, 2239.009999999999764 ) ) ;
#7524=EDGE_LOOP ( 'NONE', ( #9493, #5812, #15911, #12581, #13745, #1009, #14284, #16014 ) ) ;
#7525=CARTESIAN_POINT ( 'NONE',  ( 18.26645764376696235, -3580.789478182200128, 2245.301509789812371 ) ) ;
#7527=CARTESIAN_POINT ( 'NONE',  ( 136.8709027835478196, -3659.159706171275047, 2250.069058248565852 ) ) ;
#7528=AXIS2_PLACEMENT_3D ( 'NONE', #10121, #15290, #7912 ) ;
#7529=ORIENTED_EDGE ( 'NONE', *, *, #5391, .T. ) ;
#7530=ORIENTED_EDGE ( 'NONE', *, *, #8131, .F. ) ;
#7531=CARTESIAN_POINT ( 'NONE',  ( 141.2546625656592028, -3661.887891249280983, 2249.636713181481355 ) ) ;
#7534=ADVANCED_FACE ( 'NONE', ( #8473 ), #5069, .F. ) ;
#7541=EDGE_LOOP ( 'NONE', ( #6428, #8632, #4442, #3896, #18945, #6525, #9014, #21457 ) ) ;
#7545=DIRECTION ( 'NONE',  ( 1.000000000000000000, 0.000000000000000000, 0.000000000000000000 ) ) ;
#7550=ORIENTED_EDGE ( 'NONE', *, *, #22002, .T. ) ;
#7554=ORIENTED_EDGE ( 'NONE', *, *, #7515, .F. ) ;
#7555=CIRCLE ( 'NONE', #4190, 0.7619999999999987894 ) ;
#7556=EDGE_CURVE ( 'NONE', #19621, #7999, #1507, .T. ) ;
#7557=DIRECTION ( 'NONE',  ( 0.000000000000000000, 0.000000000000000000, 1.000000000000000000 ) ) ;
#7558=AXIS2_PLACEMENT_3D ( 'NONE', #10887, #17913, #3851 ) ;
#7561=CARTESIAN_POINT ( 'NONE',  ( 76.20000000000000284, -3670.300000000000182, 2260.600000000000364 ) ) ;
#7562=FACE_OUTER_BOUND ( 'NONE', #3515, .T. ) ;
#7564=CARTESIAN_POINT ( 'NONE',  ( 147.6473427028456342, -3695.618941227105097, 2259.780211612979656 ) ) ;
#7569=FACE_OUTER_BOUND ( 'NONE', #22857, .T. ) ;
#7570=CARTESIAN_POINT ( 'NONE',  ( 101.5999999999999943, -3670.300000000000182, 2259.837999999999738 ) ) ;
#7571=CARTESIAN_POINT ( 'NONE',  ( 86.05520000000001346, -3644.899999999999636, 2259.837999999999738 ) ) ;
#7573=AXIS2_PLACEMENT_3D ( 'NONE', #12044, #19197, #22812 ) ;
#7574=CARTESIAN_POINT ( 'NONE',  ( 7.652106483500662470, -3576.815456713399726, 2245.413922136005567 ) ) ;
#7575=VERTEX_POINT ( 'NONE', #17592 ) ;
#7579=CARTESIAN_POINT ( 'NONE',  ( 95.25000000000000000, -3544.570000000000164, 2244.547199999999975 ) ) ;
#7591=CARTESIAN_POINT ( 'NONE',  ( 104.4447999999999865, -3568.700000000000273, 2239.771999999999935 ) ) ;
#7593=CARTESIAN_POINT ( 'NONE',  ( 63.50000000000000000, -3644.899999999999636, 2261.869999999999891 ) ) ;
#7595=ORIENTED_EDGE ( 'NONE', *, *, #6952, .T. ) ;
#7597=CARTESIAN_POINT ( 'NONE',  ( 1.270000000000000018, -3694.430000000000291, 2260.600000000000364 ) ) ;
#7599=ORIENTED_EDGE ( 'NONE', *, *, #6312, .F. ) ;
#7602=ORIENTED_EDGE ( 'NONE', *, *, #16443, .T. ) ;
#7604=CARTESIAN_POINT ( 'NONE',  ( 145.1404951596551598, -3581.245129387089946, 2245.841260533643435 ) ) ;
#7608=DIRECTION ( 'NONE',  ( 0.000000000000000000, 0.000000000000000000, -1.000000000000000000 ) ) ;
#7610=CARTESIAN_POINT ( 'NONE',  ( 141.1391456164894578, -3577.040607256482417, 2249.579133306534459 ) ) ;
#7612=CIRCLE ( 'NONE', #15113, 3.606800000000000228 ) ;
#7617=CARTESIAN_POINT ( 'NONE',  ( 15.54897409013627652, -3543.400907226583968, 2255.000090470922714 ) ) ;
#7618=VECTOR ( 'NONE', #1884, 1000.000000000000000 ) ;
#7621=CARTESIAN_POINT ( 'NONE',  ( 137.7875023037999824, -3581.600928630999988, 2246.630000000000109 ) ) ;
#7622=ORIENTED_EDGE ( 'NONE', *, *, #337, .T. ) ;
#7625=CARTESIAN_POINT ( 'NONE',  ( 13.65342256834697388, -3576.814163253546212, 2249.368886017665773 ) ) ;
#7628=ORIENTED_EDGE ( 'NONE', *, *, #14422, .F. ) ;
#7630=AXIS2_PLACEMENT_3D ( 'NONE', #21317, #8428, #13931 ) ;
#7635=CARTESIAN_POINT ( 'NONE',  ( 18.12991818266355892, -3581.277546170917049, 2245.892459010505263 ) ) ;
#7638=SPHERICAL_SURFACE ( 'NONE', #6108, 1.270000000000000018 ) ;
#7639=VERTEX_POINT ( 'NONE', #1784 ) ;
#7640=CARTESIAN_POINT ( 'NONE',  ( 141.4267388136501040, -3661.765907838432668, 2249.726436259035381 ) ) ;
#7642=ORIENTED_EDGE ( 'NONE', *, *, #956, .F. ) ;
#7646=FACE_OUTER_BOUND ( 'NONE', #45, .T. ) ;
#7652=DIRECTION ( 'NONE',  ( 0.000000000000000000, 0.000000000000000000, -1.000000000000000000 ) ) ;
#7653=FACE_BOUND ( 'NONE', #16045, .T. ) ;
#7654=CARTESIAN_POINT ( 'NONE',  ( 7.179586105935542584, -3580.969250050631217, 2245.481136081417844 ) ) ;
#7655=CARTESIAN_POINT ( 'NONE',  ( 63.50000000000000000, -3594.099999999999909, 2239.771999999999935 ) ) ;
#7657=EDGE_CURVE ( 'NONE', #15883, #8860, #16842, .T. ) ;
#7659=VECTOR ( 'NONE', #8492, 1000.000000000000000 ) ;
#7660=AXIS2_PLACEMENT_3D ( 'NONE', #21801, #14549, #2464 ) ;
#7663=ADVANCED_FACE ( 'NONE', ( #12906 ), #3418, .T. ) ;
#7665=CARTESIAN_POINT ( 'NONE',  ( 142.4715777200796367, -3658.856899883896403, 2249.932665716038628 ) ) ;
#7667=AXIS2_PLACEMENT_3D ( 'NONE', #15989, #4029, #5679 ) ;
#7668=ORIENTED_EDGE ( 'NONE', *, *, #5162, .T. ) ;
#7670=DIRECTION ( 'NONE',  ( -1.000000000000000000, 0.000000000000000000, 0.000000000000000000 ) ) ;
#7673=CARTESIAN_POINT ( 'NONE',  ( 0.000000000000000000, -3660.140000000000327, 2247.392000000000280 ) ) ;
#7674=ORIENTED_EDGE ( 'NONE', *, *, #9106, .F. ) ;
#7675=CARTESIAN_POINT ( 'NONE',  ( 147.5973730189926982, -3543.437357047961086, 2259.905208148476504 ) ) ;
#7676=ORIENTED_EDGE ( 'NONE', *, *, #6510, .F. ) ;
#7678=ADVANCED_FACE ( 'NONE', ( #17709 ), #16074, .T. ) ;
#7681=VECTOR ( 'NONE', #13351, 1000.000000000000000 ) ;
#7683=TOROIDAL_SURFACE ( 'NONE', #9909, 6.477000000000000313, 0.7620000000000000107 ) ;
#7684=CARTESIAN_POINT ( 'NONE',  ( 12.69999999999999929, -3579.494999999999891, 2239.009999999999764 ) ) ;
#7686=DIRECTION ( 'NONE',  ( 0.000000000000000000, 1.000000000000000000, 0.000000000000000000 ) ) ;
#7688=CARTESIAN_POINT ( 'NONE',  ( 7.020348529275000082, -3578.860230781999689, 2244.548186305999934 ) ) ;
#7691=CARTESIAN_POINT ( 'NONE',  ( 145.1681434097811234, -3657.843844258350600, 2245.707489631754015 ) ) ;
#7692=CARTESIAN_POINT ( 'NONE',  ( 15.24000000000000021, -3660.786127253999894, 2255.774000000000342 ) ) ;
#7694=AXIS2_PLACEMENT_3D ( 'NONE', #4646, #10037, #17180 ) ;
#7697=CARTESIAN_POINT ( 'NONE',  ( 25.39999999999999858, -3670.300000000000182, 2259.837999999999738 ) ) ;
#7701=EDGE_CURVE ( 'NONE', #3136, #6642, #20438, .T. ) ;
#7703=EDGE_CURVE ( 'NONE', #22988, #10080, #9383, .T. ) ;
#7705=DIRECTION ( 'NONE',  ( -1.000000000000000000, 0.000000000000000000, 0.000000000000000000 ) ) ;
#7706=VERTEX_POINT ( 'NONE', #1601 ) ;
#7708=CARTESIAN_POINT ( 'NONE',  ( 14.51618957457999493, -3661.694864241059349, 2249.774377504978474 ) ) ;
#7709=DIRECTION ( 'NONE',  ( -1.000000000000000000, 0.000000000000000000, 0.000000000000000000 ) ) ;
#7710=ORIENTED_EDGE ( 'NONE', *, *, #14422, .T. ) ;
#7711=ADVANCED_FACE ( 'NONE', ( #8206 ), #5246, .F. ) ;
#7712=CARTESIAN_POINT ( 'NONE',  ( 9.653930614662758813, -3657.399154393335721, 2246.629994487922431 ) ) ;
#7716=AXIS2_PLACEMENT_3D ( 'NONE', #15527, #12478, #21387 ) ;
#7717=DIRECTION ( 'NONE',  ( 0.000000000000000000, 0.000000000000000000, -1.000000000000000000 ) ) ;
#7719=AXIS2_PLACEMENT_3D ( 'NONE', #15990, #1686, #17620 ) ;
#7720=VECTOR ( 'NONE', #15511, 1000.000000000000000 ) ;
#7726=CARTESIAN_POINT ( 'NONE',  ( 66.34479999999999222, -3644.899999999999636, 2239.771999999999935 ) ) ;
#7727=ORIENTED_EDGE ( 'NONE', *, *, #17551, .T. ) ;
#7728=B_SPLINE_CURVE_WITH_KNOTS ( 'NONE', 3,
 ( #18143, #7483, #16276, #19677, #3966, #7041, #11123, #21438, #12646, #5743, #9251, #14641, #21668, #7376, #1863, #19796, #12759, #16389, #9134, #14292, #14529, #14407, #18260, #9362, #12528, #5623, #21783, #19913, #111, #3850, #14183 ),
 .UNSPECIFIED., .F., .F.,
 ( 4, 2, 2, 2, 2, 2, 1, 2, 2, 2, 2, 1, 1, 2, 2, 2, 4 ),
 ( 0.000000000000000000, 0.1250000000011337598, 0.1875000000020345392, 0.2500000000029353187, 0.3750000000047304383, 0.4375000000053519411, 0.4687500000056163962, 0.4843750000059510175, 0.5000000000062856387, 0.6250000000045987658, 0.6875000000039348524, 0.7187500000033559822, 0.7343750000030726532, 0.7421875000030454528, 0.7500000000030181413, 0.8750000000015091262, 1.000000000000000000 ),
 .UNSPECIFIED. ) ;
#7730=SHAPE_REPRESENTATION ( 'Base Plate', ( #5611 ), #2239 ) ;
#7734=CARTESIAN_POINT ( 'NONE',  ( 18.34030854049733605, -3660.434275077790517, 2244.558523461154437 ) ) ;
#7735=CARTESIAN_POINT ( 'NONE',  ( 21.79320000000099711, -3670.300000000000182, 2239.771999999999935 ) ) ;
#7737=EDGE_CURVE ( 'NONE', #8199, #12626, #12757, .T. ) ;
#7738=CARTESIAN_POINT ( 'NONE',  ( 142.0475659686787822, -3577.885968673145271, 2250.065841773341617 ) ) ;
#7739=ORIENTED_EDGE ( 'NONE', *, *, #4489, .T. ) ;
#7740=AXIS2_PLACEMENT_3D ( 'NONE', #61, #12822, #20206 ) ;
#7742=DIRECTION ( 'NONE',  ( 0.000000000000000000, 0.000000000000000000, 1.000000000000000000 ) ) ;
#7743=VERTEX_POINT ( 'NONE', #22601 ) ;
#7744=DIRECTION ( 'NONE',  ( -1.000000000000000000, 0.000000000000000000, 0.000000000000000000 ) ) ;
#7746=CARTESIAN_POINT ( 'NONE',  ( 1.270000000000000018, -3544.570000000000164, 2240.279999999999745 ) ) ;
#7747=AXIS2_PLACEMENT_3D ( 'NONE', #9209, #18561, #16688 ) ;
#7749=AXIS2_PLACEMENT_3D ( 'NONE', #17287, #15544, #5001 ) ;
#7750=ORIENTED_EDGE ( 'NONE', *, *, #10002, .F. ) ;
#7751=B_SPLINE_CURVE_WITH_KNOTS ( 'NONE', 3,
 ( #9898, #876, #1230, #16819 ),
 .UNSPECIFIED., .F., .F.,
 ( 4, 4 ),
 ( 0.000000000000000000, 1.000000000000000000 ),
 .UNSPECIFIED. ) ;
#7753=LINE ( 'NONE', #813, #19693 ) ;
#7754=CARTESIAN_POINT ( 'NONE',  ( 13.59572439041964032, -3576.794808590030243, 2249.348515776098338 ) ) ;
#7755=DIRECTION ( 'NONE',  ( -5.197384013923000042E-14, -1.000000000000000000, 2.639941086436999774E-14 ) ) ;
#7757=CIRCLE ( 'NONE', #16729, 2.844800000000098361 ) ;
#7760=CIRCLE ( 'NONE', #7391, 4.114799999999974034 ) ;
#7763=CARTESIAN_POINT ( 'NONE',  ( 35.56000000000000227, -3670.300000000000182, 2247.392000000000280 ) ) ;
#7764=AXIS2_PLACEMENT_3D ( 'NONE', #6300, #19055, #11656 ) ;
#7765=AXIS2_PLACEMENT_3D ( 'NONE', #10579, #5426, #17715 ) ;
#7766=AXIS2_PLACEMENT_3D ( 'NONE', #16308, #19944, #20173 ) ;
#7768=CARTESIAN_POINT ( 'NONE',  ( 141.8096541925104077, -3661.413627425323284, 2249.935838938367851 ) ) ;
#7770=ORIENTED_EDGE ( 'NONE', *, *, #8941, .T. ) ;
#7771=ORIENTED_EDGE ( 'NONE', *, *, #18279, .T. ) ;
#7774=EDGE_CURVE ( 'NONE', #17371, #17962, #14639, .T. ) ;
#7776=CARTESIAN_POINT ( 'NONE',  ( 25.39999999999999858, -3568.700000000000273, 2239.771999999999935 ) ) ;
#7778=EDGE_LOOP ( 'NONE', ( #5318, #22918, #13917, #6937 ) ) ;
#7780=CARTESIAN_POINT ( 'NONE',  ( 7.223429647927347652, -3657.870544957902439, 2245.674539183268280 ) ) ;
#7782=DIRECTION ( 'NONE',  ( 0.000000000000000000, 0.000000000000000000, -1.000000000000000000 ) ) ;
#7783=CARTESIAN_POINT ( 'NONE',  ( 129.8447999999989975, -3568.700000000000273, 2239.771999999999935 ) ) ;
#7786=ORIENTED_EDGE ( 'NONE', *, *, #22096, .F. ) ;
#7788=CIRCLE ( 'NONE', #9282, 4.114799999999974034 ) ;
#7789=CARTESIAN_POINT ( 'NONE',  ( 127.0000000000000000, -3660.140000000000327, 2247.392000000000280 ) ) ;
#7791=CARTESIAN_POINT ( 'NONE',  ( 139.6999999999999886, -3659.504999999999654, 2239.009999999999764 ) ) ;
#7794=VERTEX_POINT ( 'NONE', #6577 ) ;
#7795=DIRECTION ( 'NONE',  ( 0.000000000000000000, 1.000000000000000000, 0.000000000000000000 ) ) ;
#7796=EDGE_LOOP ( 'NONE', ( #16489, #10920, #12529, #8960 ) ) ;
#7799=ORIENTED_EDGE ( 'NONE', *, *, #23017, .T. ) ;
#7805=EDGE_CURVE ( 'NONE', #11209, #8599, #15000, .T. ) ;
#7807=DIRECTION ( 'NONE',  ( 0.000000000000000000, -1.000000000000000000, 0.000000000000000000 ) ) ;
#7810=VERTEX_POINT ( 'NONE', #12503 ) ;
#7812=CARTESIAN_POINT ( 'NONE',  ( 54.40679999999999694, -3619.500000000000000, 2239.771999999999935 ) ) ;
#7815=CARTESIAN_POINT ( 'NONE',  ( 25.39999999999999858, -3578.860000000000127, 2250.236800000000130 ) ) ;
#7816=EDGE_CURVE ( 'NONE', #2568, #7197, #8880, .T. ) ;
#7819=DIRECTION ( 'NONE',  ( 1.000000000000000000, 0.000000000000000000, 0.000000000000000000 ) ) ;
#7821=AXIS2_PLACEMENT_3D ( 'NONE', #9074, #17974, #19742 ) ;
#7823=CARTESIAN_POINT ( 'NONE',  ( 14.97732264284127446, -3661.210416770012216, 2250.027943346653501 ) ) ;
#7825=ORIENTED_EDGE ( 'NONE', *, *, #988, .T. ) ;
#7827=EDGE_CURVE ( 'NONE', #11664, #10874, #6878, .T. ) ;
#7829=DIRECTION ( 'NONE',  ( 0.000000000000000000, 0.000000000000000000, -1.000000000000000000 ) ) ;
#7836=DIRECTION ( 'NONE',  ( 1.000000000000000000, 0.000000000000000000, 0.000000000000000000 ) ) ;
#7838=EDGE_LOOP ( 'NONE', ( #17049, #3505, #8526, #8471 ) ) ;
#7839=AXIS2_PLACEMENT_3D ( 'NONE', #7684, #18462, #9671 ) ;
#7841=PRODUCT_CONTEXT ( 'NONE', #19647, 'mechanical' ) ;
#7843=CARTESIAN_POINT ( 'NONE',  ( 17.44548393074270365, -3662.697233759483879, 2246.100251725204544 ) ) ;
#7844=CARTESIAN_POINT ( 'NONE',  ( 131.8733692468000243, -3544.443975433000105, 2260.595783961000052 ) ) ;
#7845=DIRECTION ( 'NONE',  ( 1.224646799147353207E-16, 1.000000000000000000, -0.000000000000000000 ) ) ;
#7849=AXIS2_PLACEMENT_3D ( 'NONE', #9024, #16286, #21570 ) ;
#7852=ORIENTED_EDGE ( 'NONE', *, *, #1235, .F. ) ;
#7855=VECTOR ( 'NONE', #2043, 1000.000000000000000 ) ;
#7857=ORIENTED_EDGE ( 'NONE', *, *, #11693, .F. ) ;
#7859=ORIENTED_EDGE ( 'NONE', *, *, #18021, .T. ) ;
#7862=VERTEX_POINT ( 'NONE', #14616 ) ;
#7865=CARTESIAN_POINT ( 'NONE',  ( 14.89507094893205519, -3577.685273219328337, 2249.982988182303870 ) ) ;
#7867=CARTESIAN_POINT ( 'NONE',  ( 141.8137592268451499, -3581.398919698233840, 2248.675269099207981 ) ) ;
#7873=DIRECTION ( 'NONE',  ( -1.000000000000000000, 0.000000000000000000, 0.000000000000000000 ) ) ;
#7877=ADVANCED_FACE ( 'NONE', ( #18234 ), #2736, .T. ) ;
#7879=EDGE_CURVE ( 'NONE', #4712, #3136, #542, .T. ) ;
#7884=CARTESIAN_POINT ( 'NONE',  ( 12.69999999999999929, -3659.504999999999654, 2239.771999999999935 ) ) ;
#7885=ORIENTED_EDGE ( 'NONE', *, *, #1108, .T. ) ;
#7888=CARTESIAN_POINT ( 'NONE',  ( 35.56000000000000227, -3568.700000000000273, 2247.392000000000280 ) ) ;
#7890=VERTEX_POINT ( 'NONE', #5834 ) ;
#7891=CARTESIAN_POINT ( 'NONE',  ( 7.155628190510333830, -3658.118427763718046, 2245.389413767294627 ) ) ;
#7892=CARTESIAN_POINT ( 'NONE',  ( 152.4000000000000057, -3695.699999999999818, 2239.009999999999764 ) ) ;
#7893=LINE ( 'NONE', #1074, #19960 ) ;
#7898=CARTESIAN_POINT ( 'NONE',  ( 142.5447969220999767, -3659.505006299999877, 2250.165025787000104 ) ) ;
#7902=ORIENTED_EDGE ( 'NONE', *, *, #12219, .T. ) ;
#7903=CARTESIAN_POINT ( 'NONE',  ( 137.0705190374700351, -3543.848287276122392, 2255.549776698934238 ) ) ;
#7910=ORIENTED_EDGE ( 'NONE', *, *, #21752, .T. ) ;
#7911=EDGE_LOOP ( 'NONE', ( #8852, #17855, #14794, #22893, #15404, #5877, #3733, #5210, #22182, #7710 ) ) ;
#7912=DIRECTION ( 'NONE',  ( 1.000000000000000000, 0.000000000000000000, 0.000000000000000000 ) ) ;
#7913=CARTESIAN_POINT ( 'NONE',  ( 127.0000000000000000, -3578.860000000000127, 2250.236800000000130 ) ) ;
#7916=CARTESIAN_POINT ( 'NONE',  ( 25.39999999999999858, -3568.700000000000273, 2239.771999999999935 ) ) ;
#7917=DIRECTION ( 'NONE',  ( 0.000000000000000000, 1.000000000000000000, 0.000000000000000000 ) ) ;
#7918=CARTESIAN_POINT ( 'NONE',  ( 20.66691620702998478, -3695.635001937071593, 2259.731083289085291 ) ) ;
#7923=AXIS2_PLACEMENT_3D ( 'NONE', #5554, #16200, #2023 ) ;
#7926=EDGE_CURVE ( 'NONE', #20430, #16634, #6758, .T. ) ;
#7927=CARTESIAN_POINT ( 'NONE',  ( 131.7757523116999891, -3544.570000000000164, 2260.600000000000364 ) ) ;
#7934=CARTESIAN_POINT ( 'NONE',  ( 134.2179335353430076, -3577.879693976099134, 2244.721041474473623 ) ) ;
#7937=CIRCLE ( 'NONE', #21038, 1.269999999999882334 ) ;
#7938=DIRECTION ( 'NONE',  ( 0.000000000000000000, -1.000000000000000000, 0.000000000000000000 ) ) ;
#7939=LINE ( 'NONE', #9910, #235 ) ;
#7942=AXIS2_PLACEMENT_3D ( 'NONE', #10802, #9045, #16646 ) ;
#7945=FACE_OUTER_BOUND ( 'NONE', #20148, .T. ) ;
#7946=VECTOR ( 'NONE', #21587, 1000.000000000000000 ) ;
#7947=DIRECTION ( 'NONE',  ( 0.000000000000000000, 0.000000000000000000, -1.000000000000000000 ) ) ;
#7954=CARTESIAN_POINT ( 'NONE',  ( 145.1299181802738758, -3581.277546178230750, 2245.892459022343701 ) ) ;
#7957=CARTESIAN_POINT ( 'NONE',  ( 145.4149999194000600, -3579.389963339004225, 2244.594906236255156 ) ) ;
#7958=CARTESIAN_POINT ( 'NONE',  ( 25.39999999999999858, -3619.500000000000000, 2239.771999999999935 ) ) ;
#7959=AXIS2_PLACEMENT_3D ( 'NONE', #13889, #8614, #10601 ) ;
#7960=EDGE_CURVE ( 'NONE', #6861, #5300, #22200, .T. ) ;
#7963=DIRECTION ( 'NONE',  ( 1.000000000000000000, 0.000000000000000000, 0.000000000000000000 ) ) ;
#7964=AXIS2_PLACEMENT_3D ( 'NONE', #19778, #3705, #7462 ) ;
#7965=DIRECTION ( 'NONE',  ( 0.000000000000000000, -1.000000000000000000, 0.000000000000000000 ) ) ;
#7969=ORIENTED_EDGE ( 'NONE', *, *, #12245, .F. ) ;
#7971=CARTESIAN_POINT ( 'NONE',  ( 10.90366342691393164, -3657.299102526176739, 2247.222754898936728 ) ) ;
#7975=ORIENTED_EDGE ( 'NONE', *, *, #2009, .F. ) ;
#7978=ORIENTED_EDGE ( 'NONE', *, *, #9825, .F. ) ;
#7979=CIRCLE ( 'NONE', #4983, 0.7619999999999987894 ) ;
#7980=FACE_OUTER_BOUND ( 'NONE', #15760, .T. ) ;
#7981=CARTESIAN_POINT ( 'NONE',  ( 14.71696921254339685, -3577.486687656909453, 2249.884401328558397 ) ) ;
#7983=CARTESIAN_POINT ( 'NONE',  ( 142.0870141205355992, -3581.042503004332502, 2249.216714460935691 ) ) ;
#7984=VERTEX_POINT ( 'NONE', #22312 ) ;
#7985=CARTESIAN_POINT ( 'NONE',  ( 50.79999999999999716, -3670.300000000000182, 2261.869999999999891 ) ) ;
#7989=AXIS2_PLACEMENT_3D ( 'NONE', #2230, #7495, #11014 ) ;
#7992=AXIS2_PLACEMENT_3D ( 'NONE', #5775, #487, #21593 ) ;
#7995=CIRCLE ( 'NONE', #16945, 2.844799999998998796 ) ;
#7996=ADVANCED_FACE ( 'NONE', ( #6168 ), #13304, .T. ) ;
#7999=VERTEX_POINT ( 'NONE', #13533 ) ;
#8001=CARTESIAN_POINT ( 'NONE',  ( 66.34479999999999222, -3594.099999999999909, 2261.869999999999891 ) ) ;
#8005=EDGE_CURVE ( 'NONE', #13997, #21361, #2716, .T. ) ;
#8012=EDGE_CURVE ( 'NONE', #6309, #2800, #18772, .T. ) ;
#8014=EDGE_CURVE ( 'NONE', #20229, #22764, #22553, .T. ) ;
#8016=CARTESIAN_POINT ( 'NONE',  ( 63.50000000000000000, -3594.099999999999909, 2239.771999999999935 ) ) ;
#8017=CARTESIAN_POINT ( 'NONE',  ( 59.89320000000000022, -3594.099999999999909, 2260.600000000000364 ) ) ;
#8021=CARTESIAN_POINT ( 'NONE',  ( 136.9723221135144797, -3543.579977981522461, 2255.303759353553687 ) ) ;
#8023=ORIENTED_EDGE ( 'NONE', *, *, #5931, .F. ) ;
#8026=VERTEX_POINT ( 'NONE', #21037 ) ;
#8027=VERTEX_POINT ( 'NONE', #1693 ) ;
#8028=DIRECTION ( 'NONE',  ( -0.6887494619146540265, 0.000000000000000000, -0.7249994335944508483 ) ) ;
#8032=CARTESIAN_POINT ( 'NONE',  ( 123.3932000000010021, -3619.500000000000000, 2260.600000000000364 ) ) ;
#8034=DIRECTION ( 'NONE',  ( 0.000000000000000000, 0.000000000000000000, 1.000000000000000000 ) ) ;
#8035=EDGE_LOOP ( 'NONE', ( #20051, #3522, #5640, #21614 ) ) ;
#8038=AXIS2_PLACEMENT_3D ( 'NONE', #1568, #13644, #8375 ) ;
#8039=CARTESIAN_POINT ( 'NONE',  ( 145.1018191042290084, -3657.638755556700744, 2246.035947349423623 ) ) ;
#8040=CARTESIAN_POINT ( 'NONE',  ( 9.862268097132236733, -3579.717233113928614, 2250.106397596277475 ) ) ;
#8041=CARTESIAN_POINT ( 'NONE',  ( 57.14999999999999858, -3544.570000000000164, 2247.392000000000280 ) ) ;
#8043=CARTESIAN_POINT ( 'NONE',  ( 28.24479999999899604, -3619.500000000000000, 2239.771999999999935 ) ) ;
#8044=TOROIDAL_SURFACE ( 'NONE', #20036, 4.114799999999999791, 1.270000000000000018 ) ;
#8046=CARTESIAN_POINT ( 'NONE',  ( 145.1961821871802272, -3661.071248187899528, 2244.703885868029829 ) ) ;
#8049=AXIS2_PLACEMENT_3D ( 'NONE', #3406, #10559, #11358 ) ;
#8050=CARTESIAN_POINT ( 'NONE',  ( 14.79088965948426804, -3661.435447629304235, 2249.925490890767378 ) ) ;
#8052=AXIS2_PLACEMENT_3D ( 'NONE', #22937, #7037, #19441 ) ;
#8055=ORIENTED_EDGE ( 'NONE', *, *, #18163, .F. ) ;
#8057=DIRECTION ( 'NONE',  ( -1.000000000000000000, 0.000000000000000000, 0.000000000000000000 ) ) ;
#8058=EDGE_CURVE ( 'NONE', #928, #21153, #10367, .T. ) ;
#8060=CARTESIAN_POINT ( 'NONE',  ( 15.48600340796466135, -3658.926920653574598, 2249.965218490672214 ) ) ;
#8062=VERTEX_POINT ( 'NONE', #4859 ) ;
#8068=CARTESIAN_POINT ( 'NONE',  ( 145.1457547493498055, -3581.228764793822393, 2245.816281768045428 ) ) ;
#8069=AXIS2_PLACEMENT_3D ( 'NONE', #4793, #8080, #11472 ) ;
#8071=TOROIDAL_SURFACE ( 'NONE', #4702, 3.606799999999999784, 0.7620000000000000107 ) ;
#8073=CARTESIAN_POINT ( 'NONE',  ( 17.77895441395078890, -3662.125108044190711, 2245.354081002604289 ) ) ;
#8075=FACE_OUTER_BOUND ( 'NONE', #6006, .T. ) ;
#8076=VECTOR ( 'NONE', #17251, 1000.000000000000000 ) ;
#8078=ORIENTED_EDGE ( 'NONE', *, *, #16885, .T. ) ;
#8080=DIRECTION ( 'NONE',  ( 0.000000000000000000, 1.000000000000000000, 0.000000000000000000 ) ) ;
#8082=CIRCLE ( 'NONE', #21915, 2.844800000000001550 ) ;
#8084=DIRECTION ( 'NONE',  ( 1.000000000000000000, 0.000000000000000000, 1.344534956950000190E-13 ) ) ;
#8087=VERTEX_POINT ( 'NONE', #1341 ) ;
#8088=AXIS2_PLACEMENT_3D ( 'NONE', #23049, #16260, #21656 ) ;
#8095=EDGE_CURVE ( 'NONE', #18734, #7197, #11695, .T. ) ;
#8096=ORIENTED_EDGE ( 'NONE', *, *, #1029, .F. ) ;
#8099=CARTESIAN_POINT ( 'NONE',  ( 10.97145801871307924, -3577.235475337109165, 2249.727398826565604 ) ) ;
#8101=CIRCLE ( 'NONE', #11093, 2.844800000000091700 ) ;
#8102=CIRCLE ( 'NONE', #16329, 2.844799999999994444 ) ;
#8104=VERTEX_POINT ( 'NONE', #20921 ) ;
#8109=PRODUCT_DEFINITION_SHAPE ( 'NONE', 'NONE',  #15652 ) ;
#8110=VECTOR ( 'NONE', #7203, 1000.000000000000000 ) ;
#8113=AXIS2_PLACEMENT_3D ( 'NONE', #14595, #18217, #638 ) ;
#8114=VECTOR ( 'NONE', #2855, 1000.000000000000000 ) ;
#8115=CARTESIAN_POINT ( 'NONE',  ( 142.2944679814244751, -3660.711379646646492, 2250.192293398927632 ) ) ;
#8116=ORIENTED_EDGE ( 'NONE', *, *, #13590, .F. ) ;
#8117=ORIENTED_EDGE ( 'NONE', *, *, #4263, .T. ) ;
#8118=CARTESIAN_POINT ( 'NONE',  ( 10.16000000000000014, -3544.570000000000164, 2255.774000000000342 ) ) ;
#8119=ORIENTED_EDGE ( 'NONE', *, *, #11851, .F. ) ;
#8120=DIRECTION ( 'NONE',  ( 1.000000000000000000, 0.000000000000000000, 1.165588477298000095E-13 ) ) ;
#8121=DIRECTION ( 'NONE',  ( -1.000000000000000000, 0.000000000000000000, 0.000000000000000000 ) ) ;
#8122=AXIS2_PLACEMENT_3D ( 'NONE', #9964, #22152, #7873 ) ;
#8123=EDGE_LOOP ( 'NONE', ( #20577, #23111 ) ) ;
#8125=AXIS2_PLACEMENT_3D ( 'NONE', #15155, #22282, #12217 ) ;
#8128=FACE_OUTER_BOUND ( 'NONE', #17910, .T. ) ;
#8130=ADVANCED_FACE ( 'NONE', ( #8505 ), #11822, .T. ) ;
#8131=EDGE_CURVE ( 'NONE', #19682, #4249, #14830, .T. ) ;
#8134=DIRECTION ( 'NONE',  ( -1.000000000000000000, 0.000000000000000000, 0.000000000000000000 ) ) ;
#8135=DIRECTION ( 'NONE',  ( 1.000000000000000000, 0.000000000000000000, 0.000000000000000000 ) ) ;
#8137=ORIENTED_EDGE ( 'NONE', *, *, #11146, .F. ) ;
#8139=CARTESIAN_POINT ( 'NONE',  ( 137.1349247998588794, -3544.173420539443214, 2255.711168198842643 ) ) ;
#8140=AXIS2_PLACEMENT_3D ( 'NONE', #9260, #119, #12651 ) ;
#8143=DIRECTION ( 'NONE',  ( 0.000000000000000000, 0.000000000000000000, 1.000000000000000000 ) ) ;
#8148=CARTESIAN_POINT ( 'NONE',  ( 63.50000000000000000, -3644.899999999999636, 2260.600000000000364 ) ) ;
#8153=CARTESIAN_POINT ( 'NONE',  ( 21.79320000000099711, -3568.700000000000273, 2259.837999999999738 ) ) ;
#8157=CIRCLE ( 'NONE', #2176, 1.269999999999882334 ) ;
#8160=CARTESIAN_POINT ( 'NONE',  ( 145.3865858764642383, -3658.926257878062643, 2244.815985133692266 ) ) ;
#8162=DIRECTION ( 'NONE',  ( 1.000000000000000000, 0.000000000000000000, 0.000000000000000000 ) ) ;
#8166=CARTESIAN_POINT ( 'NONE',  ( 145.3787012162004544, -3660.148468257834793, 2244.547209130087140 ) ) ;
#8169=EDGE_CURVE ( 'NONE', #3614, #10242, #19993, .T. ) ;
#8170=CARTESIAN_POINT ( 'NONE',  ( 14.73423477643819268, -3661.495730106304563, 2249.893851560407256 ) ) ;
#8174=CARTESIAN_POINT ( 'NONE',  ( 7.387125747139000609, -3581.600847139000052, 2246.630000000000109 ) ) ;
#8176=CARTESIAN_POINT ( 'NONE',  ( 142.7470794804999912, -3695.699999999999818, 2254.503999999999905 ) ) ;
#8185=CARTESIAN_POINT ( 'NONE',  ( 35.56000000000000227, -3543.299999999999727, 2247.392000000000280 ) ) ;
#8187=CARTESIAN_POINT ( 'NONE',  ( 17.58955766687454769, -3662.463685539857579, 2245.750755658854814 ) ) ;
#8188=CIRCLE ( 'NONE', #22762, 0.7619999999999294005 ) ;
#8189=CARTESIAN_POINT ( 'NONE',  ( 15.44319999999931525, -3660.383257047475126, 2255.967040000000907 ) ) ;
#8190=CARTESIAN_POINT ( 'NONE',  ( 124.1552000000010025, -3619.500000000000000, 2259.837999999999738 ) ) ;
#8191=B_SPLINE_CURVE_WITH_KNOTS ( 'NONE', 3,
 ( #14035, #21187, #10275, #15439 ),
 .UNSPECIFIED., .F., .F.,
 ( 4, 4 ),
 ( 0.000000000000000000, 1.000000000000000000 ),
 .UNSPECIFIED. ) ;
#8193=EDGE_LOOP ( 'NONE', ( #11048, #8096, #18351, #20030 ) ) ;
#8194=DIRECTION ( 'NONE',  ( -1.000000000000000000, 0.000000000000000000, 0.000000000000000000 ) ) ;
#8196=ORIENTED_EDGE ( 'NONE', *, *, #516, .T. ) ;
#8198=CARTESIAN_POINT ( 'NONE',  ( 10.63228947054044760, -3657.550950343449131, 2248.571178883313223 ) ) ;
#8199=VERTEX_POINT ( 'NONE', #13055 ) ;
#8201=VERTEX_POINT ( 'NONE', #14587 ) ;
#8203=AXIS2_PLACEMENT_3D ( 'NONE', #4503, #10365, #11642 ) ;
#8206=FACE_OUTER_BOUND ( 'NONE', #18450, .T. ) ;
#8208=CARTESIAN_POINT ( 'NONE',  ( 142.2925313698394234, -3580.666266504254054, 2249.589929609103820 ) ) ;
#8215=AXIS2_PLACEMENT_3D ( 'NONE', #21285, #19403, #4991 ) ;
#8216=CARTESIAN_POINT ( 'NONE',  ( 134.2764082060851933, -3657.703343431524900, 2245.923799496059928 ) ) ;
#8217=ADVANCED_FACE ( 'NONE', ( #7439 ), #8764, .T. ) ;
#8219=ORIENTED_EDGE ( 'NONE', *, *, #829, .T. ) ;
#8220=CARTESIAN_POINT ( 'NONE',  ( 142.1265142685761873, -3660.990011674679408, 2250.106896142239293 ) ) ;
#8225=ORIENTED_EDGE ( 'NONE', *, *, #501, .T. ) ;
#8230=AXIS2_PLACEMENT_3D ( 'NONE', #14193, #1760, #7155 ) ;
#8233=DIRECTION ( 'NONE',  ( -1.000000000000000000, 0.000000000000000000, 0.000000000000000000 ) ) ;
#8236=LINE ( 'NONE', #9532, #11471 ) ;
#8239=CARTESIAN_POINT ( 'NONE',  ( 1.270000000000000018, -3695.699999999999818, 2259.329999999999927 ) ) ;
#8241=DIRECTION ( 'NONE',  ( 0.000000000000000000, 0.000000000000000000, 1.000000000000000000 ) ) ;
#8242=CARTESIAN_POINT ( 'NONE',  ( 141.8175935050403780, -3657.605346374574765, 2248.683677737056314 ) ) ;
#8243=FACE_OUTER_BOUND ( 'NONE', #10536, .T. ) ;
#8247=ADVANCED_FACE ( 'NONE', ( #14703 ), #9983, .T. ) ;
#8250=ORIENTED_EDGE ( 'NONE', *, *, #9513, .F. ) ;
#8251=DIRECTION ( 'NONE',  ( 0.000000000000000000, 0.000000000000000000, -1.000000000000000000 ) ) ;
#8252=ADVANCED_FACE ( 'NONE', ( #16564 ), #20833, .T. ) ;
#8253=EDGE_CURVE ( 'NONE', #6304, #18734, #10720, .T. ) ;
#8255=EDGE_LOOP ( 'NONE', ( #14736, #21117, #2275, #15215 ) ) ;
#8257=DIRECTION ( 'NONE',  ( 0.000000000000000000, 0.000000000000000000, -1.000000000000000000 ) ) ;
#8259=DIRECTION ( 'NONE',  ( -1.000000000000000000, 0.000000000000000000, 0.000000000000000000 ) ) ;
#8261=DIRECTION ( 'NONE',  ( 1.000000000000000000, 0.000000000000000000, 0.000000000000000000 ) ) ;
#8264=CARTESIAN_POINT ( 'NONE',  ( 18.13822863179804301, -3577.698793233671040, 2244.777281343887807 ) ) ;
#8265=CARTESIAN_POINT ( 'NONE',  ( 0.000000000000000000, -3544.570000000000164, 2259.329999999999927 ) ) ;
#8269=CARTESIAN_POINT ( 'NONE',  ( 47.19319999999999737, -3619.500000000000000, 2239.009999999999764 ) ) ;
#8272=CARTESIAN_POINT ( 'NONE',  ( 10.41817338763723022, -3581.193830325411454, 2249.018787504950069 ) ) ;
#8277=CARTESIAN_POINT ( 'NONE',  ( 144.8225857063939372, -3662.039185438572531, 2245.272442455612236 ) ) ;
#8278=CARTESIAN_POINT ( 'NONE',  ( 15.44319999999931525, -3578.616742952524419, 2255.967040000000907 ) ) ;
#8284=ADVANCED_FACE ( 'NONE', ( #5575 ), #19861, .F. ) ;
#8286=DIRECTION ( 'NONE',  ( 0.000000000000000000, -1.000000000000000000, 0.000000000000000000 ) ) ;
#8289=DIRECTION ( 'NONE',  ( -0.000000000000000000, -1.000000000000000000, -0.000000000000000000 ) ) ;
#8290=CARTESIAN_POINT ( 'NONE',  ( 20.62424768829000143, -3694.430000000000291, 2260.600000000000364 ) ) ;
#8292=ADVANCED_FACE ( 'NONE', ( #8128 ), #9868, .F. ) ;
#8294=EDGE_LOOP ( 'NONE', ( #802, #11257, #21638, #7595 ) ) ;
#8298=B_SPLINE_CURVE_WITH_KNOTS ( 'NONE', 3,
 ( #11643, #16922, #18579, #15412 ),
 .UNSPECIFIED., .F., .F.,
 ( 4, 4 ),
 ( 0.000000000000000000, 1.000000000000000000 ),
 .UNSPECIFIED. ) ;
#8299=CARTESIAN_POINT ( 'NONE',  ( 9.787381488757823433, -3543.344914975609754, 2254.841485305899823 ) ) ;
#8301=EDGE_CURVE ( 'NONE', #8104, #3611, #22695, .T. ) ;
#8302=CYLINDRICAL_SURFACE ( 'NONE', #2696, 2.844799999999009010 ) ;
#8304=CYLINDRICAL_SURFACE ( 'NONE', #16834, 2.844800000000091700 ) ;
#8306=CARTESIAN_POINT ( 'NONE',  ( 15.54479999999932716, -3659.956214629474744, 2256.063560000000962 ) ) ;
#8307=DIRECTION ( 'NONE',  ( 1.000000000000000000, 0.000000000000000000, 0.000000000000000000 ) ) ;
#8311=CARTESIAN_POINT ( 'NONE',  ( 101.5999999999999943, -3568.700000000000273, 2260.600000000000364 ) ) ;
#8313=LINE ( 'NONE', #8432, #13297 ) ;
#8314=ORIENTED_EDGE ( 'NONE', *, *, #12013, .F. ) ;
#8316=CARTESIAN_POINT ( 'NONE',  ( 139.6999999999999886, -3579.494999999999891, 2255.774000000000342 ) ) ;
#8317=ORIENTED_EDGE ( 'NONE', *, *, #21324, .T. ) ;
#8318=EDGE_LOOP ( 'NONE', ( #8799, #6548, #20434, #8603 ) ) ;
#8319=CARTESIAN_POINT ( 'NONE',  ( 134.0487369367239694, -3580.386377785477634, 2244.978268890278741 ) ) ;
#8321=AXIS2_PLACEMENT_3D ( 'NONE', #13082, #11775, #998 ) ;
#8324=DIRECTION ( 'NONE',  ( 1.000000000000000000, 0.000000000000000000, 0.000000000000000000 ) ) ;
#8326=CARTESIAN_POINT ( 'NONE',  ( 136.9738742589587162, -3580.309117874636740, 2249.840541574770668 ) ) ;
#8328=ORIENTED_EDGE ( 'NONE', *, *, #8941, .F. ) ;
#8330=CARTESIAN_POINT ( 'NONE',  ( 131.9330360192018077, -3695.324988468914853, 2260.231623935620519 ) ) ;
#8334=CARTESIAN_POINT ( 'NONE',  ( 14.56265065754690191, -3581.645345613470909, 2247.977218229329537 ) ) ;
#8335=CARTESIAN_POINT ( 'NONE',  ( 134.2762276231818532, -3657.703887669735650, 2245.922900958339142 ) ) ;
#8336=VECTOR ( 'NONE', #11538, 1000.000000000000000 ) ;
#8337=VERTEX_POINT ( 'NONE', #7783 ) ;
#8340=CARTESIAN_POINT ( 'NONE',  ( 85.29320000000001301, -3594.099999999999909, 2259.837999999999738 ) ) ;
#8341=ORIENTED_EDGE ( 'NONE', *, *, #5407, .F. ) ;
#8342=DIRECTION ( 'NONE',  ( 0.000000000000000000, 0.000000000000000000, -1.000000000000000000 ) ) ;
#8343=AXIS2_PLACEMENT_3D ( 'NONE', #11895, #6055, #869 ) ;
#8346=FACE_OUTER_BOUND ( 'NONE', #4014, .T. ) ;
#8349=LINE ( 'NONE', #8694, #786 ) ;
#8351=ORIENTED_EDGE ( 'NONE', *, *, #1108, .F. ) ;
#8354=EDGE_CURVE ( 'NONE', #4174, #2146, #8236, .T. ) ;
#8355=FACE_OUTER_BOUND ( 'NONE', #8645, .T. ) ;
#8357=LINE ( 'NONE', #4827, #14870 ) ;
#8358=AXIS2_PLACEMENT_3D ( 'NONE', #16175, #3288, #9147 ) ;
#8361=LINE ( 'NONE', #15499, #21571 ) ;
#8363=CARTESIAN_POINT ( 'NONE',  ( 127.0000000000000000, -3619.500000000000000, 2260.600000000000364 ) ) ;
#8365=CARTESIAN_POINT ( 'NONE',  ( 141.6571813405579405, -3657.440126662888360, 2248.289601892444352 ) ) ;
#8366=ADVANCED_FACE ( 'NONE', ( #11619 ), #13350, .T. ) ;
#8370=CARTESIAN_POINT ( 'NONE',  ( 12.69999999999999929, -3579.494999999999891, 2246.630000000000109 ) ) ;
#8371=FACE_OUTER_BOUND ( 'NONE', #7314, .T. ) ;
#8373=ORIENTED_EDGE ( 'NONE', *, *, #22559, .F. ) ;
#8374=CARTESIAN_POINT ( 'NONE',  ( 142.4431999999993366, -3660.383257047431925, 2255.967040000000907 ) ) ;
#8375=DIRECTION ( 'NONE',  ( -1.000000000000000000, 0.000000000000000000, 0.000000000000000000 ) ) ;
#8376=DIRECTION ( 'NONE',  ( 0.000000000000000000, -1.000000000000000000, 0.000000000000000000 ) ) ;
#8380=CARTESIAN_POINT ( 'NONE',  ( 116.8400000000000034, -3694.430000000000291, 2247.392000000000280 ) ) ;
#8381=DIRECTION ( 'NONE',  ( -1.000000000000000000, 0.000000000000000000, 0.000000000000000000 ) ) ;
#8384=EDGE_CURVE ( 'NONE', #20696, #444, #3249, .T. ) ;
#8388=ORIENTED_EDGE ( 'NONE', *, *, #3771, .T. ) ;
#8391=DIRECTION ( 'NONE',  ( 0.000000000000000000, 0.000000000000000000, 1.000000000000000000 ) ) ;
#8395=CARTESIAN_POINT ( 'NONE',  ( 25.39999999999999858, -3619.500000000000000, 2261.869999999999891 ) ) ;
#8396=ADVANCED_FACE ( 'NONE', ( #15382 ), #7374, .T. ) ;
#8398=CARTESIAN_POINT ( 'NONE',  ( 144.7204148360012255, -3662.235733769309263, 2245.468189506944327 ) ) ;
#8403=DIRECTION ( 'NONE',  ( 0.000000000000000000, 0.000000000000000000, -1.000000000000000000 ) ) ;
#8404=AXIS2_PLACEMENT_3D ( 'NONE', #22680, #2062, #16352 ) ;
#8405=CARTESIAN_POINT ( 'NONE',  ( 34.49320000000000164, -3594.099999999999909, 2239.009999999999764 ) ) ;
#8406=CIRCLE ( 'NONE', #3160, 0.7619999999999987894 ) ;
#8407=FACE_OUTER_BOUND ( 'NONE', #18391, .T. ) ;
#8411=ORIENTED_EDGE ( 'NONE', *, *, #2100, .F. ) ;
#8414=CARTESIAN_POINT ( 'NONE',  ( 9.971028676360534249, -3543.580319128281644, 2255.300887233377580 ) ) ;
#8419=CARTESIAN_POINT ( 'NONE',  ( 60.65520000000000067, -3644.899999999999636, 2239.771999999999935 ) ) ;
#8420=CARTESIAN_POINT ( 'NONE',  ( 9.855199999999999960, -3659.504999999999654, 2272.030000000000200 ) ) ;
#8422=B_SPLINE_CURVE_WITH_KNOTS ( 'NONE', 3,
 ( #9376, #466, #11242, #16748 ),
 .UNSPECIFIED., .F., .F.,
 ( 4, 4 ),
 ( 0.000000000000000000, 1.000000000000000000 ),
 .UNSPECIFIED. ) ;
#8423=AXIS2_PLACEMENT_3D ( 'NONE', #10789, #8686, #5054 ) ;
#8424=DIRECTION ( 'NONE',  ( 0.000000000000000000, -1.000000000000000000, 0.000000000000000000 ) ) ;
#8426=DIRECTION ( 'NONE',  ( -1.000000000000000000, 0.000000000000000000, 0.000000000000000000 ) ) ;
#8428=DIRECTION ( 'NONE',  ( -0.000000000000000000, -1.000000000000000000, -0.000000000000000000 ) ) ;
#8429=EDGE_CURVE ( 'NONE', #2255, #8201, #272, .T. ) ;
#8432=CARTESIAN_POINT ( 'NONE',  ( 127.0000000000000000, -3660.140000000000327, 2250.236800000000130 ) ) ;
#8434=CARTESIAN_POINT ( 'NONE',  ( 25.39999999999999858, -3670.300000000000182, 2261.869999999999891 ) ) ;
#8436=B_SPLINE_CURVE_WITH_KNOTS ( 'NONE', 3,
 ( #8787, #10424, #5273, #19223 ),
 .UNSPECIFIED., .F., .F.,
 ( 4, 4 ),
 ( 0.000000000000000000, 1.000000000000000000 ),
 .UNSPECIFIED. ) ;
#8439=EDGE_CURVE ( 'NONE', #17151, #10571, #999, .T. ) ;
#8447=DIRECTION ( 'NONE',  ( 0.000000000000000000, 0.000000000000000000, -1.000000000000000000 ) ) ;
#8451=ORIENTED_EDGE ( 'NONE', *, *, #18440, .F. ) ;
#8452=CARTESIAN_POINT ( 'NONE',  ( 131.7911717319573484, -3695.576947737646606, 2259.876481750800394 ) ) ;
#8454=EDGE_CURVE ( 'NONE', #14892, #3037, #13977, .T. ) ;
#8456=CARTESIAN_POINT ( 'NONE',  ( 114.2999999999999972, -3644.899999999999636, 2259.837999999999738 ) ) ;
#8457=CARTESIAN_POINT ( 'NONE',  ( 134.0212837167035502, -3658.862064473952614, 2244.850302162179105 ) ) ;
#8465=CYLINDRICAL_SURFACE ( 'NONE', #7250, 2.844800000000001550 ) ;
#8466=CIRCLE ( 'NONE', #8851, 0.7619999999999987894 ) ;
#8467=ORIENTED_EDGE ( 'NONE', *, *, #20404, .T. ) ;
#8468=AXIS2_PLACEMENT_3D ( 'NONE', #1192, #13506, #4600 ) ;
#8471=ORIENTED_EDGE ( 'NONE', *, *, #14607, .F. ) ;
#8473=FACE_OUTER_BOUND ( 'NONE', #153, .T. ) ;
#8474=DIRECTION ( 'NONE',  ( 0.000000000000000000, 0.000000000000000000, -1.000000000000000000 ) ) ;
#8481=CARTESIAN_POINT ( 'NONE',  ( 88.90000000000000568, -3644.899999999999636, 2259.837999999999738 ) ) ;
#8483=CARTESIAN_POINT ( 'NONE',  ( 18.41499991942999159, -3579.609095813635122, 2244.645121672054302 ) ) ;
#8485=CIRCLE ( 'NONE', #3236, 0.7619999999999987894 ) ;
#8486=CARTESIAN_POINT ( 'NONE',  ( 142.0943346817877284, -3657.968795034299546, 2249.230143411615245 ) ) ;
#8490=ORIENTED_EDGE ( 'NONE', *, *, #15719, .T. ) ;
#8492=DIRECTION ( 'NONE',  ( 1.000000000000000000, 0.000000000000000000, 0.000000000000000000 ) ) ;
#8493=EDGE_LOOP ( 'NONE', ( #17581, #18803, #5695, #20834 ) ) ;
#8495=CARTESIAN_POINT ( 'NONE',  ( 4.806249414519654373, -3543.438632180929289, 2259.914298575651628 ) ) ;
#8496=CARTESIAN_POINT ( 'NONE',  ( 151.4000000000000057, -3695.670967364599164, 2240.279999999999745 ) ) ;
#8497=CIRCLE ( 'NONE', #21602, 2.844799999999994444 ) ;
#8498=CARTESIAN_POINT ( 'NONE',  ( 137.1599999999999966, -3660.786127253999894, 2255.774000000000342 ) ) ;
#8505=FACE_OUTER_BOUND ( 'NONE', #5759, .T. ) ;
#8506=ORIENTED_EDGE ( 'NONE', *, *, #17722, .F. ) ;
#8515=FACE_BOUND ( 'NONE', #11247, .T. ) ;
#8518=ADVANCED_FACE ( 'NONE', ( #21129 ), #14113, .T. ) ;
#8519=VECTOR ( 'NONE', #5039, 1000.000000000000000 ) ;
#8521=CARTESIAN_POINT ( 'NONE',  ( 144.6523069729103099, -3662.357674682753895, 2245.609748382597900 ) ) ;
#8523=CARTESIAN_POINT ( 'NONE',  ( 11.52540003424859982, -3662.096080434181204, 2249.457718961763021 ) ) ;
#8525=CARTESIAN_POINT ( 'NONE',  ( 147.3199999999999932, -3544.570000000000164, 2260.600000000000364 ) ) ;
#8526=ORIENTED_EDGE ( 'NONE', *, *, #19094, .T. ) ;
#8530=DIRECTION ( 'NONE',  ( 0.000000000000000000, 0.000000000000000000, 1.000000000000000000 ) ) ;
#8531=CARTESIAN_POINT ( 'NONE',  ( 15.09459832061900464, -3657.969225429738799, 2249.230664226648514 ) ) ;
#8532=DIRECTION ( 'NONE',  ( 0.000000000000000000, 0.000000000000000000, 1.000000000000000000 ) ) ;
#8534=ADVANCED_FACE ( 'NONE', ( #5071 ), #22753, .F. ) ;
#8538=EDGE_CURVE ( 'NONE', #17318, #22471, #22399, .T. ) ;
#8542=FACE_OUTER_BOUND ( 'NONE', #19845, .T. ) ;
#8545=CARTESIAN_POINT ( 'NONE',  ( 1.270000000000000018, -3660.140000000000327, 2243.277199999999993 ) ) ;
#8550=CYLINDRICAL_SURFACE ( 'NONE', #20795, 2.844800000000001550 ) ;
#8554=CARTESIAN_POINT ( 'NONE',  ( 136.8551930557000276, -3659.505009668000184, 2250.165028799000083 ) ) ;
#8555=CARTESIAN_POINT ( 'NONE',  ( 10.68379541473369976, -3657.497568268327541, 2248.446992609373410 ) ) ;
#8556=EDGE_CURVE ( 'NONE', #16324, #2966, #2882, .T. ) ;
#8558=EDGE_LOOP ( 'NONE', ( #8598, #8137, #15346, #13736 ) ) ;
#8559=CARTESIAN_POINT ( 'NONE',  ( 134.3605230499748302, -3581.533682376092202, 2246.411846944817171 ) ) ;
#8561=CARTESIAN_POINT ( 'NONE',  ( 15.24000000000000021, -3580.776127254000130, 2255.774000000000342 ) ) ;
#8564=ORIENTED_EDGE ( 'NONE', *, *, #14591, .T. ) ;
#8565=AXIS2_PLACEMENT_3D ( 'NONE', #10886, #1751, #8901 ) ;
#8568=CARTESIAN_POINT ( 'NONE',  ( 6.222999999999998977, -3659.504999999999654, 2239.771999999999935 ) ) ;
#8569=CARTESIAN_POINT ( 'NONE',  ( 15.39964945764670645, -3580.393900429462519, 2249.788766634620060 ) ) ;
#8571=CARTESIAN_POINT ( 'NONE',  ( 133.9850000806000025, -3659.504501929000071, 2244.618659328000376 ) ) ;
#8573=VERTEX_POINT ( 'NONE', #7070 ) ;
#8576=AXIS2_PLACEMENT_3D ( 'NONE', #20225, #3939, #11094 ) ;
#8578=EDGE_CURVE ( 'NONE', #20939, #17497, #8357, .T. ) ;
#8580=ORIENTED_EDGE ( 'NONE', *, *, #22888, .F. ) ;
#8582=CARTESIAN_POINT ( 'NONE',  ( 57.14999999999999858, -3670.300000000000182, 2247.392000000000280 ) ) ;
#8586=CARTESIAN_POINT ( 'NONE',  ( 127.0000000000000000, -3660.140000000000327, 2247.392000000000280 ) ) ;
#8590=CARTESIAN_POINT ( 'NONE',  ( 1.270000000000000018, -3660.140000000000327, 2251.506800000000112 ) ) ;
#8591=CARTESIAN_POINT ( 'NONE',  ( 18.38859181429490519, -3580.043763408477844, 2244.804994013233681 ) ) ;
#8592=AXIS2_PLACEMENT_3D ( 'NONE', #15876, #5219, #10944 ) ;
#8593=EDGE_CURVE ( 'NONE', #10141, #22306, #11981, .T. ) ;
#8594=EDGE_CURVE ( 'NONE', #15748, #13823, #17840, .T. ) ;
#8595=CARTESIAN_POINT ( 'NONE',  ( 141.5264891900619659, -3657.323731859511554, 2246.960912804729105 ) ) ;
#8596=ORIENTED_EDGE ( 'NONE', *, *, #17718, .T. ) ;
#8597=DIRECTION ( 'NONE',  ( 0.000000000000000000, 0.000000000000000000, -1.000000000000000000 ) ) ;
#8598=ORIENTED_EDGE ( 'NONE', *, *, #16012, .F. ) ;
#8599=VERTEX_POINT ( 'NONE', #1432 ) ;
#8600=ORIENTED_EDGE ( 'NONE', *, *, #12089, .T. ) ;
#8602=ORIENTED_EDGE ( 'NONE', *, *, #16811, .F. ) ;
#8603=ORIENTED_EDGE ( 'NONE', *, *, #17722, .T. ) ;
#8608=CARTESIAN_POINT ( 'NONE',  ( 127.0000000000000000, -3660.140000000000327, 2250.236800000000130 ) ) ;
#8610=CARTESIAN_POINT ( 'NONE',  ( 18.37960467573999779, -3578.859731361000286, 2244.547525601999951 ) ) ;
#8612=CARTESIAN_POINT ( 'NONE',  ( 137.1599999999999966, -3578.213872745999652, 2255.774000000000342 ) ) ;
#8613=CARTESIAN_POINT ( 'NONE',  ( 59.89320000000000022, -3644.899999999999636, 2260.600000000000364 ) ) ;
#8614=DIRECTION ( 'NONE',  ( 0.000000000000000000, 0.000000000000000000, -1.000000000000000000 ) ) ;
#8616=DIRECTION ( 'NONE',  ( 1.000000000000000000, 0.000000000000000000, 0.000000000000000000 ) ) ;
#8621=CARTESIAN_POINT ( 'NONE',  ( 10.06389858027753448, -3580.564515547758219, 2249.669647745964994 ) ) ;
#8622=DIRECTION ( 'NONE',  ( 1.000000000000000000, 0.000000000000000000, 0.000000000000000000 ) ) ;
#8625=ORIENTED_EDGE ( 'NONE', *, *, #7556, .T. ) ;
#8629=CARTESIAN_POINT ( 'NONE',  ( 131.9679793872000175, -3694.678775005999796, 2260.577432963000319 ) ) ;
#8630=CARTESIAN_POINT ( 'NONE',  ( 9.990450446634426385, -3660.417187683251086, 2250.236801297000056 ) ) ;
#8632=ORIENTED_EDGE ( 'NONE', *, *, #4435, .T. ) ;
#8633=DIRECTION ( 'NONE',  ( 0.000000000000000000, 0.000000000000000000, -1.000000000000000000 ) ) ;
#8636=CARTESIAN_POINT ( 'NONE',  ( 116.8400000000000034, -3694.430000000000291, 2247.392000000000280 ) ) ;
#8637=DIRECTION ( 'NONE',  ( 0.000000000000000000, 0.000000000000000000, -1.000000000000000000 ) ) ;
#8644=EDGE_CURVE ( 'NONE', #16167, #7890, #12564, .T. ) ;
#8645=EDGE_LOOP ( 'NONE', ( #13357, #20838, #4383, #10589 ) ) ;
#8651=FACE_OUTER_BOUND ( 'NONE', #13615, .T. ) ;
#8653=DIRECTION ( 'NONE',  ( 0.000000000000000000, 0.000000000000000000, -1.000000000000000000 ) ) ;
#8654=CARTESIAN_POINT ( 'NONE',  ( 17.33724445481948706, -3576.154475310671842, 2246.502948247453787 ) ) ;
#8659=DIRECTION ( 'NONE',  ( 0.000000000000000000, 0.000000000000000000, 1.000000000000000000 ) ) ;
#8660=DIRECTION ( 'NONE',  ( 0.000000000000000000, 0.000000000000000000, -1.000000000000000000 ) ) ;
#8662=EDGE_CURVE ( 'NONE', #16167, #7575, #10000, .T. ) ;
#8663=LINE ( 'NONE', #5157, #3174 ) ;
#8664=DIRECTION ( 'NONE',  ( -0.8928571428563309986, 0.4503400076058416968, 0.000000000000000000 ) ) ;
#8667=DIRECTION ( 'NONE',  ( 1.000000000000000000, 0.000000000000000000, 0.000000000000000000 ) ) ;
#8670=DIRECTION ( 'NONE',  ( -1.000000000000000000, 0.000000000000000000, 0.000000000000000000 ) ) ;
#8673=EDGE_CURVE ( 'NONE', #9684, #12626, #15251, .T. ) ;
#8678=EDGE_CURVE ( 'NONE', #6472, #19890, #1012, .T. ) ;
#8679=CARTESIAN_POINT ( 'NONE',  ( 15.37455142657321083, -3580.464775575591375, 2249.741195994737609 ) ) ;
#8685=CARTESIAN_POINT ( 'NONE',  ( 15.39361733587799819, -3695.340677397469335, 2255.389245125670186 ) ) ;
#8686=DIRECTION ( 'NONE',  ( 0.000000000000000000, 0.000000000000000000, 1.000000000000000000 ) ) ;
#8687=ORIENTED_EDGE ( 'NONE', *, *, #7280, .T. ) ;
#8688=EDGE_CURVE ( 'NONE', #1252, #14593, #7295, .T. ) ;
#8689=CARTESIAN_POINT ( 'NONE',  ( 101.5999999999999943, -3568.700000000000273, 2260.600000000000364 ) ) ;
#8692=ORIENTED_EDGE ( 'NONE', *, *, #21603, .F. ) ;
#8693=ORIENTED_EDGE ( 'NONE', *, *, #21895, .F. ) ;
#8694=CARTESIAN_POINT ( 'NONE',  ( 98.75520000000000209, -3670.300000000000182, 2261.869999999999891 ) ) ;
#8697=AXIS2_PLACEMENT_3D ( 'NONE', #2783, #16426, #9928 ) ;
#8698=ORIENTED_EDGE ( 'NONE', *, *, #10304, .T. ) ;
#8699=AXIS2_PLACEMENT_3D ( 'NONE', #20702, #8532, #1015 ) ;
#8703=DIRECTION ( 'NONE',  ( 1.000000000000000000, 0.000000000000000000, 0.000000000000000000 ) ) ;
#8706=CARTESIAN_POINT ( 'NONE',  ( 9.886249413367808714, -3695.561367819954285, 2255.088298574058626 ) ) ;
#8707=CARTESIAN_POINT ( 'NONE',  ( 18.31792581816387155, -3580.544012085188569, 2245.098288300677268 ) ) ;
#8708=CIRCLE ( 'NONE', #3833, 1.240967364599221412 ) ;
#8709=ADVANCED_FACE ( 'NONE', ( #10803 ), #17944, .F. ) ;
#8710=CARTESIAN_POINT ( 'NONE',  ( 142.1023807964371883, -3657.981398713484396, 2249.244952485364138 ) ) ;
#8713=VERTEX_POINT ( 'NONE', #16422 ) ;
#8714=VECTOR ( 'NONE', #9777, 1000.000000000000000 ) ;
#8720=ORIENTED_EDGE ( 'NONE', *, *, #3938, .F. ) ;
#8725=CARTESIAN_POINT ( 'NONE',  ( 4.931826670915151034, -3543.672816123386383, 2260.228926848877109 ) ) ;
#8728=CIRCLE ( 'NONE', #17696, 2.844799999998995244 ) ;
#8729=DIRECTION ( 'NONE',  ( -1.000000000000000000, 0.000000000000000000, 0.000000000000000000 ) ) ;
#8733=EDGE_CURVE ( 'NONE', #4102, #3518, #20850, .T. ) ;
#8737=ORIENTED_EDGE ( 'NONE', *, *, #2841, .F. ) ;
#8740=CARTESIAN_POINT ( 'NONE',  ( 131.8995956651736208, -3543.598402616399198, 2260.148194448883260 ) ) ;
#8741=CARTESIAN_POINT ( 'NONE',  ( 10.31198979717081343, -3581.040930137735813, 2249.218597259193757 ) ) ;
#8742=EDGE_CURVE ( 'NONE', #15879, #4712, #22337, .T. ) ;
#8743=DIRECTION ( 'NONE',  ( 0.000000000000000000, 0.000000000000000000, 1.000000000000000000 ) ) ;
#8744=EDGE_LOOP ( 'NONE', ( #5066, #12430, #5846, #5742 ) ) ;
#8749=FACE_BOUND ( 'NONE', #14273, .T. ) ;
#8750=CARTESIAN_POINT ( 'NONE',  ( 1.270000000000000018, -3543.299999999999727, 2240.279999999999745 ) ) ;
#8751=CARTESIAN_POINT ( 'NONE',  ( 12.06527293566236203, -3662.278322999314241, 2249.268379514652679 ) ) ;
#8752=VECTOR ( 'NONE', #21347, 1000.000000000000000 ) ;
#8753=CARTESIAN_POINT ( 'NONE',  ( 10.16000000000000014, -3658.223872745999870, 2255.774000000000342 ) ) ;
#8758=CARTESIAN_POINT ( 'NONE',  ( 91.74479999999999791, -3644.899999999999636, 2261.869999999999891 ) ) ;
#8759=CARTESIAN_POINT ( 'NONE',  ( 14.50925869426821713, -3657.309602984159483, 2247.678649714388030 ) ) ;
#8760=CARTESIAN_POINT ( 'NONE',  ( 137.1599999999999397, -3694.509865589630408, 2255.773999999999432 ) ) ;
#8761=AXIS2_PLACEMENT_3D ( 'NONE', #19667, #12518, #21774 ) ;
#8764=TOROIDAL_SURFACE ( 'NONE', #13023, 4.114799999999999791, 1.270000000000000018 ) ;
#8767=CARTESIAN_POINT ( 'NONE',  ( 127.0000000000000000, -3568.700000000000273, 2261.869999999999891 ) ) ;
#8772=CARTESIAN_POINT ( 'NONE',  ( 17.53979493689646674, -3576.455561739696350, 2245.871465501990315 ) ) ;
#8773=DIRECTION ( 'NONE',  ( 0.000000000000000000, 0.000000000000000000, -1.000000000000000000 ) ) ;
#8778=TOROIDAL_SURFACE ( 'NONE', #5031, 3.606799999998999695, 0.7620000000000000107 ) ;
#8779=ORIENTED_EDGE ( 'NONE', *, *, #4777, .T. ) ;
#8780=CARTESIAN_POINT ( 'NONE',  ( 38.10000000000000142, -3594.099999999999909, 2239.009999999999764 ) ) ;
#8783=CARTESIAN_POINT ( 'NONE',  ( 19.17699999999999960, -3579.494999999999891, 2239.771999999999935 ) ) ;
#8785=ORIENTED_EDGE ( 'NONE', *, *, #3399, .F. ) ;
#8787=CARTESIAN_POINT ( 'NONE',  ( 15.54479999999999862, -3579.494999999999891, 2256.063560000000052 ) ) ;
#8790=VECTOR ( 'NONE', #20994, 1000.000000000000000 ) ;
#8792=CIRCLE ( 'NONE', #6171, 3.606799999999001027 ) ;
#8794=CARTESIAN_POINT ( 'NONE',  ( 15.52686321059681518, -3579.859966820806676, 2250.062296236718339 ) ) ;
#8795=CYLINDRICAL_SURFACE ( 'NONE', #17879, 2.844799999999994444 ) ;
#8798=DIRECTION ( 'NONE',  ( 1.000000000000000000, 0.000000000000000000, 0.000000000000000000 ) ) ;
#8799=ORIENTED_EDGE ( 'NONE', *, *, #4555, .F. ) ;
#8801=EDGE_CURVE ( 'NONE', #13188, #16556, #5528, .T. ) ;
#8803=EDGE_LOOP ( 'NONE', ( #13339, #20852 ) ) ;
#8804=TOROIDAL_SURFACE ( 'NONE', #1691, 3.606799999999999784, 0.7620000000000000107 ) ;
#8805=CARTESIAN_POINT ( 'NONE',  ( 5.080000000000000071, -3694.430000000000291, 2260.600000000000364 ) ) ;
#8807=VECTOR ( 'NONE', #6564, 1000.000000000000000 ) ;
#8808=EDGE_CURVE ( 'NONE', #12928, #17318, #20291, .T. ) ;
#8809=VECTOR ( 'NONE', #8084, 1000.000000000000000 ) ;
#8811=CARTESIAN_POINT ( 'NONE',  ( 15.24000000000000021, -3695.699999999999818, 2255.774000000000342 ) ) ;
#8815=CARTESIAN_POINT ( 'NONE',  ( 95.25000000000000000, -3670.300000000000182, 2244.547199999999975 ) ) ;
#8816=ORIENTED_EDGE ( 'NONE', *, *, #19476, .F. ) ;
#8817=DIRECTION ( 'NONE',  ( 0.000000000000000000, 0.000000000000000000, 1.000000000000000000 ) ) ;
#8818=CARTESIAN_POINT ( 'NONE',  ( 9.285288183368999526, -3544.570000000000164, 2254.853250718999789 ) ) ;
#8823=DIRECTION ( 'NONE',  ( 0.000000000000000000, 0.000000000000000000, -1.000000000000000000 ) ) ;
#8824=EDGE_CURVE ( 'NONE', #16556, #11901, #13477, .T. ) ;
#8825=AXIS2_PLACEMENT_3D ( 'NONE', #3122, #15903, #22795 ) ;
#8826=AXIS2_PLACEMENT_3D ( 'NONE', #9217, #9098, #12618 ) ;
#8827=CARTESIAN_POINT ( 'NONE',  ( 137.0863986929037708, -3658.381654322079612, 2249.628458754722033 ) ) ;
#8829=CARTESIAN_POINT ( 'NONE',  ( 137.0887894918462280, -3660.636540989195510, 2250.194016773457861 ) ) ;
#8832=EDGE_LOOP ( 'NONE', ( #8870, #9969, #1215 ) ) ;
#8833=ADVANCED_FACE ( 'NONE', ( #17108 ), #5896, .F. ) ;
#8835=ORIENTED_EDGE ( 'NONE', *, *, #1353, .F. ) ;
#8836=EDGE_LOOP ( 'NONE', ( #17558, #21613, #9241, #2715, #21486, #1305, #4589, #102 ) ) ;
#8840=DIRECTION ( 'NONE',  ( 1.000000000000000000, 0.000000000000000000, 0.000000000000000000 ) ) ;
#8843=EDGE_CURVE ( 'NONE', #6254, #9478, #9267, .T. ) ;
#8844=ORIENTED_EDGE ( 'NONE', *, *, #16996, .T. ) ;
#8847=DIRECTION ( 'NONE',  ( -1.000000000000000000, 0.000000000000000000, 0.000000000000000000 ) ) ;
#8849=FACE_OUTER_BOUND ( 'NONE', #1642, .T. ) ;
#8851=AXIS2_PLACEMENT_3D ( 'NONE', #6650, #20930, #4634 ) ;
#8852=ORIENTED_EDGE ( 'NONE', *, *, #4131, .T. ) ;
#8859=CARTESIAN_POINT ( 'NONE',  ( 50.79999999999999716, -3670.300000000000182, 2239.771999999999935 ) ) ;
#8860=VERTEX_POINT ( 'NONE', #20510 ) ;
#8862=CARTESIAN_POINT ( 'NONE',  ( 76.20000000000000284, -3568.700000000000273, 2259.837999999999738 ) ) ;
#8863=CIRCLE ( 'NONE', #21949, 3.606799999999993567 ) ;
#8865=CARTESIAN_POINT ( 'NONE',  ( 144.4983527463949713, -3576.390212577335205, 2245.979656122563938 ) ) ;
#8866=DIRECTION ( 'NONE',  ( 1.000000000000000000, 0.000000000000000000, 0.000000000000000000 ) ) ;
#8869=AXIS2_PLACEMENT_3D ( 'NONE', #73, #12723, #17994 ) ;
#8870=ORIENTED_EDGE ( 'NONE', *, *, #5118, .T. ) ;
#8871=CARTESIAN_POINT ( 'NONE',  ( 1.270000000000000018, -3694.430000000000291, 2259.329999999999927 ) ) ;
#8875=CARTESIAN_POINT ( 'NONE',  ( 20.62424768829000143, -3695.699999999999818, 2259.837999999999738 ) ) ;
#8876=CARTESIAN_POINT ( 'NONE',  ( 14.81100937555136987, -3657.598029303296244, 2248.669232965897208 ) ) ;
#8877=CARTESIAN_POINT ( 'NONE',  ( 136.7382561681559991, -3695.684722677371155, 2254.718515783431940 ) ) ;
#8880=LINE ( 'NONE', #7120, #3870 ) ;
#8883=DIRECTION ( 'NONE',  ( 1.224646799147353207E-16, 1.000000000000000000, -0.000000000000000000 ) ) ;
#8884=CARTESIAN_POINT ( 'NONE',  ( 101.5999999999999943, -3670.300000000000182, 2261.869999999999891 ) ) ;
#8886=CARTESIAN_POINT ( 'NONE',  ( 53.64479999999999649, -3670.300000000000182, 2261.869999999999891 ) ) ;
#8889=EDGE_CURVE ( 'NONE', #20430, #17962, #16648, .T. ) ;
#8890=DIRECTION ( 'NONE',  ( 0.000000000000000000, 1.000000000000000000, 0.000000000000000000 ) ) ;
#8891=EDGE_LOOP ( 'NONE', ( #19096, #1183 ) ) ;
#8892=DIRECTION ( 'NONE',  ( 1.000000000000000000, 0.000000000000000000, 0.000000000000000000 ) ) ;
#8895=AXIS2_PLACEMENT_3D ( 'NONE', #5777, #5657, #268 ) ;
#8898=CARTESIAN_POINT ( 'NONE',  ( 35.56000000000000227, -3568.700000000000273, 2250.236800000000130 ) ) ;
#8900=VERTEX_POINT ( 'NONE', #16769 ) ;
#8901=DIRECTION ( 'NONE',  ( 0.000000000000000000, 0.000000000000000000, -1.000000000000000000 ) ) ;
#8902=CARTESIAN_POINT ( 'NONE',  ( 151.1299999999999955, -3578.860000000000127, 2247.392000000000280 ) ) ;
#8904=ORIENTED_EDGE ( 'NONE', *, *, #20380, .T. ) ;
#8911=LINE ( 'NONE', #12656, #15270 ) ;
#8914=DIRECTION ( 'NONE',  ( 1.000000000000000000, 0.000000000000000000, 0.000000000000000000 ) ) ;
#8919=CARTESIAN_POINT ( 'NONE',  ( 4.769632180749402650, -3695.600514564973764, 2259.822746372431993 ) ) ;
#8920=EDGE_LOOP ( 'NONE', ( #10008, #4774, #11414, #14672 ) ) ;
#8922=CARTESIAN_POINT ( 'NONE',  ( 145.0128742528000032, -3657.399152860999493, 2246.630000000000109 ) ) ;
#8923=ORIENTED_EDGE ( 'NONE', *, *, #20342, .F. ) ;
#8924=DIRECTION ( 'NONE',  ( 0.8928571428588618630, -0.4503400076008236552, 0.000000000000000000 ) ) ;
#8927=ORIENTED_EDGE ( 'NONE', *, *, #5999, .T. ) ;
#8930=CARTESIAN_POINT ( 'NONE',  ( 1.270000000000000018, -3694.430000000000291, 2239.009999999999764 ) ) ;
#8934=DIRECTION ( 'NONE',  ( 0.000000000000000000, 0.000000000000000000, 1.000000000000000000 ) ) ;
#8936=EDGE_CURVE ( 'NONE', #21490, #5839, #1818, .T. ) ;
#8938=CARTESIAN_POINT ( 'NONE',  ( 10.15999999990231650, -3694.746619022270806, 2255.773999999897569 ) ) ;
#8939=ORIENTED_EDGE ( 'NONE', *, *, #9526, .F. ) ;
#8941=EDGE_CURVE ( 'NONE', #7082, #16518, #10752, .T. ) ;
#8946=DIRECTION ( 'NONE',  ( 0.000000000000000000, 0.000000000000000000, 1.000000000000000000 ) ) ;
#8949=ORIENTED_EDGE ( 'NONE', *, *, #5203, .F. ) ;
#8950=ORIENTED_EDGE ( 'NONE', *, *, #8384, .F. ) ;
#8951=FACE_OUTER_BOUND ( 'NONE', #13292, .T. ) ;
#8960=ORIENTED_EDGE ( 'NONE', *, *, #16870, .F. ) ;
#8962=FACE_BOUND ( 'NONE', #2729, .T. ) ;
#8967=VERTEX_POINT ( 'NONE', #1406 ) ;
#8970=DIRECTION ( 'NONE',  ( -1.000000000000000000, 0.000000000000000000, 0.000000000000000000 ) ) ;
#8971=ORIENTED_EDGE ( 'NONE', *, *, #20722, .F. ) ;
#8972=FACE_OUTER_BOUND ( 'NONE', #11772, .T. ) ;
#8973=CIRCLE ( 'NONE', #22054, 0.7619999999999294005 ) ;
#8975=CARTESIAN_POINT ( 'NONE',  ( 144.3372440649679049, -3576.154474778157237, 2246.502950162860998 ) ) ;
#8976=AXIS2_PLACEMENT_3D ( 'NONE', #9078, #21622, #5450 ) ;
#8977=CARTESIAN_POINT ( 'NONE',  ( 139.6999999999999886, -3659.504999999999654, 2239.009999999999764 ) ) ;
#8979=CARTESIAN_POINT ( 'NONE',  ( 18.24452305891707127, -3658.119603952914076, 2245.389097658092851 ) ) ;
#8982=DIRECTION ( 'NONE',  ( -1.000000000000000000, 0.000000000000000000, 0.000000000000000000 ) ) ;
#8984=CARTESIAN_POINT ( 'NONE',  ( 14.50229919307735571, -3657.303941002375723, 2247.615651459047967 ) ) ;
#8989=AXIS2_PLACEMENT_3D ( 'NONE', #212, #3951, #14742 ) ;
#8990=CARTESIAN_POINT ( 'NONE',  ( 1.270000000000000018, -3660.140000000000327, 2247.392000000000280 ) ) ;
#8993=FACE_OUTER_BOUND ( 'NONE', #20728, .T. ) ;
#8996=CARTESIAN_POINT ( 'NONE',  ( 104.4447999999999865, -3619.500000000000000, 2239.771999999999935 ) ) ;
#8997=FACE_OUTER_BOUND ( 'NONE', #8318, .T. ) ;
#8998=DIRECTION ( 'NONE',  ( 0.000000000000000000, 0.000000000000000000, -1.000000000000000000 ) ) ;
#8999=EDGE_CURVE ( 'NONE', #20116, #15997, #16002, .T. ) ;
#9004=VERTEX_POINT ( 'NONE', #16053 ) ;
#9005=CIRCLE ( 'NONE', #5259, 0.7619999999999294005 ) ;
#9006=FACE_OUTER_BOUND ( 'NONE', #16609, .T. ) ;
#9014=ORIENTED_EDGE ( 'NONE', *, *, #10451, .F. ) ;
#9017=ADVANCED_FACE ( 'NONE', ( #14648 ), #19569, .F. ) ;
#9018=EDGE_LOOP ( 'NONE', ( #22276, #14657, #10704, #1788 ) ) ;
#9020=CARTESIAN_POINT ( 'NONE',  ( 137.7360682368147877, -3581.553478357457152, 2248.308632888655666 ) ) ;
#9021=EDGE_LOOP ( 'NONE', ( #14223, #13741 ) ) ;
#9022=CARTESIAN_POINT ( 'NONE',  ( 95.25000000000000000, -3543.299999999999727, 2247.392000000000280 ) ) ;
#9024=CARTESIAN_POINT ( 'NONE',  ( 95.25000000000000000, -3695.699999999999818, 2247.392000000000280 ) ) ;
#9030=CARTESIAN_POINT ( 'NONE',  ( 139.4317159485291029, -3576.659585059088386, 2249.195327489805550 ) ) ;
#9032=TOROIDAL_SURFACE ( 'NONE', #22117, 4.114799999999999791, 1.270000000000000018 ) ;
#9033=CARTESIAN_POINT ( 'NONE',  ( 134.0531819916954248, -3578.609843495611130, 2244.556611876764237 ) ) ;
#9038=CARTESIAN_POINT ( 'NONE',  ( 20.09942059832000183, -3544.570000000000164, 2260.390449568000349 ) ) ;
#9045=DIRECTION ( 'NONE',  ( -1.000000000000000000, 0.000000000000000000, 0.000000000000000000 ) ) ;
#9046=TOROIDAL_SURFACE ( 'NONE', #7923, 4.114799999999999791, 1.270000000000000018 ) ;
#9047=CARTESIAN_POINT ( 'NONE',  ( 123.3932000000010021, -3619.500000000000000, 2239.771999999999935 ) ) ;
#9050=CARTESIAN_POINT ( 'NONE',  ( 1.270000000000000018, -3660.140000000000327, 2244.547199999999975 ) ) ;
#9051=DIRECTION ( 'NONE',  ( 0.000000000000000000, 0.000000000000000000, -1.000000000000000000 ) ) ;
#9054=CARTESIAN_POINT ( 'NONE',  ( 137.7383617481069109, -3657.443753316391849, 2248.304914619292504 ) ) ;
#9056=CARTESIAN_POINT ( 'NONE',  ( 137.5318703103976077, -3661.346907438663948, 2249.968155576829304 ) ) ;
#9058=ORIENTED_EDGE ( 'NONE', *, *, #19140, .F. ) ;
#9059=VERTEX_POINT ( 'NONE', #21674 ) ;
#9061=AXIS2_PLACEMENT_3D ( 'NONE', #21898, #5864, #13002 ) ;
#9063=AXIS2_PLACEMENT_3D ( 'NONE', #5726, #14741, #19898 ) ;
#9064=AXIS2_PLACEMENT_3D ( 'NONE', #14184, #19914, #5267 ) ;
#9066=EDGE_CURVE ( 'NONE', #22364, #15258, #7760, .T. ) ;
#9068=VERTEX_POINT ( 'NONE', #7046 ) ;
#9069=B_SPLINE_CURVE_WITH_KNOTS ( 'NONE', 3,
 ( #6974, #3441, #8374, #12351 ),
 .UNSPECIFIED., .F., .F.,
 ( 4, 4 ),
 ( 0.000000000000000000, 1.000000000000000000 ),
 .UNSPECIFIED. ) ;
#9071=EDGE_CURVE ( 'NONE', #19732, #10096, #19918, .T. ) ;
#9074=CARTESIAN_POINT ( 'NONE',  ( 139.6999999999999886, -3659.504999999999654, 2246.630000000000109 ) ) ;
#9077=DIRECTION ( 'NONE',  ( 1.000000000000000000, 0.000000000000000000, 0.000000000000000000 ) ) ;
#9078=CARTESIAN_POINT ( 'NONE',  ( 12.69999999999999929, -3579.494999999999891, 2239.009999999999764 ) ) ;
#9081=AXIS2_PLACEMENT_3D ( 'NONE', #5951, #11320, #11543 ) ;
#9084=CARTESIAN_POINT ( 'NONE',  ( 29.00679999999900005, -3670.300000000000182, 2239.009999999999764 ) ) ;
#9086=CIRCLE ( 'NONE', #5339, 2.844800000000001550 ) ;
#9088=AXIS2_PLACEMENT_3D ( 'NONE', #1478, #2775, #3009 ) ;
#9090=DIRECTION ( 'NONE',  ( 1.000000000000000000, 0.000000000000000000, 0.000000000000000000 ) ) ;
#9091=EDGE_LOOP ( 'NONE', ( #11659, #12428, #19516, #16525 ) ) ;
#9098=DIRECTION ( 'NONE',  ( 0.000000000000000000, 0.000000000000000000, -1.000000000000000000 ) ) ;
#9099=EDGE_CURVE ( 'NONE', #15748, #7197, #284, .T. ) ;
#9100=ORIENTED_EDGE ( 'NONE', *, *, #1850, .F. ) ;
#9103=TOROIDAL_SURFACE ( 'NONE', #19184, 3.606799999998999695, 0.7620000000000000107 ) ;
#9104=EDGE_CURVE ( 'NONE', #2862, #15378, #5153, .T. ) ;
#9106=EDGE_CURVE ( 'NONE', #10186, #20939, #21243, .T. ) ;
#9108=CYLINDRICAL_SURFACE ( 'NONE', #10834, 2.844800000000091700 ) ;
#9109=CARTESIAN_POINT ( 'NONE',  ( 142.6617438336326131, -3543.315277321872600, 2254.718515779005429 ) ) ;
#9110=CARTESIAN_POINT ( 'NONE',  ( 137.0453000019917056, -3695.234698871024193, 2255.486749946129748 ) ) ;
#9111=ORIENTED_EDGE ( 'NONE', *, *, #8005, .F. ) ;
#9112=CARTESIAN_POINT ( 'NONE',  ( 7.817606081005259000, -3576.524523609905373, 2245.767529109110455 ) ) ;
#9115=CARTESIAN_POINT ( 'NONE',  ( 1.270000000000000018, -3578.860000000000127, 2250.236800000000130 ) ) ;
#9119=CARTESIAN_POINT ( 'NONE',  ( 105.2067999999999870, -3619.500000000000000, 2239.771999999999935 ) ) ;
#9122=DIRECTION ( 'NONE',  ( -1.224646799147353207E-16, 1.000000000000000000, 0.000000000000000000 ) ) ;
#9126=ORIENTED_EDGE ( 'NONE', *, *, #15898, .T. ) ;
#9127=CARTESIAN_POINT ( 'NONE',  ( 47.19319999999999737, -3568.700000000000273, 2239.009999999999764 ) ) ;
#9129=ORIENTED_EDGE ( 'NONE', *, *, #15293, .T. ) ;
#9130=CYLINDRICAL_SURFACE ( 'NONE', #3546, 2.844800000000001550 ) ;
#9131=CIRCLE ( 'NONE', #14739, 0.7619999999999987894 ) ;
#9133=ORIENTED_EDGE ( 'NONE', *, *, #4910, .F. ) ;
#9134=CARTESIAN_POINT ( 'NONE',  ( 142.4684590622430846, -3695.492037865699785, 2255.201583320599184 ) ) ;
#9135=CARTESIAN_POINT ( 'NONE',  ( 142.5447969220999767, -3659.505006299999877, 2250.165025787000104 ) ) ;
#9136=EDGE_LOOP ( 'NONE', ( #18905, #17968, #2625, #2366, #18310, #12183 ) ) ;
#9137=EDGE_CURVE ( 'NONE', #9389, #19621, #17454, .T. ) ;
#9139=CARTESIAN_POINT ( 'NONE',  ( 137.9028742141985049, -3581.700239090842388, 2247.226065275468045 ) ) ;
#9142=DIRECTION ( 'NONE',  ( 0.000000000000000000, 0.000000000000000000, -1.000000000000000000 ) ) ;
#9143=CARTESIAN_POINT ( 'NONE',  ( 35.56000000000000227, -3694.430000000000291, 2247.392000000000280 ) ) ;
#9147=DIRECTION ( 'NONE',  ( -1.000000000000000000, 0.000000000000000000, 0.000000000000000000 ) ) ;
#9149=CARTESIAN_POINT ( 'NONE',  ( 138.2611185054702787, -3577.039135743023053, 2249.578612792418426 ) ) ;
#9151=CARTESIAN_POINT ( 'NONE',  ( 134.8157984830815224, -3576.527304683796956, 2245.762539383495550 ) ) ;
#9154=CARTESIAN_POINT ( 'NONE',  ( 127.0000000000000000, -3670.300000000000182, 2239.009999999999764 ) ) ;
#9158=ORIENTED_EDGE ( 'NONE', *, *, #3478, .T. ) ;
#9162=ORIENTED_EDGE ( 'NONE', *, *, #12641, .T. ) ;
#9165=DIRECTION ( 'NONE',  ( 0.000000000000000000, 0.000000000000000000, -1.000000000000000000 ) ) ;
#9167=VECTOR ( 'NONE', #5445, 1000.000000000000000 ) ;
#9168=FACE_OUTER_BOUND ( 'NONE', #5571, .T. ) ;
#9172=CARTESIAN_POINT ( 'NONE',  ( 20.62424768829000143, -3694.430000000000291, 2260.600000000000364 ) ) ;
#9173=CARTESIAN_POINT ( 'NONE',  ( 9.849683474922617421, -3695.600514565444882, 2254.996725890482594 ) ) ;
#9174=ORIENTED_EDGE ( 'NONE', *, *, #19700, .F. ) ;
#9175=CARTESIAN_POINT ( 'NONE',  ( 18.12475792849799205, -3581.293143188160229, 2245.917988635005713 ) ) ;
#9178=AXIS2_PLACEMENT_3D ( 'NONE', #5792, #19736, #5440 ) ;
#9180=CARTESIAN_POINT ( 'NONE',  ( 141.7787351652112591, -3661.447272802506632, 2249.918713514176034 ) ) ;
#9186=DIRECTION ( 'NONE',  ( 0.000000000000000000, 0.000000000000000000, -1.000000000000000000 ) ) ;
#9189=DIRECTION ( 'NONE',  ( -0.000000000000000000, -1.000000000000000000, -0.000000000000000000 ) ) ;
#9194=CARTESIAN_POINT ( 'NONE',  ( 7.298181435199534661, -3581.361247027800346, 2246.035952059512510 ) ) ;
#9197=DIRECTION ( 'NONE',  ( -0.000000000000000000, 1.000000000000000000, 0.000000000000000000 ) ) ;
#9200=ORIENTED_EDGE ( 'NONE', *, *, #1463, .T. ) ;
#9202=FACE_OUTER_BOUND ( 'NONE', #9303, .T. ) ;
#9208=ORIENTED_EDGE ( 'NONE', *, *, #4639, .F. ) ;
#9209=CARTESIAN_POINT ( 'NONE',  ( 117.9067999999989951, -3594.099999999999909, 2259.837999999999738 ) ) ;
#9210=TOROIDAL_SURFACE ( 'NONE', #16317, 3.606799999999999784, 0.7620000000000000107 ) ;
#9211=DIRECTION ( 'NONE',  ( 0.000000000000000000, 0.000000000000000000, 1.000000000000000000 ) ) ;
#9217=CARTESIAN_POINT ( 'NONE',  ( 139.6999999999999886, -3579.494999999999891, 2239.771999999999935 ) ) ;
#9219=CARTESIAN_POINT ( 'NONE',  ( 147.3450958631953256, -3694.826579461069286, 2260.537176449191975 ) ) ;
#9221=CARTESIAN_POINT ( 'NONE',  ( 38.10000000000000142, -3644.899999999999636, 2239.771999999999935 ) ) ;
#9222=CIRCLE ( 'NONE', #18559, 1.269999999999882334 ) ;
#9224=CARTESIAN_POINT ( 'NONE',  ( 114.2999999999999972, -3644.899999999999636, 2239.771999999999935 ) ) ;
#9225=CARTESIAN_POINT ( 'NONE',  ( 137.0970213875862385, -3695.048176949268964, 2255.616427087924876 ) ) ;
#9226=CARTESIAN_POINT ( 'NONE',  ( 7.481739961591920007, -3577.164555605966598, 2245.107626269509183 ) ) ;
#9230=FACE_OUTER_BOUND ( 'NONE', #9255, .T. ) ;
#9234=VECTOR ( 'NONE', #18507, 1000.000000000000000 ) ;
#9237=ADVANCED_FACE ( 'NONE', ( #12043 ), #3132, .T. ) ;
#9238=CARTESIAN_POINT ( 'NONE',  ( 134.6064618253988101, -3662.097549161604093, 2245.303073078320722 ) ) ;
#9240=VECTOR ( 'NONE', #8866, 1000.000000000000000 ) ;
#9241=ORIENTED_EDGE ( 'NONE', *, *, #11296, .F. ) ;
#9242=CARTESIAN_POINT ( 'NONE',  ( 88.90000000000000568, -3594.099999999999909, 2260.600000000000364 ) ) ;
#9250=ORIENTED_EDGE ( 'NONE', *, *, #10667, .T. ) ;
#9251=CARTESIAN_POINT ( 'NONE',  ( 142.3391137066397221, -3695.185487565168842, 2255.525687528044273 ) ) ;
#9252=DIRECTION ( 'NONE',  ( 0.000000000000000000, 0.000000000000000000, -1.000000000000000000 ) ) ;
#9254=TOROIDAL_SURFACE ( 'NONE', #9970, 3.606799999999999784, 0.7620000000000000107 ) ;
#9255=EDGE_LOOP ( 'NONE', ( #7857, #1319, #15370, #12041 ) ) ;
#9256=AXIS2_PLACEMENT_3D ( 'NONE', #188, #7224, #4047 ) ;
#9257=CARTESIAN_POINT ( 'NONE',  ( 137.2861954999169143, -3581.000367542877484, 2249.265958390819378 ) ) ;
#9259=ORIENTED_EDGE ( 'NONE', *, *, #1942, .T. ) ;
#9260=CARTESIAN_POINT ( 'NONE',  ( 123.3932000000010021, -3568.700000000000273, 2259.837999999999738 ) ) ;
#9262=CARTESIAN_POINT ( 'NONE',  ( 114.2999999999999972, -3644.899999999999636, 2260.600000000000364 ) ) ;
#9263=DIRECTION ( 'NONE',  ( 0.000000000000000000, 0.000000000000000000, 1.000000000000000000 ) ) ;
#9265=EDGE_CURVE ( 'NONE', #14824, #20865, #13556, .T. ) ;
#9267=CIRCLE ( 'NONE', #18995, 2.844800000000091700 ) ;
#9268=CARTESIAN_POINT ( 'NONE',  ( 142.0937630362152788, -3577.955592839939072, 2250.090245135924306 ) ) ;
#9272=CIRCLE ( 'NONE', #4759, 0.7619999999999294005 ) ;
#9274=TOROIDAL_SURFACE ( 'NONE', #11885, 6.477000000000000313, 0.7620000000000000107 ) ;
#9275=CARTESIAN_POINT ( 'NONE',  ( 1.270000000000000018, -3578.860000000000127, 2247.392000000000280 ) ) ;
#9279=ORIENTED_EDGE ( 'NONE', *, *, #5704, .F. ) ;
#9280=CARTESIAN_POINT ( 'NONE',  ( 4.572920519510000226, -3543.299999999999727, 2259.329999999999927 ) ) ;
#9282=AXIS2_PLACEMENT_3D ( 'NONE', #11103, #4602, #2201 ) ;
#9288=DIRECTION ( 'NONE',  ( -0.000000000000000000, -1.000000000000000000, -0.000000000000000000 ) ) ;
#9289=ADVANCED_FACE ( 'NONE', ( #12508 ), #19427, .F. ) ;
#9291=AXIS2_PLACEMENT_3D ( 'NONE', #5527, #125, #5283 ) ;
#9293=CARTESIAN_POINT ( 'NONE',  ( 12.69999999999999929, -3659.504999999999654, 2246.630000000000109 ) ) ;
#9295=CARTESIAN_POINT ( 'NONE',  ( 18.20689721057726373, -3581.023318642830418, 2245.544194210850492 ) ) ;
#9296=CARTESIAN_POINT ( 'NONE',  ( 137.5404010602593985, -3657.652756290912748, 2248.773912801639653 ) ) ;
#9299=CARTESIAN_POINT ( 'NONE',  ( 137.2437110623308456, -3660.940235422853675, 2250.121982768094313 ) ) ;
#9301=TOROIDAL_SURFACE ( 'NONE', #15653, 3.606799999998999695, 0.7620000000000000107 ) ;
#9303=EDGE_LOOP ( 'NONE', ( #8939, #10715, #8506, #21210 ) ) ;
#9304=EDGE_CURVE ( 'NONE', #14295, #21153, #12282, .T. ) ;
#9306=CARTESIAN_POINT ( 'NONE',  ( 139.6999999999999886, -3579.494999999999891, 2246.630000000000109 ) ) ;
#9307=ORIENTED_EDGE ( 'NONE', *, *, #16247, .T. ) ;
#9310=DIRECTION ( 'NONE',  ( -0.7249994335945011414, 0.000000000000000000, 0.6887494619146010688 ) ) ;
#9313=DIRECTION ( 'NONE',  ( 0.7249994335945011414, 6.337882393832011514E-14, -0.6887494619146010688 ) ) ;
#9317=ADVANCED_FACE ( 'NONE', ( #8993 ), #12640, .T. ) ;
#9319=AXIS2_PLACEMENT_3D ( 'NONE', #4083, #7829, #16952 ) ;
#9323=B_SPLINE_CURVE_WITH_KNOTS ( 'NONE', 3,
 ( #10734, #14372, #10498, #21517 ),
 .UNSPECIFIED., .F., .F.,
 ( 4, 4 ),
 ( 0.000000000000000000, 1.000000000000000000 ),
 .UNSPECIFIED. ) ;
#9326=FACE_OUTER_BOUND ( 'NONE', #2381, .T. ) ;
#9330=ORIENTED_EDGE ( 'NONE', *, *, #6816, .T. ) ;
#9331=CARTESIAN_POINT ( 'NONE',  ( 18.12252087484897345, -3657.700112227995760, 2245.929179952064260 ) ) ;
#9332=ORIENTED_EDGE ( 'NONE', *, *, #21318, .F. ) ;
#9333=CARTESIAN_POINT ( 'NONE',  ( 12.69999999999999929, -3579.494999999999891, 2246.630000000000109 ) ) ;
#9336=CARTESIAN_POINT ( 'NONE',  ( 1.270000000000000018, -3543.299999999999727, 2259.329999999999927 ) ) ;
#9337=FACE_OUTER_BOUND ( 'NONE', #20168, .T. ) ;
#9338=FACE_OUTER_BOUND ( 'NONE', #2935, .T. ) ;
#9339=FACE_OUTER_BOUND ( 'NONE', #19313, .T. ) ;
#9340=CARTESIAN_POINT ( 'NONE',  ( 7.562696255153550595, -3576.991455836282512, 2245.246524209903328 ) ) ;
#9343=CARTESIAN_POINT ( 'NONE',  ( 21.79320000000099711, -3568.700000000000273, 2239.771999999999935 ) ) ;
#9344=DIRECTION ( 'NONE',  ( -1.000000000000000000, 0.000000000000000000, 0.000000000000000000 ) ) ;
#9347=CARTESIAN_POINT ( 'NONE',  ( 151.1299999999999955, -3695.699999999999818, 2240.279999999999745 ) ) ;
#9350=CARTESIAN_POINT ( 'NONE',  ( 135.0627559351442244, -3662.845525222075139, 2246.502950163688183 ) ) ;
#9352=DIRECTION ( 'NONE',  ( 0.000000000000000000, 0.000000000000000000, 1.000000000000000000 ) ) ;
#9353=VERTEX_POINT ( 'NONE', #91 ) ;
#9354=DIRECTION ( 'NONE',  ( -1.000000000000000000, 0.000000000000000000, 0.000000000000000000 ) ) ;
#9356=FACE_OUTER_BOUND ( 'NONE', #854, .T. ) ;
#9362=CARTESIAN_POINT ( 'NONE',  ( 142.5377065954122315, -3695.586719555400578, 2255.028323494163942 ) ) ;
#9368=CARTESIAN_POINT ( 'NONE',  ( 137.8781067631969677, -3581.679898106256132, 2246.981755619571686 ) ) ;
#9370=CARTESIAN_POINT ( 'NONE',  ( 145.3610525455973175, -3580.284312841534302, 2244.927052815919069 ) ) ;
#9372=CARTESIAN_POINT ( 'NONE',  ( 18.41500000000100101, -3579.494999999999891, 2246.630000000000109 ) ) ;
#9373=EDGE_CURVE ( 'NONE', #16752, #10141, #7467, .T. ) ;
#9375=CARTESIAN_POINT ( 'NONE',  ( 50.79999999999999716, -3568.700000000000273, 2239.771999999999935 ) ) ;
#9376=CARTESIAN_POINT ( 'NONE',  ( 145.4149999978999972, -3659.505243078000149, 2244.618209833000492 ) ) ;
#9379=CARTESIAN_POINT ( 'NONE',  ( 141.0602533517877362, -3576.996034928207791, 2249.541273427662873 ) ) ;
#9382=CARTESIAN_POINT ( 'NONE',  ( 134.4872152579750377, -3577.152335362136455, 2245.116748440663287 ) ) ;
#9383=CIRCLE ( 'NONE', #765, 2.844800000000091700 ) ;
#9386=ORIENTED_EDGE ( 'NONE', *, *, #11677, .F. ) ;
#9387=DIRECTION ( 'NONE',  ( 1.224646799147353207E-16, 1.000000000000000000, -0.000000000000000000 ) ) ;
#9388=CARTESIAN_POINT ( 'NONE',  ( 15.51375058686055652, -3543.438632179887918, 2255.088298573608881 ) ) ;
#9389=VERTEX_POINT ( 'NONE', #10629 ) ;
#9390=DIRECTION ( 'NONE',  ( 0.000000000000000000, -1.000000000000000000, 0.000000000000000000 ) ) ;
#9392=EDGE_CURVE ( 'NONE', #12110, #2146, #8157, .T. ) ;
#9395=FACE_OUTER_BOUND ( 'NONE', #16100, .T. ) ;
#9396=CARTESIAN_POINT ( 'NONE',  ( 15.14732702124904407, -3578.044519771737669, 2250.117477721357773 ) ) ;
#9399=CARTESIAN_POINT ( 'NONE',  ( 57.14999999999999858, -3544.570000000000164, 2244.547199999999975 ) ) ;
#9406=ORIENTED_EDGE ( 'NONE', *, *, #18272, .F. ) ;
#9407=CARTESIAN_POINT ( 'NONE',  ( 18.16297020592579514, -3581.174070066103923, 2245.736054050092662 ) ) ;
#9409=AXIS2_PLACEMENT_3D ( 'NONE', #12469, #12238, #17734 ) ;
#9412=CARTESIAN_POINT ( 'NONE',  ( 139.8351778257380431, -3662.349770900797466, 2249.183591361917934 ) ) ;
#9413=ORIENTED_EDGE ( 'NONE', *, *, #18162, .F. ) ;
#9415=VERTEX_POINT ( 'NONE', #6491 ) ;
#9416=DIRECTION ( 'NONE',  ( 0.000000000000000000, 1.000000000000000000, 0.000000000000000000 ) ) ;
#9420=DIRECTION ( 'NONE',  ( 0.000000000000000000, 1.000000000000000000, 0.000000000000000000 ) ) ;
#9421=AXIS2_PLACEMENT_3D ( 'NONE', #11210, #4513, #2638 ) ;
#9422=ORIENTED_EDGE ( 'NONE', *, *, #8999, .T. ) ;
#9427=ADVANCED_FACE ( 'NONE', ( #12854 ), #1800, .T. ) ;
#9429=DIRECTION ( 'NONE',  ( -1.000000000000000000, 0.000000000000000000, 0.000000000000000000 ) ) ;
#9432=CARTESIAN_POINT ( 'NONE',  ( 142.5401018058971090, -3659.315465601250708, 2250.116512621371385 ) ) ;
#9436=CIRCLE ( 'NONE', #16538, 3.606799999999993567 ) ;
#9440=ORIENTED_EDGE ( 'NONE', *, *, #18659, .T. ) ;
#9441=EDGE_CURVE ( 'NONE', #10242, #3614, #10391, .T. ) ;
#9444=CARTESIAN_POINT ( 'NONE',  ( 147.3829786123148438, -3695.048176948414493, 2260.442427088400564 ) ) ;
#9448=CARTESIAN_POINT ( 'NONE',  ( 142.2706313854639291, -3544.133557167201616, 2255.697303096545056 ) ) ;
#9450=CIRCLE ( 'NONE', #12441, 0.7620000000000126672 ) ;
#9451=AXIS2_PLACEMENT_3D ( 'NONE', #11039, #14679, #21822 ) ;
#9455=CIRCLE ( 'NONE', #8699, 2.844799999998995244 ) ;
#9456=EDGE_CURVE ( 'NONE', #6511, #8337, #18666, .T. ) ;
#9457=CARTESIAN_POINT ( 'NONE',  ( 145.1107615082556777, -3657.665077820303395, 2245.989155495581599 ) ) ;
#9458=CARTESIAN_POINT ( 'NONE',  ( 9.995409801658235338, -3580.378055366828448, 2249.798395734993846 ) ) ;
#9459=DIRECTION ( 'NONE',  ( -1.224646799147353207E-16, 1.000000000000000000, 0.000000000000000000 ) ) ;
#9461=CIRCLE ( 'NONE', #4971, 2.873832635400752622 ) ;
#9464=ORIENTED_EDGE ( 'NONE', *, *, #10960, .F. ) ;
#9466=DIRECTION ( 'NONE',  ( -0.9999999999992201793, 1.248865928399024183E-06, 0.000000000000000000 ) ) ;
#9468=CYLINDRICAL_SURFACE ( 'NONE', #17800, 2.844799999999994444 ) ;
#9469=ORIENTED_EDGE ( 'NONE', *, *, #3938, .T. ) ;
#9471=ORIENTED_EDGE ( 'NONE', *, *, #4207, .F. ) ;
#9472=FACE_OUTER_BOUND ( 'NONE', #11924, .T. ) ;
#9473=CARTESIAN_POINT ( 'NONE',  ( 110.6932000000009992, -3594.099999999999909, 2239.009999999999764 ) ) ;
#9474=VECTOR ( 'NONE', #21227, 1000.000000000000000 ) ;
#9478=VERTEX_POINT ( 'NONE', #7579 ) ;
#9484=CARTESIAN_POINT ( 'NONE',  ( 142.2400000000000091, -3580.776127254000130, 2255.774000000000342 ) ) ;
#9487=EDGE_CURVE ( 'NONE', #6224, #18611, #13385, .T. ) ;
#9488=CARTESIAN_POINT ( 'NONE',  ( 139.1589808602738856, -3576.701270618950730, 2249.244916196757458 ) ) ;
#9489=ORIENTED_EDGE ( 'NONE', *, *, #16997, .T. ) ;
#9493=ORIENTED_EDGE ( 'NONE', *, *, #13083, .F. ) ;
#9495=CARTESIAN_POINT ( 'NONE',  ( 142.4431999999993366, -3658.626742952568293, 2255.967040000000907 ) ) ;
#9496=ORIENTED_EDGE ( 'NONE', *, *, #4435, .F. ) ;
#9500=ORIENTED_EDGE ( 'NONE', *, *, #17556, .F. ) ;
#9502=CARTESIAN_POINT ( 'NONE',  ( 11.95351013509671745, -3576.749823794578788, 2249.299903167124739 ) ) ;
#9506=AXIS2_PLACEMENT_3D ( 'NONE', #11577, #13582, #4441 ) ;
#9509=CARTESIAN_POINT ( 'NONE',  ( 127.0000000000000000, -3660.140000000000327, 2247.392000000000280 ) ) ;
#9510=FACE_OUTER_BOUND ( 'NONE', #7541, .T. ) ;
#9511=CARTESIAN_POINT ( 'NONE',  ( 20.56213590047408246, -3543.486725648842821, 2259.993682086426361 ) ) ;
#9513=EDGE_CURVE ( 'NONE', #15997, #20116, #7788, .T. ) ;
#9515=CARTESIAN_POINT ( 'NONE',  ( 138.0302948368629643, -3661.810155319285059, 2249.696016199272435 ) ) ;
#9516=EDGE_CURVE ( 'NONE', #22942, #10444, #675, .T. ) ;
#9523=ORIENTED_EDGE ( 'NONE', *, *, #8688, .F. ) ;
#9525=FACE_OUTER_BOUND ( 'NONE', #2878, .T. ) ;
#9526=EDGE_CURVE ( 'NONE', #5890, #2318, #10765, .T. ) ;
#9527=ORIENTED_EDGE ( 'NONE', *, *, #10113, .F. ) ;
#9528=CARTESIAN_POINT ( 'NONE',  ( 7.192890077382537939, -3657.977450208451501, 2245.543294774859532 ) ) ;
#9529=DIRECTION ( 'NONE',  ( 1.000000000000000000, 0.000000000000000000, 0.000000000000000000 ) ) ;
#9532=CARTESIAN_POINT ( 'NONE',  ( 116.8400000000000034, -3568.700000000000273, 2250.236800000000130 ) ) ;
#9538=CARTESIAN_POINT ( 'NONE',  ( 14.61266695128000137, -3657.399152860999493, 2246.630000000000109 ) ) ;
#9539=AXIS2_PLACEMENT_3D ( 'NONE', #13770, #20913, #4849 ) ;
#9542=ADVANCED_FACE ( 'NONE', ( #21763 ), #10106, .F. ) ;
#9545=DIRECTION ( 'NONE',  ( 1.000000000000000000, 0.000000000000000000, 0.000000000000000000 ) ) ;
#9548=EDGE_CURVE ( 'NONE', #7211, #3298, #16764, .T. ) ;
#9556=AXIS2_PLACEMENT_3D ( 'NONE', #18947, #15319, #15434 ) ;
#9558=AXIS2_PLACEMENT_3D ( 'NONE', #16305, #21808, #18174 ) ;
#9561=DIRECTION ( 'NONE',  ( -1.000000000000000000, 0.000000000000000000, 0.000000000000000000 ) ) ;
#9562=VERTEX_POINT ( 'NONE', #15969 ) ;
#9564=CARTESIAN_POINT ( 'NONE',  ( 145.0933512042157645, -3657.614374765385946, 2246.082311836971712 ) ) ;
#9569=ORIENTED_EDGE ( 'NONE', *, *, #7280, .F. ) ;
#9570=AXIS2_PLACEMENT_3D ( 'NONE', #14375, #19999, #5823 ) ;
#9571=CARTESIAN_POINT ( 'NONE',  ( 116.8400000000000034, -3568.700000000000273, 2247.392000000000280 ) ) ;
#9573=VECTOR ( 'NONE', #22583, 1000.000000000000000 ) ;
#9574=CIRCLE ( 'NONE', #19687, 3.606799999999993567 ) ;
#9575=DIRECTION ( 'NONE',  ( 0.000000000000000000, 0.000000000000000000, 1.000000000000000000 ) ) ;
#9578=CARTESIAN_POINT ( 'NONE',  ( 13.53726674519237250, -3662.223867174984662, 2249.328617614321047 ) ) ;
#9579=EDGE_CURVE ( 'NONE', #22364, #20612, #5942, .T. ) ;
#9583=CARTESIAN_POINT ( 'NONE',  ( 63.50000000000000000, -3594.099999999999909, 2260.600000000000364 ) ) ;
#9584=B_SPLINE_CURVE_WITH_KNOTS ( 'NONE', 3,
 ( #22404, #9655, #9432, #12943, #20210, #16794, #736, #20101, #16570, #7665, #14825, #5925, #11405, #4151, #2397, #16683, #20649, #6729, #11988, #4727, #15632, #13867, #13758, #10461, #8710, #11875, #8486, #6845, #21018, #22641, #19259, #6380, #11747, #1198, #22868, #9994, #15502, #1082, #1317, #15744, #17362, #12226, #13509, #20902, #3078, #4957, #8242, #6494, #12106, #4835, #8365, #19141, #22760, #6619, #3195, #5082, #10230, #19023, #13629, #10344, #17492, #13987, #1437, #19373, #8595, #21134, #3310 ),
 .UNSPECIFIED., .F., .F.,
 ( 4, 2, 1, 1, 2, 2, 2, 1, 1, 2, 2, 2, 2, 1, 1, 1, 2, 2, 2, 2, 1, 2, 2, 2, 2, 1, 1, 2, 2, 2, 2, 2, 2, 2, 2, 1, 2, 2, 4 ),
 ( 0.000000000000000000, 0.06249999999687816388, 0.09374999999549321616, 0.1093749999946744406, 0.1171874999942121715, 0.1249999999937499023, 0.1874999999894321756, 0.2187499999871572731, 0.2343749999860897937, 0.2421874999855584409, 0.2499999999850270604, 0.3124999999787857474, 0.3437499999755888047, 0.3593749999739168088, 0.3671874999730100342, 0.3710937499726200128, 0.3730468749724225042, 0.3749999999722250510, 0.4062499999690292740, 0.4218749999673663265, 0.4296874999666068784, 0.4335937499661114414, 0.4374999999656160043, 0.4687499999620942659, 0.4843749999603362832, 0.4921874999596303479, 0.4960937499594011424, 0.4980468749594834654, 0.4999999999595658440, 0.5624999999646774773, 0.5937499999673057083, 0.6093749999686635110, 0.6249999999700213138, 0.7499999999813724560, 0.8124999999870490264, 0.8437499999897181135, 0.8593749999908758541, 0.8749999999920334837, 1.000000000000000000 ),
 .UNSPECIFIED. ) ;
#9586=ORIENTED_EDGE ( 'NONE', *, *, #17142, .T. ) ;
#9587=CARTESIAN_POINT ( 'NONE',  ( 95.25000000000000000, -3694.430000000000291, 2243.277199999999993 ) ) ;
#9589=ORIENTED_EDGE ( 'NONE', *, *, #18567, .T. ) ;
#9599=ADVANCED_FACE ( 'NONE', ( #4832 ), #17844, .F. ) ;
#9600=DIRECTION ( 'NONE',  ( 0.000000000000000000, 0.000000000000000000, -1.000000000000000000 ) ) ;
#9601=CARTESIAN_POINT ( 'NONE',  ( 17.62147847323069172, -3662.410506574471583, 2245.677565646850780 ) ) ;
#9602=FACE_OUTER_BOUND ( 'NONE', #16653, .T. ) ;
#9606=VECTOR ( 'NONE', #31, 1000.000000000000000 ) ;
#9608=CARTESIAN_POINT ( 'NONE',  ( 136.9568000000001291, -3578.616742952567620, 2255.967039999999997 ) ) ;
#9610=DIRECTION ( 'NONE',  ( 1.000000000000000000, 0.000000000000000000, 0.000000000000000000 ) ) ;
#9611=AXIS2_PLACEMENT_3D ( 'NONE', #10288, #2911, #5024 ) ;
#9612=CARTESIAN_POINT ( 'NONE',  ( 15.24000000016591727, -3544.253380977658708, 2255.773999999824809 ) ) ;
#9616=CARTESIAN_POINT ( 'NONE',  ( 50.79999999999999716, -3670.300000000000182, 2259.837999999999738 ) ) ;
#9620=CARTESIAN_POINT ( 'NONE',  ( 14.29432915190223419, -3577.137138884523665, 2249.656628075460503 ) ) ;
#9621=CARTESIAN_POINT ( 'NONE',  ( 141.4881110317870423, -3581.707777077976971, 2247.291309677514619 ) ) ;
#9622=ORIENTED_EDGE ( 'NONE', *, *, #3055, .F. ) ;
#9627=ORIENTED_EDGE ( 'NONE', *, *, #1169, .T. ) ;
#9631=CIRCLE ( 'NONE', #7765, 3.606799999999993567 ) ;
#9635=ORIENTED_EDGE ( 'NONE', *, *, #2510, .T. ) ;
#9638=DIRECTION ( 'NONE',  ( -1.224646799147353207E-16, 1.000000000000000000, 0.000000000000000000 ) ) ;
#9644=CIRCLE ( 'NONE', #6667, 2.844800000000091700 ) ;
#9645=CARTESIAN_POINT ( 'NONE',  ( 7.025241774765377478, -3658.828171944931455, 2244.867706167576216 ) ) ;
#9648=DIRECTION ( 'NONE',  ( -1.000000000000000000, 0.000000000000000000, 0.000000000000000000 ) ) ;
#9650=DIRECTION ( 'NONE',  ( 0.000000000000000000, 1.000000000000000000, 0.000000000000000000 ) ) ;
#9652=EDGE_CURVE ( 'NONE', #20457, #11664, #6307, .T. ) ;
#9654=ORIENTED_EDGE ( 'NONE', *, *, #12250, .T. ) ;
#9655=CARTESIAN_POINT ( 'NONE',  ( 142.5447969220999767, -3659.410301963842812, 2250.143339135433507 ) ) ;
#9657=CARTESIAN_POINT ( 'NONE',  ( 72.59320000000001016, -3568.700000000000273, 2239.771999999999935 ) ) ;
#9659=ORIENTED_EDGE ( 'NONE', *, *, #11389, .F. ) ;
#9663=VERTEX_POINT ( 'NONE', #3538 ) ;
#9671=DIRECTION ( 'NONE',  ( 1.000000000000000000, 0.000000000000000000, 0.000000000000000000 ) ) ;
#9672=CYLINDRICAL_SURFACE ( 'NONE', #8343, 2.844800000000091700 ) ;
#9675=CARTESIAN_POINT ( 'NONE',  ( 20.42971111056401767, -3695.268694217237226, 2260.325313175604151 ) ) ;
#9676=EDGE_CURVE ( 'NONE', #11901, #11706, #2930, .T. ) ;
#9679=EDGE_CURVE ( 'NONE', #3220, #14115, #4419, .T. ) ;
#9681=DIRECTION ( 'NONE',  ( 1.273565328809000167E-14, 1.000000000000000000, -1.319970543219000025E-14 ) ) ;
#9683=DIRECTION ( 'NONE',  ( 1.000000000000000000, 0.000000000000000000, 0.000000000000000000 ) ) ;
#9684=VERTEX_POINT ( 'NONE', #3191 ) ;
#9686=FACE_OUTER_BOUND ( 'NONE', #12154, .T. ) ;
#9688=CIRCLE ( 'NONE', #9319, 2.844800000000001550 ) ;
#9690=CARTESIAN_POINT ( 'NONE',  ( 14.46545461912941022, -3661.735746247042243, 2249.747105226763779 ) ) ;
#9693=FACE_OUTER_BOUND ( 'NONE', #16791, .T. ) ;
#9695=CARTESIAN_POINT ( 'NONE',  ( 114.2999999999999972, -3644.899999999999636, 2261.869999999999891 ) ) ;
#9696=CARTESIAN_POINT ( 'NONE',  ( 25.39999999999999858, -3670.300000000000182, 2259.837999999999738 ) ) ;
#9698=ORIENTED_EDGE ( 'NONE', *, *, #22934, .T. ) ;
#9699=AXIS2_PLACEMENT_3D ( 'NONE', #6874, #8622, #3457 ) ;
#9703=CARTESIAN_POINT ( 'NONE',  ( 145.2664576437646815, -3580.789478182276071, 2245.301509789881493 ) ) ;
#9705=EDGE_CURVE ( 'NONE', #5314, #1446, #1263, .T. ) ;
#9709=CARTESIAN_POINT ( 'NONE',  ( 17.57087389318388659, -3662.494267584890622, 2245.794996442214597 ) ) ;
#9710=DIRECTION ( 'NONE',  ( 0.000000000000000000, 0.000000000000000000, -1.000000000000000000 ) ) ;
#9712=DIRECTION ( 'NONE',  ( 1.000000000000000000, 0.000000000000000000, 0.000000000000000000 ) ) ;
#9713=EDGE_CURVE ( 'NONE', #14933, #11901, #5133, .T. ) ;
#9714=EDGE_LOOP ( 'NONE', ( #15112, #14067 ) ) ;
#9717=EDGE_LOOP ( 'NONE', ( #5862, #2767, #14349, #23107 ) ) ;
#9719=CARTESIAN_POINT ( 'NONE',  ( 18.41519309054999809, -3659.710859637462363, 2244.571829071724096 ) ) ;
#9721=CARTESIAN_POINT ( 'NONE',  ( 10.87796901928627058, -3657.320223683514996, 2246.982647036138587 ) ) ;
#9725=EDGE_LOOP ( 'NONE', ( #18478, #65, #22329, #11018 ) ) ;
#9727=ORIENTED_EDGE ( 'NONE', *, *, #526, .T. ) ;
#9729=CARTESIAN_POINT ( 'NONE',  ( 15.28019367547714680, -3578.294426589508930, 2250.180878883692458 ) ) ;
#9731=CARTESIAN_POINT ( 'NONE',  ( 142.3050992937297110, -3580.638258740797937, 2249.612730726536029 ) ) ;
#9732=ORIENTED_EDGE ( 'NONE', *, *, #19582, .F. ) ;
#9735=CARTESIAN_POINT ( 'NONE',  ( 1.270000000000000018, -3694.430000000000291, 2259.329999999999927 ) ) ;
#9737=CARTESIAN_POINT ( 'NONE',  ( 20.70572851130767233, -3543.336642707656665, 2259.634237443121492 ) ) ;
#9739=EDGE_LOOP ( 'NONE', ( #622, #1465, #15692, #7422 ) ) ;
#9744=EDGE_LOOP ( 'NONE', ( #5905, #8596, #21355, #3042 ) ) ;
#9747=DIRECTION ( 'NONE',  ( 1.000000000000000000, 0.000000000000000000, 0.000000000000000000 ) ) ;
#9751=DIRECTION ( 'NONE',  ( 0.000000000000000000, 0.000000000000000000, 1.000000000000000000 ) ) ;
#9753=CARTESIAN_POINT ( 'NONE',  ( 12.69999999999999929, -3659.504999999999654, 2239.009999999999764 ) ) ;
#9756=DIRECTION ( 'NONE',  ( 0.000000000000000000, 0.000000000000000000, -1.000000000000000000 ) ) ;
#9757=DIRECTION ( 'NONE',  ( -1.000000000000000000, 0.000000000000000000, 0.000000000000000000 ) ) ;
#9760=FACE_OUTER_BOUND ( 'NONE', #11025, .T. ) ;
#9766=AXIS2_PLACEMENT_3D ( 'NONE', #16817, #4062, #15189 ) ;
#9770=CARTESIAN_POINT ( 'NONE',  ( 105.2067999999999870, -3568.700000000000273, 2239.771999999999935 ) ) ;
#9773=FACE_OUTER_BOUND ( 'NONE', #18425, .T. ) ;
#9777=DIRECTION ( 'NONE',  ( -1.000000000000000000, 0.000000000000000000, 0.000000000000000000 ) ) ;
#9778=CARTESIAN_POINT ( 'NONE',  ( 20.75836682411413747, -3695.690215920803439, 2259.501687144741027 ) ) ;
#9779=ORIENTED_EDGE ( 'NONE', *, *, #5081, .T. ) ;
#9781=VERTEX_POINT ( 'NONE', #1793 ) ;
#9783=AXIS2_PLACEMENT_3D ( 'NONE', #7210, #300, #10837 ) ;
#9784=CIRCLE ( 'NONE', #2326, 3.606800000000000228 ) ;
#9787=ORIENTED_EDGE ( 'NONE', *, *, #12250, .F. ) ;
#9788=CARTESIAN_POINT ( 'NONE',  ( 9.855199999999999960, -3579.494999999999891, 2272.030000000000200 ) ) ;
#9794=CARTESIAN_POINT ( 'NONE',  ( 40.94480000000000075, -3644.899999999999636, 2239.771999999999935 ) ) ;
#9796=CIRCLE ( 'NONE', #19920, 2.844799999999994444 ) ;
#9797=EDGE_CURVE ( 'NONE', #4689, #3037, #6352, .T. ) ;
#9798=DIRECTION ( 'NONE',  ( -1.000000000000000000, 0.000000000000000000, 0.000000000000000000 ) ) ;
#9799=ORIENTED_EDGE ( 'NONE', *, *, #20109, .F. ) ;
#9801=DIRECTION ( 'NONE',  ( 0.000000000000000000, 0.000000000000000000, 1.000000000000000000 ) ) ;
#9804=CIRCLE ( 'NONE', #823, 0.7619999999999987894 ) ;
#9805=CARTESIAN_POINT ( 'NONE',  ( 151.4000000000000057, -3660.140000000000327, 2247.392000000000280 ) ) ;
#9806=DIRECTION ( 'NONE',  ( -1.000000000000000000, 0.000000000000000000, 0.000000000000000000 ) ) ;
#9808=VERTEX_POINT ( 'NONE', #22379 ) ;
#9810=DIRECTION ( 'NONE',  ( 0.000000000000000000, 0.000000000000000000, -1.000000000000000000 ) ) ;
#9816=FACE_OUTER_BOUND ( 'NONE', #7911, .T. ) ;
#9817=CARTESIAN_POINT ( 'NONE',  ( 18.37893127878000143, -3660.140301727999940, 2244.547200027999679 ) ) ;
#9821=VECTOR ( 'NONE', #22750, 1000.000000000000000 ) ;
#9822=CARTESIAN_POINT ( 'NONE',  ( 63.50000000000000000, -3594.099999999999909, 2239.771999999999935 ) ) ;
#9825=EDGE_CURVE ( 'NONE', #16546, #10242, #1422, .T. ) ;
#9826=DIRECTION ( 'NONE',  ( 0.000000000000000000, 0.000000000000000000, -1.000000000000000000 ) ) ;
#9827=VERTEX_POINT ( 'NONE', #11601 ) ;
#9829=CARTESIAN_POINT ( 'NONE',  ( 15.40195214416352876, -3543.639179024606165, 2255.368362556376724 ) ) ;
#9831=EDGE_CURVE ( 'NONE', #553, #8199, #22493, .T. ) ;
#9833=EDGE_CURVE ( 'NONE', #2616, #15095, #11120, .T. ) ;
#9835=ORIENTED_EDGE ( 'NONE', *, *, #5148, .F. ) ;
#9840=CARTESIAN_POINT ( 'NONE',  ( 14.86805197786120480, -3577.652999197129247, 2249.968111766196216 ) ) ;
#9843=ORIENTED_EDGE ( 'NONE', *, *, #12964, .F. ) ;
#9846=CARTESIAN_POINT ( 'NONE',  ( 38.10000000000000142, -3594.099999999999909, 2260.600000000000364 ) ) ;
#9847=DIRECTION ( 'NONE',  ( 1.122008997397786234E-13, 0.000000000000000000, -1.000000000000000000 ) ) ;
#9850=DIRECTION ( 'NONE',  ( 0.000000000000000000, 0.000000000000000000, 1.000000000000000000 ) ) ;
#9851=EDGE_CURVE ( 'NONE', #3037, #18991, #4302, .T. ) ;
#9853=ORIENTED_EDGE ( 'NONE', *, *, #4229, .T. ) ;
#9855=LINE ( 'NONE', #18879, #10313 ) ;
#9862=DIRECTION ( 'NONE',  ( 1.000000000000000000, 0.000000000000000000, 0.000000000000000000 ) ) ;
#9863=DIRECTION ( 'NONE',  ( 0.000000000000000000, 1.000000000000000000, 0.000000000000000000 ) ) ;
#9864=AXIS2_PLACEMENT_3D ( 'NONE', #4330, #18621, #9712 ) ;
#9866=CARTESIAN_POINT ( 'NONE',  ( 7.135618720840391838, -3658.201644552495509, 2245.309768844839255 ) ) ;
#9868=CYLINDRICAL_SURFACE ( 'NONE', #12611, 2.844800000000091700 ) ;
#9872=EDGE_CURVE ( 'NONE', #18081, #13878, #4008, .T. ) ;
#9875=ORIENTED_EDGE ( 'NONE', *, *, #13083, .T. ) ;
#9877=CARTESIAN_POINT ( 'NONE',  ( 50.79999999999999716, -3670.300000000000182, 2260.600000000000364 ) ) ;
#9880=CARTESIAN_POINT ( 'NONE',  ( 50.79999999999999716, -3568.700000000000273, 2239.771999999999935 ) ) ;
#9881=FACE_OUTER_BOUND ( 'NONE', #17161, .T. ) ;
#9882=EDGE_LOOP ( 'NONE', ( #12753, #160, #22116, #19533 ) ) ;
#9883=EDGE_LOOP ( 'NONE', ( #20099, #3324, #1705, #9208 ) ) ;
#9885=CARTESIAN_POINT ( 'NONE',  ( 20.12315942193000140, -3694.472271328999796, 2260.413001451000127 ) ) ;
#9889=CARTESIAN_POINT ( 'NONE',  ( 18.37960467573999779, -3578.859731361000286, 2244.547525601999951 ) ) ;
#9892=ORIENTED_EDGE ( 'NONE', *, *, #11984, .F. ) ;
#9894=ORIENTED_EDGE ( 'NONE', *, *, #2542, .T. ) ;
#9896=CARTESIAN_POINT ( 'NONE',  ( 10.16000000000000014, -3578.213872745999652, 2255.774000000000342 ) ) ;
#9898=CARTESIAN_POINT ( 'NONE',  ( 9.855099624826999971, -3659.505002774999411, 2250.165042250000170 ) ) ;
#9904=CARTESIAN_POINT ( 'NONE',  ( 144.7839377732694288, -3662.117457879833637, 2245.342794673845219 ) ) ;
#9905=ORIENTED_EDGE ( 'NONE', *, *, #799, .F. ) ;
#9906=LINE ( 'NONE', #20472, #6620 ) ;
#9908=CARTESIAN_POINT ( 'NONE',  ( 15.05122374280866815, -3661.108641140468990, 2250.067759433852189 ) ) ;
#9909=AXIS2_PLACEMENT_3D ( 'NONE', #14752, #21779, #20145 ) ;
#9910=CARTESIAN_POINT ( 'NONE',  ( 124.1552000000010025, -3568.700000000000273, 2261.869999999999891 ) ) ;
#9913=CARTESIAN_POINT ( 'NONE',  ( 145.0128742528999908, -3581.600847139000052, 2246.630000000000109 ) ) ;
#9916=CYLINDRICAL_SURFACE ( 'NONE', #11931, 5.714999999999999858 ) ;
#9917=CARTESIAN_POINT ( 'NONE',  ( 15.48868721613555977, -3658.939971329327818, 2249.971339383300347 ) ) ;
#9922=LINE ( 'NONE', #686, #5767 ) ;
#9924=CIRCLE ( 'NONE', #5845, 1.269999999999882334 ) ;
#9927=ADVANCED_FACE ( 'NONE', ( #13839 ), #9301, .T. ) ;
#9928=DIRECTION ( 'NONE',  ( -1.000000000000000000, 0.000000000000000000, 0.000000000000000000 ) ) ;
#9929=CIRCLE ( 'NONE', #6596, 3.606799999999001027 ) ;
#9930=DIRECTION ( 'NONE',  ( 1.000000000000000000, 0.000000000000000000, 0.000000000000000000 ) ) ;
#9931=CARTESIAN_POINT ( 'NONE',  ( 17.69701424773149512, -3662.279354287278238, 2245.514279573343629 ) ) ;
#9933=CARTESIAN_POINT ( 'NONE',  ( 15.54479999999999862, -3659.504999999999654, 2256.063560000000052 ) ) ;
#9939=CARTESIAN_POINT ( 'NONE',  ( 18.41499999999999915, -3659.504999999999654, 2239.771999999999935 ) ) ;
#9940=ORIENTED_EDGE ( 'NONE', *, *, #20465, .T. ) ;
#9942=AXIS2_PLACEMENT_3D ( 'NONE', #12002, #10241, #8729 ) ;
#9943=CARTESIAN_POINT ( 'NONE',  ( 142.7470794804999912, -3543.299999999999727, 2254.503999999999905 ) ) ;
#9944=CARTESIAN_POINT ( 'NONE',  ( 10.08643964193837661, -3658.381561134523054, 2249.628385529651496 ) ) ;
#9946=VERTEX_POINT ( 'NONE', #4810 ) ;
#9956=VECTOR ( 'NONE', #11787, 1000.000000000000000 ) ;
#9958=CARTESIAN_POINT ( 'NONE',  ( 141.9245196256013060, -3581.268366753078681, 2248.906305629936924 ) ) ;
#9959=ORIENTED_EDGE ( 'NONE', *, *, #16821, .F. ) ;
#9964=CARTESIAN_POINT ( 'NONE',  ( 67.10679999999999268, -3594.099999999999909, 2239.771999999999935 ) ) ;
#9965=EDGE_CURVE ( 'NONE', #20114, #16063, #2070, .T. ) ;
#9966=DIRECTION ( 'NONE',  ( 0.000000000000000000, 0.000000000000000000, 1.000000000000000000 ) ) ;
#9967=VECTOR ( 'NONE', #7652, 1000.000000000000000 ) ;
#9968=EDGE_CURVE ( 'NONE', #9781, #14341, #20848, .T. ) ;
#9969=ORIENTED_EDGE ( 'NONE', *, *, #21014, .T. ) ;
#9970=AXIS2_PLACEMENT_3D ( 'NONE', #6097, #13224, #20373 ) ;
#9971=CIRCLE ( 'NONE', #11477, 4.114799999999974034 ) ;
#9974=B_SPLINE_CURVE_WITH_KNOTS ( 'NONE', 3,
 ( #22124, #14764, #20156, #4324, #11464, #16847, #791, #4093, #7957, #15107 ),
 .UNSPECIFIED., .F., .F.,
 ( 4, 2, 1, 1, 2, 4 ),
 ( 0.000000000000000000, 0.06250000000027773617, 0.1250000000005554723, 0.2500000000010659806, 0.5000000000000244249, 1.000000000000000000 ),
 .UNSPECIFIED. ) ;
#9976=CARTESIAN_POINT ( 'NONE',  ( 142.2400000000000091, -3694.430000000000291, 2255.774000000000342 ) ) ;
#9977=VERTEX_POINT ( 'NONE', #21677 ) ;
#9980=CIRCLE ( 'NONE', #23074, 2.844800000000091700 ) ;
#9982=VERTEX_POINT ( 'NONE', #11011 ) ;
#9983=TOROIDAL_SURFACE ( 'NONE', #7740, 4.114799999999999791, 1.270000000000000018 ) ;
#9986=CARTESIAN_POINT ( 'NONE',  ( 117.9067999999989951, -3594.099999999999909, 2239.771999999999935 ) ) ;
#9987=DIRECTION ( 'NONE',  ( 0.000000000000000000, 0.000000000000000000, 1.000000000000000000 ) ) ;
#9989=AXIS2_PLACEMENT_3D ( 'NONE', #18337, #20217, #21518 ) ;
#9990=DIRECTION ( 'NONE',  ( 0.000000000000000000, 0.000000000000000000, -1.000000000000000000 ) ) ;
#9993=CARTESIAN_POINT ( 'NONE',  ( 116.8400000000000034, -3544.570000000000164, 2251.506800000000112 ) ) ;
#9994=CARTESIAN_POINT ( 'NONE',  ( 141.9598072415896866, -3657.776943722216402, 2248.975963221890197 ) ) ;
#9996=DIRECTION ( 'NONE',  ( 0.000000000000000000, 0.000000000000000000, -1.000000000000000000 ) ) ;
#9997=EDGE_CURVE ( 'NONE', #2232, #17371, #17085, .T. ) ;
#9999=CARTESIAN_POINT ( 'NONE',  ( 137.0230254594939368, -3543.701815209647521, 2255.430976451319566 ) ) ;
#10000=CIRCLE ( 'NONE', #8895, 2.844799999998995244 ) ;
#10001=ORIENTED_EDGE ( 'NONE', *, *, #10302, .T. ) ;
#10002=EDGE_CURVE ( 'NONE', #15239, #12110, #1762, .T. ) ;
#10003=VERTEX_POINT ( 'NONE', #5280 ) ;
#10005=CIRCLE ( 'NONE', #17862, 2.844799999998995244 ) ;
#10006=CYLINDRICAL_SURFACE ( 'NONE', #13650, 1.269999999999882334 ) ;
#10007=CIRCLE ( 'NONE', #12263, 3.606800000000000228 ) ;
#10008=ORIENTED_EDGE ( 'NONE', *, *, #1635, .F. ) ;
#10009=ORIENTED_EDGE ( 'NONE', *, *, #19286, .T. ) ;
#10013=ADVANCED_FACE ( 'NONE', ( #246 ), #1996, .F. ) ;
#10015=EDGE_CURVE ( 'NONE', #8026, #16063, #7757, .T. ) ;
#10024=LINE ( 'NONE', #17165, #15025 ) ;
#10026=CARTESIAN_POINT ( 'NONE',  ( 10.59475168835936998, -3581.408331351744437, 2248.656493541727286 ) ) ;
#10029=FACE_BOUND ( 'NONE', #2014, .T. ) ;
#10030=CARTESIAN_POINT ( 'NONE',  ( 35.56000000000000227, -3670.300000000000182, 2250.236800000000130 ) ) ;
#10031=CARTESIAN_POINT ( 'NONE',  ( 145.1668838676556561, -3661.170433021055032, 2244.740127772376582 ) ) ;
#10033=CARTESIAN_POINT ( 'NONE',  ( 12.69999999999999929, -3579.494999999999891, 2255.774000000000342 ) ) ;
#10034=CARTESIAN_POINT ( 'NONE',  ( 14.85464569033375781, -3661.362555271571637, 2249.960724679396208 ) ) ;
#10037=DIRECTION ( 'NONE',  ( 0.000000000000000000, 0.000000000000000000, -1.000000000000000000 ) ) ;
#10043=ORIENTED_EDGE ( 'NONE', *, *, #76, .F. ) ;
#10048=CARTESIAN_POINT ( 'NONE',  ( 117.1447999999989946, -3644.899999999999636, 2259.837999999999738 ) ) ;
#10050=AXIS2_PLACEMENT_3D ( 'NONE', #11228, #4532, #11671 ) ;
#10054=CARTESIAN_POINT ( 'NONE',  ( 136.9269754645999910, -3578.860002036999958, 2250.236803302000226 ) ) ;
#10055=ORIENTED_EDGE ( 'NONE', *, *, #5146, .T. ) ;
#10058=DIRECTION ( 'NONE',  ( 1.000000000000000000, 0.000000000000000000, 0.000000000000000000 ) ) ;
#10061=DIRECTION ( 'NONE',  ( 0.7249994335945011414, 6.337882393832011514E-14, 0.6887494619146010688 ) ) ;
#10065=ORIENTED_EDGE ( 'NONE', *, *, #16169, .F. ) ;
#10066=CARTESIAN_POINT ( 'NONE',  ( 134.2797385147190710, -3581.306672009827707, 2245.940466658847981 ) ) ;
#10071=CARTESIAN_POINT ( 'NONE',  ( 142.3965585763085642, -3580.405385417485377, 2249.782477816118899 ) ) ;
#10072=VERTEX_POINT ( 'NONE', #19923 ) ;
#10075=DIRECTION ( 'NONE',  ( -1.000000000000000000, 0.000000000000000000, 0.000000000000000000 ) ) ;
#10076=CARTESIAN_POINT ( 'NONE',  ( 14.62656071289291404, -3581.588169671847027, 2248.198601268956281 ) ) ;
#10078=CARTESIAN_POINT ( 'NONE',  ( 134.2752418639106509, -3657.706857388223852, 2245.917987683012143 ) ) ;
#10080=VERTEX_POINT ( 'NONE', #21572 ) ;
#10082=CARTESIAN_POINT ( 'NONE',  ( 142.4066795037432485, -3660.429743292840158, 2250.236799901205814 ) ) ;
#10084=EDGE_CURVE ( 'NONE', #19890, #22201, #9980, .T. ) ;
#10088=ADVANCED_FACE ( 'NONE', ( #5526 ), #19807, .T. ) ;
#10092=ORIENTED_EDGE ( 'NONE', *, *, #19838, .T. ) ;
#10095=CIRCLE ( 'NONE', #17201, 0.7619999999999294005 ) ;
#10096=VERTEX_POINT ( 'NONE', #14652 ) ;
#10106=PLANE ( 'NONE',  #6681 ) ;
#10110=ORIENTED_EDGE ( 'NONE', *, *, #11208, .F. ) ;
#10111=CARTESIAN_POINT ( 'NONE',  ( 137.1599999999999966, -3544.570000000000164, 2255.774000000000342 ) ) ;
#10113=EDGE_CURVE ( 'NONE', #15883, #2915, #581, .T. ) ;
#10116=ORIENTED_EDGE ( 'NONE', *, *, #2100, .T. ) ;
#10117=CARTESIAN_POINT ( 'NONE',  ( 4.770976268947110022, -3695.599092773176380, 2259.826110292242447 ) ) ;
#10121=CARTESIAN_POINT ( 'NONE',  ( 76.20000000000000284, -3670.300000000000182, 2259.837999999999738 ) ) ;
#10122=CARTESIAN_POINT ( 'NONE',  ( 142.2400000000000091, -3544.570000000000164, 2255.774000000000342 ) ) ;
#10124=ADVANCED_FACE ( 'NONE', ( #4094 ), #2110, .T. ) ;
#10125=ORIENTED_EDGE ( 'NONE', *, *, #5725, .F. ) ;
#10126=ADVANCED_FACE ( 'NONE', ( #6094 ), #11684, .F. ) ;
#10127=CARTESIAN_POINT ( 'NONE',  ( 130.6067999999989979, -3568.700000000000273, 2239.009999999999764 ) ) ;
#10130=DIRECTION ( 'NONE',  ( -1.000000000000000000, 0.000000000000000000, 0.000000000000000000 ) ) ;
#10131=CARTESIAN_POINT ( 'NONE',  ( 20.60962197524936457, -3695.579402567507259, 2259.874448544494044 ) ) ;
#10137=EDGE_CURVE ( 'NONE', #3108, #11298, #926, .T. ) ;
#10139=DIRECTION ( 'NONE',  ( -1.000000000000000000, 0.000000000000000000, 0.000000000000000000 ) ) ;
#10141=VERTEX_POINT ( 'NONE', #13344 ) ;
#10146=DIRECTION ( 'NONE',  ( 0.000000000000000000, 0.000000000000000000, 1.000000000000000000 ) ) ;
#10147=CARTESIAN_POINT ( 'NONE',  ( 145.1120077101980712, -3661.341326264781856, 2244.812092251788727 ) ) ;
#10148=CARTESIAN_POINT ( 'NONE',  ( 57.14999999999999858, -3568.700000000000273, 2247.392000000000280 ) ) ;
#10149=CARTESIAN_POINT ( 'NONE',  ( 11.74244832569119623, -3662.185093235403201, 2249.370122485771844 ) ) ;
#10150=CARTESIAN_POINT ( 'NONE',  ( 79.04479999999999507, -3568.700000000000273, 2239.771999999999935 ) ) ;
#10152=DIRECTION ( 'NONE',  ( -1.000000000000000000, 0.000000000000000000, 0.000000000000000000 ) ) ;
#10154=EDGE_CURVE ( 'NONE', #15928, #22036, #17544, .T. ) ;
#10157=DIRECTION ( 'NONE',  ( 0.000000000000000000, 0.000000000000000000, -1.000000000000000000 ) ) ;
#10158=VERTEX_POINT ( 'NONE', #3022 ) ;
#10159=AXIS2_PLACEMENT_3D ( 'NONE', #8990, #16141, #14274 ) ;
#10160=ORIENTED_EDGE ( 'NONE', *, *, #6510, .T. ) ;
#10161=VECTOR ( 'NONE', #2832, 1000.000000000000000 ) ;
#10163=ORIENTED_EDGE ( 'NONE', *, *, #13381, .T. ) ;
#10164=CARTESIAN_POINT ( 'NONE',  ( 9.916876041047901325, -3543.482543405149954, 2255.165366398012793 ) ) ;
#10165=DIRECTION ( 'NONE',  ( 0.000000000000000000, 0.000000000000000000, 1.000000000000000000 ) ) ;
#10168=DIRECTION ( 'NONE',  ( 0.000000000000000000, 1.000000000000000000, 1.224646799147353207E-16 ) ) ;
#10169=CYLINDRICAL_SURFACE ( 'NONE', #16714, 2.844799999999009010 ) ;
#10170=DIRECTION ( 'NONE',  ( 0.000000000000000000, 0.000000000000000000, -1.000000000000000000 ) ) ;
#10180=ORIENTED_EDGE ( 'NONE', *, *, #21483, .F. ) ;
#10184=ORIENTED_EDGE ( 'NONE', *, *, #6233, .F. ) ;
#10186=VERTEX_POINT ( 'NONE', #20715 ) ;
#10187=DIRECTION ( 'NONE',  ( 0.000000000000000000, 0.000000000000000000, 1.000000000000000000 ) ) ;
#10189=DIRECTION ( 'NONE',  ( 0.7249994335945011414, 0.000000000000000000, 0.6887494619146010688 ) ) ;
#10190=TOROIDAL_SURFACE ( 'NONE', #1199, 3.606799999998999695, 0.7620000000000000107 ) ;
#10192=CIRCLE ( 'NONE', #19925, 4.114799999999974034 ) ;
#10195=CIRCLE ( 'NONE', #2343, 2.844800000000001550 ) ;
#10197=DIRECTION ( 'NONE',  ( -0.000000000000000000, -1.000000000000000000, -0.000000000000000000 ) ) ;
#10198=CARTESIAN_POINT ( 'NONE',  ( 14.56067386347176651, -3581.648071076505403, 2246.799892842011559 ) ) ;
#10199=CARTESIAN_POINT ( 'NONE',  ( 134.1386338306796802, -3658.188830379587216, 2245.321775082328259 ) ) ;
#10202=CIRCLE ( 'NONE', #19196, 0.7620000000000126672 ) ;
#10203=CARTESIAN_POINT ( 'NONE',  ( 15.24000000000000021, -3694.746619018625552, 2255.774000000000342 ) ) ;
#10207=TOROIDAL_SURFACE ( 'NONE', #17313, 3.606799999998999695, 0.7620000000000000107 ) ;
#10211=CARTESIAN_POINT ( 'NONE',  ( 20.43202024788000060, -3544.321224513000288, 2260.577432830999896 ) ) ;
#10215=DIRECTION ( 'NONE',  ( 1.000000000000000000, 0.000000000000000000, 0.000000000000000000 ) ) ;
#10216=CARTESIAN_POINT ( 'NONE',  ( 15.53879320304153744, -3659.720045446122185, 2250.207625598751747 ) ) ;
#10218=LINE ( 'NONE', #17353, #17666 ) ;
#10219=CARTESIAN_POINT ( 'NONE',  ( 136.8842289382999979, -3579.071024516000307, 2250.231635222000023 ) ) ;
#10220=AXIS2_PLACEMENT_3D ( 'NONE', #16851, #7963, #5757 ) ;
#10223=DIRECTION ( 'NONE',  ( 0.000000000000000000, 0.000000000000000000, 1.000000000000000000 ) ) ;
#10224=CARTESIAN_POINT ( 'NONE',  ( 95.25000000000000000, -3543.300000000000182, 2243.277199999999993 ) ) ;
#10226=EDGE_CURVE ( 'NONE', #17073, #3671, #16322, .T. ) ;
#10229=AXIS2_PLACEMENT_3D ( 'NONE', #19468, #6939, #10325 ) ;
#10230=CARTESIAN_POINT ( 'NONE',  ( 141.5168167239393711, -3657.315756010447785, 2247.770112268088724 ) ) ;
#10232=LINE ( 'NONE', #10702, #17075 ) ;
#10234=CIRCLE ( 'NONE', #22939, 2.844799999999961582 ) ;
#10238=SPHERICAL_SURFACE ( 'NONE', #9409, 1.270000000000000018 ) ;
#10240=CARTESIAN_POINT ( 'NONE',  ( 151.4000000000000057, -3694.430000000000291, 2239.039032635400417 ) ) ;
#10241=DIRECTION ( 'NONE',  ( -1.224646799147353207E-16, 1.000000000000000000, 0.000000000000000000 ) ) ;
#10242=VERTEX_POINT ( 'NONE', #10404 ) ;
#10246=DIRECTION ( 'NONE',  ( 0.000000000000000000, -1.000000000000000000, 0.000000000000000000 ) ) ;
#10250=ORIENTED_EDGE ( 'NONE', *, *, #20380, .F. ) ;
#10254=CARTESIAN_POINT ( 'NONE',  ( 10.51600127293235154, -3581.318391123547372, 2248.824551120855176 ) ) ;
#10257=ORIENTED_EDGE ( 'NONE', *, *, #10523, .T. ) ;
#10258=CARTESIAN_POINT ( 'NONE',  ( 101.5999999999999943, -3568.700000000000273, 2259.837999999999738 ) ) ;
#10259=EDGE_CURVE ( 'NONE', #7810, #22994, #15798, .T. ) ;
#10263=DIRECTION ( 'NONE',  ( 0.000000000000000000, 0.000000000000000000, -1.000000000000000000 ) ) ;
#10264=CARTESIAN_POINT ( 'NONE',  ( 10.44172237351025245, -3661.244228531198132, 2250.017997341298724 ) ) ;
#10265=CARTESIAN_POINT ( 'NONE',  ( 147.4602386003344918, -3543.693183278424385, 2260.248803182081247 ) ) ;
#10269=CIRCLE ( 'NONE', #8404, 1.269999999999882334 ) ;
#10270=CARTESIAN_POINT ( 'NONE',  ( 105.2067999999999870, -3670.300000000000182, 2260.600000000000364 ) ) ;
#10272=CARTESIAN_POINT ( 'NONE',  ( 136.9269649396999853, -3660.140004248000423, 2250.236800000000130 ) ) ;
#10273=VECTOR ( 'NONE', #15758, 1000.000000000000000 ) ;
#10274=CARTESIAN_POINT ( 'NONE',  ( 14.57276727744440237, -3657.363329750993216, 2248.017389562041444 ) ) ;
#10275=CARTESIAN_POINT ( 'NONE',  ( 15.54479970632153751, -3579.286029448822319, 2250.212875600666393 ) ) ;
#10276=ORIENTED_EDGE ( 'NONE', *, *, #16148, .F. ) ;
#10277=EDGE_CURVE ( 'NONE', #2318, #5890, #12575, .T. ) ;
#10278=VERTEX_POINT ( 'NONE', #1852 ) ;
#10279=DIRECTION ( 'NONE',  ( -1.000000000000000000, 0.000000000000000000, 0.000000000000000000 ) ) ;
#10280=ORIENTED_EDGE ( 'NONE', *, *, #1779, .T. ) ;
#10283=CARTESIAN_POINT ( 'NONE',  ( 38.10000000000000142, -3644.899999999999636, 2259.837999999999738 ) ) ;
#10287=TOROIDAL_SURFACE ( 'NONE', #196, 3.606799999998999695, 0.7620000000000000107 ) ;
#10288=CARTESIAN_POINT ( 'NONE',  ( 63.50000000000000000, -3594.099999999999909, 2259.837999999999738 ) ) ;
#10289=CIRCLE ( 'NONE', #198, 0.7619999999999294005 ) ;
#10290=CARTESIAN_POINT ( 'NONE',  ( 12.69999999999999929, -3659.504999999999654, 2246.630000000000109 ) ) ;
#10291=EDGE_CURVE ( 'NONE', #825, #4416, #12513, .T. ) ;
#10295=FACE_OUTER_BOUND ( 'NONE', #299, .T. ) ;
#10297=VERTEX_POINT ( 'NONE', #10633 ) ;
#10299=CARTESIAN_POINT ( 'NONE',  ( 10.33664877816801564, -3657.921536567248950, 2249.173046712553969 ) ) ;
#10300=ORIENTED_EDGE ( 'NONE', *, *, #20722, .T. ) ;
#10301=VECTOR ( 'NONE', #163, 1000.000000000000000 ) ;
#10302=EDGE_CURVE ( 'NONE', #5168, #16435, #12146, .T. ) ;
#10303=AXIS2_PLACEMENT_3D ( 'NONE', #6103, #11938, #13229 ) ;
#10304=EDGE_CURVE ( 'NONE', #4174, #14745, #4340, .T. ) ;
#10305=ORIENTED_EDGE ( 'NONE', *, *, #1850, .T. ) ;
#10306=AXIS2_PLACEMENT_3D ( 'NONE', #9583, #11450, #6191 ) ;
#10309=CIRCLE ( 'NONE', #222, 2.844800000000091700 ) ;
#10310=CYLINDRICAL_SURFACE ( 'NONE', #22945, 1.269999999999882334 ) ;
#10312=CARTESIAN_POINT ( 'NONE',  ( 131.7409145027432658, -3695.628299765889096, 2259.750699691084264 ) ) ;
#10313=VECTOR ( 'NONE', #6591, 1000.000000000000000 ) ;
#10316=CARTESIAN_POINT ( 'NONE',  ( 14.53546583297210937, -3581.668498076454853, 2247.847147041044082 ) ) ;
#10317=CARTESIAN_POINT ( 'NONE',  ( 134.1464163013289408, -3658.155994145996374, 2245.352780909838657 ) ) ;
#10318=CIRCLE ( 'NONE', #15192, 3.606799999998994366 ) ;
#10320=VERTEX_POINT ( 'NONE', #1969 ) ;
#10322=LINE ( 'NONE', #1528, #20063 ) ;
#10323=LINE ( 'NONE', #17698, #2072 ) ;
#10324=ORIENTED_EDGE ( 'NONE', *, *, #3117, .F. ) ;
#10325=DIRECTION ( 'NONE',  ( 1.000000000000000000, 0.000000000000000000, 0.000000000000000000 ) ) ;
#10326=ORIENTED_EDGE ( 'NONE', *, *, #4555, .T. ) ;
#10329=AXIS2_PLACEMENT_3D ( 'NONE', #14094, #19477, #19129 ) ;
#10331=CARTESIAN_POINT ( 'NONE',  ( 20.37131517211999920, -3544.241664856000170, 2260.557504477000293 ) ) ;
#10332=CARTESIAN_POINT ( 'NONE',  ( 134.0204252830999962, -3660.140268639000169, 2244.547525601999951 ) ) ;
#10334=DIRECTION ( 'NONE',  ( 0.000000000000000000, 0.000000000000000000, -1.000000000000000000 ) ) ;
#10337=CIRCLE ( 'NONE', #9942, 0.7620000000000126672 ) ;
#10340=CARTESIAN_POINT ( 'NONE',  ( 110.6932000000009992, -3644.899999999999636, 2239.771999999999935 ) ) ;
#10342=CARTESIAN_POINT ( 'NONE',  ( 18.41147883874532099, -3579.724573821228660, 2244.678944975004924 ) ) ;
#10344=CARTESIAN_POINT ( 'NONE',  ( 141.4924172101702595, -3657.295763141121370, 2247.322083679111529 ) ) ;
#10345=CIRCLE ( 'NONE', #5501, 6.477000000000000313 ) ;
#10346=VERTEX_POINT ( 'NONE', #23156 ) ;
#10349=ORIENTED_EDGE ( 'NONE', *, *, #13960, .T. ) ;
#10352=CARTESIAN_POINT ( 'NONE',  ( 15.24000000000000021, -3578.213872745999652, 2255.774000000000342 ) ) ;
#10356=CARTESIAN_POINT ( 'NONE',  ( 151.1299999999999955, -3543.299999999999727, 2259.329999999999927 ) ) ;
#10360=DIRECTION ( 'NONE',  ( -1.000000000000000000, 0.000000000000000000, 0.000000000000000000 ) ) ;
#10361=EDGE_CURVE ( 'NONE', #18918, #10141, #15917, .T. ) ;
#10363=CARTESIAN_POINT ( 'NONE',  ( 67.10679999999999268, -3644.899999999999636, 2260.600000000000364 ) ) ;
#10364=CIRCLE ( 'NONE', #9256, 6.477000000001009283 ) ;
#10365=DIRECTION ( 'NONE',  ( 0.000000000000000000, -1.000000000000000000, 0.000000000000000000 ) ) ;
#10367=LINE ( 'NONE', #12249, #5741 ) ;
#10368=ORIENTED_EDGE ( 'NONE', *, *, #12385, .F. ) ;
#10370=ORIENTED_EDGE ( 'NONE', *, *, #13639, .T. ) ;
#10373=CARTESIAN_POINT ( 'NONE',  ( 10.06869043667276031, -3580.576266314660643, 2249.660797463413928 ) ) ;
#10375=ADVANCED_FACE ( 'NONE', ( #8997 ), #21936, .T. ) ;
#10376=ORIENTED_EDGE ( 'NONE', *, *, #5816, .F. ) ;
#10377=FACE_BOUND ( 'NONE', #2382, .T. ) ;
#10378=TOROIDAL_SURFACE ( 'NONE', #7764, 3.606799999999999784, 0.7620000000000000107 ) ;
#10380=VECTOR ( 'NONE', #4231, 1000.000000000000000 ) ;
#10384=CARTESIAN_POINT ( 'NONE',  ( 11.43159411791845059, -3662.051383365494985, 2249.499054103035633 ) ) ;
#10385=CARTESIAN_POINT ( 'NONE',  ( 15.54478274857000031, -3659.509919104000346, 2250.166342301999521 ) ) ;
#10390=EDGE_CURVE ( 'NONE', #15239, #20703, #21560, .T. ) ;
#10391=CIRCLE ( 'NONE', #4789, 2.844799999999994444 ) ;
#10392=CARTESIAN_POINT ( 'NONE',  ( 136.8551999999999964, -3579.495007806000103, 2250.165025852999861 ) ) ;
#10393=CARTESIAN_POINT ( 'NONE',  ( 15.20174512854452686, -3658.150442273887165, 2249.426080201244986 ) ) ;
#10398=DIRECTION ( 'NONE',  ( -1.000000000000000000, 0.000000000000000000, 0.000000000000000000 ) ) ;
#10404=CARTESIAN_POINT ( 'NONE',  ( 66.34479999999999222, -3594.099999999999909, 2239.771999999999935 ) ) ;
#10406=CARTESIAN_POINT ( 'NONE',  ( 17.31138602735000021, -3576.119152860999748, 2246.630000000000109 ) ) ;
#10407=AXIS2_PLACEMENT_3D ( 'NONE', #21824, #21709, #4015 ) ;
#10414=CARTESIAN_POINT ( 'NONE',  ( 10.29220312187077013, -3657.990044192180449, 2249.254950234671014 ) ) ;
#10416=CARTESIAN_POINT ( 'NONE',  ( 6.984999999999000231, -3579.494999999999891, 2246.630000000000109 ) ) ;
#10418=VERTEX_POINT ( 'NONE', #7026 ) ;
#10420=DIRECTION ( 'NONE',  ( 0.000000000000000000, 0.000000000000000000, 1.000000000000000000 ) ) ;
#10421=EDGE_CURVE ( 'NONE', #6713, #6778, #1336, .T. ) ;
#10423=ADVANCED_FACE ( 'NONE', ( #22887 ), #17623, .T. ) ;
#10424=CARTESIAN_POINT ( 'NONE',  ( 15.54479999999932716, -3579.946214629475435, 2256.063560000000962 ) ) ;
#10427=CARTESIAN_POINT ( 'NONE',  ( 132.0441057205090658, -3694.915156834097161, 2260.510101401284828 ) ) ;
#10430=CARTESIAN_POINT ( 'NONE',  ( 15.54479951278000094, -3579.494996001999880, 2250.165024905999871 ) ) ;
#10433=DIRECTION ( 'NONE',  ( 0.000000000000000000, -1.000000000000000000, 0.000000000000000000 ) ) ;
#10434=FACE_OUTER_BOUND ( 'NONE', #13970, .T. ) ;
#10437=EDGE_CURVE ( 'NONE', #2616, #3620, #19318, .T. ) ;
#10438=EDGE_CURVE ( 'NONE', #6304, #2568, #3212, .T. ) ;
#10439=DIRECTION ( 'NONE',  ( 1.000000000000000000, 0.000000000000000000, 0.000000000000000000 ) ) ;
#10440=VERTEX_POINT ( 'NONE', #15992 ) ;
#10443=CARTESIAN_POINT ( 'NONE',  ( 88.90000000000000568, -3644.899999999999636, 2239.771999999999935 ) ) ;
#10444=VERTEX_POINT ( 'NONE', #10363 ) ;
#10446=VERTEX_POINT ( 'NONE', #8612 ) ;
#10447=CARTESIAN_POINT ( 'NONE',  ( 1.270000000000000018, -3544.570000000000164, 2240.279999999999745 ) ) ;
#10450=CARTESIAN_POINT ( 'NONE',  ( 67.10679999999999268, -3644.899999999999636, 2239.009999999999764 ) ) ;
#10451=EDGE_CURVE ( 'NONE', #8860, #18590, #6555, .T. ) ;
#10456=AXIS2_PLACEMENT_3D ( 'NONE', #7217, #14367, #22783 ) ;
#10458=FACE_OUTER_BOUND ( 'NONE', #3993, .T. ) ;
#10459=CARTESIAN_POINT ( 'NONE',  ( 18.37449373733476321, -3580.174051493370371, 2244.868862703829109 ) ) ;
#10460=AXIS2_PLACEMENT_3D ( 'NONE', #15993, #19623, #3792 ) ;
#10461=CARTESIAN_POINT ( 'NONE',  ( 142.1135160912012054, -3657.999060508418552, 2249.265414016712839 ) ) ;
#10464=VERTEX_POINT ( 'NONE', #13886 ) ;
#10467=DIRECTION ( 'NONE',  ( 0.000000000000000000, 0.000000000000000000, -1.000000000000000000 ) ) ;
#10469=VERTEX_POINT ( 'NONE', #6634 ) ;
#10472=CARTESIAN_POINT ( 'NONE',  ( 4.909282597897117739, -3543.619369473608003, 2260.172357851842207 ) ) ;
#10475=CARTESIAN_POINT ( 'NONE',  ( 101.5999999999999943, -3568.700000000000273, 2259.837999999999738 ) ) ;
#10476=ORIENTED_EDGE ( 'NONE', *, *, #13590, .T. ) ;
#10478=FACE_BOUND ( 'NONE', #14190, .T. ) ;
#10481=EDGE_LOOP ( 'NONE', ( #10180, #6919, #19069, #19244 ) ) ;
#10484=VERTEX_POINT ( 'NONE', #19504 ) ;
#10487=AXIS2_PLACEMENT_3D ( 'NONE', #2669, #11683, #9930 ) ;
#10488=CARTESIAN_POINT ( 'NONE',  ( 10.44280607625477941, -3581.226489564329768, 2248.970834726309477 ) ) ;
#10490=CARTESIAN_POINT ( 'NONE',  ( 151.1299999999999955, -3578.860000000000127, 2251.506800000000112 ) ) ;
#10491=CARTESIAN_POINT ( 'NONE',  ( 137.7873330486999919, -3657.399152860999493, 2246.630000000000109 ) ) ;
#10497=DIRECTION ( 'NONE',  ( 0.000000000000000000, 0.000000000000000000, -1.000000000000000000 ) ) ;
#10498=CARTESIAN_POINT ( 'NONE',  ( 9.855200000000680305, -3579.946214629480892, 2256.063559999999597 ) ) ;
#10500=CARTESIAN_POINT ( 'NONE',  ( 12.44056639605545556, -3662.338708085364033, 2249.197182875595445 ) ) ;
#10507=CARTESIAN_POINT ( 'NONE',  ( 14.81667057278108679, -3657.604317291794359, 2248.681661468295260 ) ) ;
#10508=DIRECTION ( 'NONE',  ( -1.000000000000000000, 0.000000000000000000, 0.000000000000000000 ) ) ;
#10511=DIRECTION ( 'NONE',  ( 0.000000000000000000, 0.000000000000000000, 1.000000000000000000 ) ) ;
#10514=AXIS2_PLACEMENT_3D ( 'NONE', #16024, #12277, #87 ) ;
#10516=CARTESIAN_POINT ( 'NONE',  ( 147.3199999999999932, -3694.430000000000291, 2260.600000000000364 ) ) ;
#10518=AXIS2_PLACEMENT_3D ( 'NONE', #2068, #21973, #312 ) ;
#10519=DIRECTION ( 'NONE',  ( 1.000000000000000000, 0.000000000000000000, 0.000000000000000000 ) ) ;
#10523=EDGE_CURVE ( 'NONE', #12211, #15816, #17051, .T. ) ;
#10528=ORIENTED_EDGE ( 'NONE', *, *, #21537, .F. ) ;
#10532=EDGE_LOOP ( 'NONE', ( #5516, #13641, #12984, #16440, #10055, #6504, #20509, #12871, #9659, #4429 ) ) ;
#10533=LINE ( 'NONE', #12178, #22621 ) ;
#10535=AXIS2_PLACEMENT_3D ( 'NONE', #21467, #10681, #19591 ) ;
#10536=EDGE_LOOP ( 'NONE', ( #6606, #2262, #1387, #6581 ) ) ;
#10537=CARTESIAN_POINT ( 'NONE',  ( 132.0583097651000060, -3694.797466901999996, 2260.545675974999995 ) ) ;
#10545=VERTEX_POINT ( 'NONE', #10127 ) ;
#10548=DIRECTION ( 'NONE',  ( -1.224646799147353207E-16, 1.000000000000000000, 0.000000000000000000 ) ) ;
#10551=DIRECTION ( 'NONE',  ( 0.000000000000000000, 1.000000000000000000, 0.000000000000000000 ) ) ;
#10553=DIRECTION ( 'NONE',  ( -1.000000000000000000, 0.000000000000000000, 0.000000000000000000 ) ) ;
#10555=CARTESIAN_POINT ( 'NONE',  ( 1.270000000000000018, -3694.430000000000291, 2240.279999999999745 ) ) ;
#10556=ORIENTED_EDGE ( 'NONE', *, *, #18733, .T. ) ;
#10557=EDGE_CURVE ( 'NONE', #16518, #12839, #5117, .T. ) ;
#10559=DIRECTION ( 'NONE',  ( 1.000000000000000000, 0.000000000000000000, 0.000000000000000000 ) ) ;
#10561=CARTESIAN_POINT ( 'NONE',  ( 4.836876043304535244, -3695.517456590399433, 2259.991366405333338 ) ) ;
#10563=AXIS2_PLACEMENT_3D ( 'NONE', #3920, #18216, #11068 ) ;
#10569=B_SPLINE_CURVE_WITH_KNOTS ( 'NONE', 3,
 ( #9172, #273, #7415, #605, #4120, #14912 ),
 .UNSPECIFIED., .F., .F.,
 ( 4, 1, 1, 4 ),
 ( 0.000000000000000000, 0.3333333333333000081, 0.6666666666667000474, 1.000000000000000000 ),
 .UNSPECIFIED. ) ;
#10570=AXIS2_PLACEMENT_3D ( 'NONE', #8767, #15915, #23046 ) ;
#10571=VERTEX_POINT ( 'NONE', #12596 ) ;
#10572=AXIS2_PLACEMENT_3D ( 'NONE', #20363, #22114, #14980 ) ;
#10573=DIRECTION ( 'NONE',  ( 0.000000000000000000, -1.000000000000000000, 0.000000000000000000 ) ) ;
#10574=DIRECTION ( 'NONE',  ( 1.000000000000000000, 0.000000000000000000, 0.000000000000000000 ) ) ;
#10579=CARTESIAN_POINT ( 'NONE',  ( 88.90000000000000568, -3594.099999999999909, 2239.009999999999764 ) ) ;
#10582=CIRCLE ( 'NONE', #18796, 2.844800000000091700 ) ;
#10583=CARTESIAN_POINT ( 'NONE',  ( 137.2953324879588592, -3657.985077304744209, 2249.249213757072994 ) ) ;
#10584=ORIENTED_EDGE ( 'NONE', *, *, #20279, .T. ) ;
#10585=CARTESIAN_POINT ( 'NONE',  ( 0.000000000000000000, -3660.140000000000327, 2251.506800000000112 ) ) ;
#10586=CIRCLE ( 'NONE', #3843, 2.844799999999994444 ) ;
#10589=ORIENTED_EDGE ( 'NONE', *, *, #4385, .F. ) ;
#10590=EDGE_LOOP ( 'NONE', ( #16178, #22693 ) ) ;
#10593=CARTESIAN_POINT ( 'NONE',  ( 4.837068669901056772, -3543.482543409432310, 2259.991289493689692 ) ) ;
#10595=LINE ( 'NONE', #10122, #11391 ) ;
#10596=AXIS2_PLACEMENT_3D ( 'NONE', #10290, #17198, #13458 ) ;
#10600=FACE_BOUND ( 'NONE', #4805, .T. ) ;
#10601=DIRECTION ( 'NONE',  ( -1.000000000000000000, 0.000000000000000000, 0.000000000000000000 ) ) ;
#10603=DIRECTION ( 'NONE',  ( 0.000000000000000000, 0.000000000000000000, -1.000000000000000000 ) ) ;
#10604=ORIENTED_EDGE ( 'NONE', *, *, #9456, .F. ) ;
#10608=CARTESIAN_POINT ( 'NONE',  ( 131.6470296322740126, -3543.300000000000182, 2259.515609114269409 ) ) ;
#10609=CARTESIAN_POINT ( 'NONE',  ( 1.270000000000000018, -3544.570000000000164, 2260.600000000000364 ) ) ;
#10611=TOROIDAL_SURFACE ( 'NONE', #16972, 3.606799999999999784, 0.7620000000000000107 ) ;
#10614=DIRECTION ( 'NONE',  ( 1.000000000000000000, 0.000000000000000000, 0.000000000000000000 ) ) ;
#10616=CARTESIAN_POINT ( 'NONE',  ( 12.24081607761725543, -3662.313325058456030, 2249.227689240982272 ) ) ;
#10619=CARTESIAN_POINT ( 'NONE',  ( 147.3321248976842242, -3544.290797603724968, 2260.569570596524045 ) ) ;
#10620=VERTEX_POINT ( 'NONE', #20092 ) ;
#10621=CARTESIAN_POINT ( 'NONE',  ( 124.1552000000010025, -3619.500000000000000, 2239.771999999999935 ) ) ;
#10624=CARTESIAN_POINT ( 'NONE',  ( 15.12638225371395073, -3658.019721843387288, 2249.289087668344564 ) ) ;
#10625=CARTESIAN_POINT ( 'NONE',  ( 136.8684216348929965, -3695.579670241058011, 2255.043798072796562 ) ) ;
#10626=AXIS2_PLACEMENT_3D ( 'NONE', #16853, #7965, #8773 ) ;
#10627=ORIENTED_EDGE ( 'NONE', *, *, #17095, .F. ) ;
#10629=CARTESIAN_POINT ( 'NONE',  ( 145.4149999194000316, -3579.495498070999474, 2244.618783703000190 ) ) ;
#10633=CARTESIAN_POINT ( 'NONE',  ( 137.1599999999999966, -3658.223872745999870, 2255.774000000000342 ) ) ;
#10636=ORIENTED_EDGE ( 'NONE', *, *, #9797, .T. ) ;
#10640=DIRECTION ( 'NONE',  ( 1.000000000000000000, 0.000000000000000000, 0.000000000000000000 ) ) ;
#10642=TOROIDAL_SURFACE ( 'NONE', #17003, 3.606799999999999784, 0.7620000000000000107 ) ;
#10643=CYLINDRICAL_SURFACE ( 'NONE', #3566, 2.844800000000091700 ) ;
#10644=TOROIDAL_SURFACE ( 'NONE', #21494, 3.606799999999999784, 0.7620000000000000107 ) ;
#10645=EDGE_LOOP ( 'NONE', ( #1829, #21920, #11881, #2041 ) ) ;
#10646=CARTESIAN_POINT ( 'NONE',  ( 133.9849999999989905, -3579.494999999999891, 2246.630000000000109 ) ) ;
#10649=DIRECTION ( 'NONE',  ( 1.000000000000000000, 0.000000000000000000, 0.000000000000000000 ) ) ;
#10652=ORIENTED_EDGE ( 'NONE', *, *, #12219, .F. ) ;
#10654=CARTESIAN_POINT ( 'NONE',  ( 136.9179185536690113, -3580.095427802566064, 2249.956228076800926 ) ) ;
#10657=CARTESIAN_POINT ( 'NONE',  ( 54.40679999999999694, -3568.700000000000273, 2259.837999999999738 ) ) ;
#10658=VECTOR ( 'NONE', #21965, 1000.000000000000000 ) ;
#10661=AXIS2_PLACEMENT_3D ( 'NONE', #14235, #2164, #8840 ) ;
#10662=CYLINDRICAL_SURFACE ( 'NONE', #8230, 2.844800000000091700 ) ;
#10663=ADVANCED_FACE ( 'NONE', ( #2276 ), #19745, .F. ) ;
#10666=CARTESIAN_POINT ( 'NONE',  ( 53.64479999999999649, -3568.700000000000273, 2239.771999999999935 ) ) ;
#10667=EDGE_CURVE ( 'NONE', #17851, #12867, #7363, .T. ) ;
#10668=DIRECTION ( 'NONE',  ( 0.000000000000000000, -1.000000000000000000, 0.000000000000000000 ) ) ;
#10669=ORIENTED_EDGE ( 'NONE', *, *, #11943, .F. ) ;
#10670=DIRECTION ( 'NONE',  ( 0.000000000000000000, 1.000000000000000000, 0.000000000000000000 ) ) ;
#10675=DIRECTION ( 'NONE',  ( -0.000000000000000000, 1.000000000000000000, 0.000000000000000000 ) ) ;
#10676=AXIS2_PLACEMENT_3D ( 'NONE', #17611, #1617, #5030 ) ;
#10678=PLANE ( 'NONE',  #4697 ) ;
#10679=CIRCLE ( 'NONE', #16285, 2.844799999998995244 ) ;
#10681=DIRECTION ( 'NONE',  ( 0.000000000000000000, -1.000000000000000000, 0.000000000000000000 ) ) ;
#10682=DIRECTION ( 'NONE',  ( 1.000000000000000000, 0.000000000000000000, 0.000000000000000000 ) ) ;
#10683=VERTEX_POINT ( 'NONE', #16339 ) ;
#10686=CARTESIAN_POINT ( 'NONE',  ( 139.6999999999999886, -3579.494999999999891, 2255.774000000000342 ) ) ;
#10687=CARTESIAN_POINT ( 'NONE',  ( 17.62395365165161110, -3576.592063800514097, 2245.667268896361293 ) ) ;
#10688=DIRECTION ( 'NONE',  ( -1.000000000000000000, -0.000000000000000000, -0.000000000000000000 ) ) ;
#10692=CARTESIAN_POINT ( 'NONE',  ( 15.74707948048999917, -3695.699999999999818, 2254.503999999999905 ) ) ;
#10694=CARTESIAN_POINT ( 'NONE',  ( 1.270000000000000018, -3694.430000000000291, 2240.279999999999745 ) ) ;
#10695=CIRCLE ( 'NONE', #21557, 2.844800000000091700 ) ;
#10698=CARTESIAN_POINT ( 'NONE',  ( 137.6640554538430194, -3657.517572872781784, 2248.495983249934852 ) ) ;
#10700=VECTOR ( 'NONE', #5029, 1000.000000000000000 ) ;
#10702=CARTESIAN_POINT ( 'NONE',  ( 79.04479999999999507, -3670.300000000000182, 2261.869999999999891 ) ) ;
#10703=ORIENTED_EDGE ( 'NONE', *, *, #16948, .T. ) ;
#10704=ORIENTED_EDGE ( 'NONE', *, *, #13438, .T. ) ;
#10706=CARTESIAN_POINT ( 'NONE',  ( 29.00679999999900005, -3670.300000000000182, 2259.837999999999738 ) ) ;
#10708=EDGE_LOOP ( 'NONE', ( #14919, #4794, #223, #14321 ) ) ;
#10709=CARTESIAN_POINT ( 'NONE',  ( 4.934152272631532554, -3543.678681369459810, 2260.234757311799058 ) ) ;
#10714=DIRECTION ( 'NONE',  ( 0.000000000000000000, 0.000000000000000000, -1.000000000000000000 ) ) ;
#10715=ORIENTED_EDGE ( 'NONE', *, *, #22546, .T. ) ;
#10718=FACE_BOUND ( 'NONE', #8803, .T. ) ;
#10720=LINE ( 'NONE', #21731, #18976 ) ;
#10721=AXIS2_PLACEMENT_3D ( 'NONE', #18935, #22558, #13788 ) ;
#10723=EDGE_CURVE ( 'NONE', #14933, #1252, #2167, .T. ) ;
#10725=CARTESIAN_POINT ( 'NONE',  ( 131.8858812533569278, -3543.570688672563847, 2260.113808066775164 ) ) ;
#10729=B_SPLINE_CURVE_WITH_KNOTS ( 'NONE', 3,
 ( #1429, #13856, #19248, #20892 ),
 .UNSPECIFIED., .F., .F.,
 ( 4, 4 ),
 ( 0.000000000000000000, 1.000000000000000000 ),
 .UNSPECIFIED. ) ;
#10731=CARTESIAN_POINT ( 'NONE',  ( 0.000000000000000000, -3695.699999999999818, 2260.600000000000364 ) ) ;
#10732=AXIS2_PLACEMENT_3D ( 'NONE', #9753, #9987, #22515 ) ;
#10733=DIRECTION ( 'NONE',  ( 1.319970543219000025E-14, -1.000000000000000000, -1.319970543219000025E-14 ) ) ;
#10734=CARTESIAN_POINT ( 'NONE',  ( 10.16000000000000014, -3580.776127254000130, 2255.774000000000342 ) ) ;
#10735=CIRCLE ( 'NONE', #6261, 0.7619999999999294005 ) ;
#10738=CARTESIAN_POINT ( 'NONE',  ( 50.79999999999999716, -3568.700000000000273, 2261.869999999999891 ) ) ;
#10744=DIRECTION ( 'NONE',  ( 0.000000000000000000, 0.000000000000000000, -1.000000000000000000 ) ) ;
#10745=CARTESIAN_POINT ( 'NONE',  ( 142.5208746554666561, -3579.068962104421644, 2250.236800009843137 ) ) ;
#10746=CARTESIAN_POINT ( 'NONE',  ( 14.55205406967190029, -3657.345427267659488, 2247.931104812607373 ) ) ;
#10750=CARTESIAN_POINT ( 'NONE',  ( 110.6932000000009992, -3594.099999999999909, 2259.837999999999738 ) ) ;
#10751=ORIENTED_EDGE ( 'NONE', *, *, #5665, .T. ) ;
#10752=CIRCLE ( 'NONE', #4024, 3.606799999999993567 ) ;
#10754=CARTESIAN_POINT ( 'NONE',  ( 10.16000000000000014, -3544.570000000000164, 2255.774000000000342 ) ) ;
#10755=VECTOR ( 'NONE', #19434, 1000.000000000000000 ) ;
#10756=CARTESIAN_POINT ( 'NONE',  ( 67.10679999999999268, -3594.099999999999909, 2239.009999999999764 ) ) ;
#10758=DIRECTION ( 'NONE',  ( 0.000000000000000000, 0.000000000000000000, 1.000000000000000000 ) ) ;
#10759=DIRECTION ( 'NONE',  ( 0.000000000000000000, 0.000000000000000000, -1.000000000000000000 ) ) ;
#10760=CARTESIAN_POINT ( 'NONE',  ( 67.10679999999999268, -3594.099999999999909, 2259.837999999999738 ) ) ;
#10763=ORIENTED_EDGE ( 'NONE', *, *, #21025, .F. ) ;
#10764=DIRECTION ( 'NONE',  ( 0.000000000000000000, -1.000000000000000000, 0.000000000000000000 ) ) ;
#10765=CIRCLE ( 'NONE', #14172, 2.844799999999994444 ) ;
#10769=VERTEX_POINT ( 'NONE', #17864 ) ;
#10770=CYLINDRICAL_SURFACE ( 'NONE', #8565, 2.844800000000091700 ) ;
#10772=ORIENTED_EDGE ( 'NONE', *, *, #9965, .T. ) ;
#10773=CARTESIAN_POINT ( 'NONE',  ( 137.2840491909711602, -3580.996921585915516, 2249.269889241358214 ) ) ;
#10778=AXIS2_PLACEMENT_3D ( 'NONE', #8884, #23152, #7021 ) ;
#10779=CARTESIAN_POINT ( 'NONE',  ( 101.5999999999999943, -3670.300000000000182, 2260.600000000000364 ) ) ;
#10780=CARTESIAN_POINT ( 'NONE',  ( 12.69999999999999929, -3579.494999999999891, 2246.630000000000109 ) ) ;
#10781=CARTESIAN_POINT ( 'NONE',  ( 76.20000000000000284, -3568.700000000000273, 2261.869999999999891 ) ) ;
#10782=CARTESIAN_POINT ( 'NONE',  ( 127.0000000000000000, -3568.700000000000273, 2260.600000000000364 ) ) ;
#10785=DIRECTION ( 'NONE',  ( -1.000000000000000000, 0.000000000000000000, 0.000000000000000000 ) ) ;
#10787=CARTESIAN_POINT ( 'NONE',  ( 135.0886139726999886, -3576.119152860999748, 2246.630000000000109 ) ) ;
#10789=CARTESIAN_POINT ( 'NONE',  ( 88.90000000000000568, -3594.099999999999909, 2259.837999999999738 ) ) ;
#10791=CYLINDRICAL_SURFACE ( 'NONE', #15904, 5.715000000000999947 ) ;
#10797=DIRECTION ( 'NONE',  ( 0.000000000000000000, 0.000000000000000000, 1.000000000000000000 ) ) ;
#10799=CARTESIAN_POINT ( 'NONE',  ( 91.74479999999999791, -3644.899999999999636, 2239.771999999999935 ) ) ;
#10802=CARTESIAN_POINT ( 'NONE',  ( 0.000000000000000000, -3695.699999999999818, 2239.009999999999764 ) ) ;
#10803=FACE_OUTER_BOUND ( 'NONE', #4909, .T. ) ;
#10805=ORIENTED_EDGE ( 'NONE', *, *, #1679, .F. ) ;
#10806=CARTESIAN_POINT ( 'NONE',  ( 59.89320000000000022, -3644.899999999999636, 2239.009999999999764 ) ) ;
#10807=CARTESIAN_POINT ( 'NONE',  ( 10.11266208017212165, -3695.066554905903558, 2255.655544454599294 ) ) ;
#10809=CARTESIAN_POINT ( 'NONE',  ( 18.25358222945826014, -3580.844011449823029, 2245.352786177662892 ) ) ;
#10810=CARTESIAN_POINT ( 'NONE',  ( 137.8353954721896173, -3657.356297066692150, 2247.981376225718122 ) ) ;
#10812=VERTEX_POINT ( 'NONE', #11510 ) ;
#10814=AXIS2_PLACEMENT_3D ( 'NONE', #3787, #10714, #12703 ) ;
#10816=CARTESIAN_POINT ( 'NONE',  ( 137.9361976825551039, -3661.737158740789255, 2249.746205788910174 ) ) ;
#10817=EDGE_CURVE ( 'NONE', #9389, #4126, #20421, .T. ) ;
#10818=ORIENTED_EDGE ( 'NONE', *, *, #14245, .T. ) ;
#10821=CARTESIAN_POINT ( 'NONE',  ( 95.25000000000000000, -3694.430000000000291, 2251.506800000000112 ) ) ;
#10822=ORIENTED_EDGE ( 'NONE', *, *, #17795, .T. ) ;
#10824=CARTESIAN_POINT ( 'NONE',  ( 25.39999999999999858, -3568.700000000000273, 2261.869999999999891 ) ) ;
#10826=CARTESIAN_POINT ( 'NONE',  ( 97.99320000000000164, -3670.300000000000182, 2239.009999999999764 ) ) ;
#10827=DIRECTION ( 'NONE',  ( 0.000000000000000000, 1.000000000000000000, 0.000000000000000000 ) ) ;
#10828=CIRCLE ( 'NONE', #10456, 1.270000000000000018 ) ;
#10829=ORIENTED_EDGE ( 'NONE', *, *, #18163, .T. ) ;
#10831=FACE_OUTER_BOUND ( 'NONE', #18939, .T. ) ;
#10834=AXIS2_PLACEMENT_3D ( 'NONE', #7233, #19648, #14380 ) ;
#10837=DIRECTION ( 'NONE',  ( 0.000000000000000000, 0.000000000000000000, 1.000000000000000000 ) ) ;
#10839=DIRECTION ( 'NONE',  ( -1.000000000000000000, 0.000000000000000000, 0.000000000000000000 ) ) ;
#10841=ORIENTED_EDGE ( 'NONE', *, *, #3476, .T. ) ;
#10842=CARTESIAN_POINT ( 'NONE',  ( 20.82707948048999924, -3695.699999999999818, 2259.329999999999927 ) ) ;
#10846=AXIS2_PLACEMENT_3D ( 'NONE', #13648, #11762, #3095 ) ;
#10847=CARTESIAN_POINT ( 'NONE',  ( 57.14999999999999858, -3694.430000000000291, 2243.277199999999993 ) ) ;
#10848=LINE ( 'NONE', #21636, #18136 ) ;
#10849=ADVANCED_FACE ( 'NONE', ( #15271 ), #22171, .T. ) ;
#10850=EDGE_CURVE ( 'NONE', #15231, #572, #15465, .T. ) ;
#10851=CARTESIAN_POINT ( 'NONE',  ( 147.6115320350049274, -3543.420329759043398, 2259.869779574393760 ) ) ;
#10853=CARTESIAN_POINT ( 'NONE',  ( 95.25000000000000000, -3670.300000000000182, 2247.392000000000280 ) ) ;
#10856=CARTESIAN_POINT ( 'NONE',  ( 79.04479999999999507, -3568.700000000000273, 2259.837999999999738 ) ) ;
#10857=CARTESIAN_POINT ( 'NONE',  ( 142.5315783651326456, -3543.420329758838761, 2255.043798072576010 ) ) ;
#10858=CARTESIAN_POINT ( 'NONE',  ( 35.56000000000000227, -3568.700000000000273, 2247.392000000000280 ) ) ;
#10860=CARTESIAN_POINT ( 'NONE',  ( 7.776600320769382790, -3576.592737331526223, 2245.673273531844188 ) ) ;
#10864=PRODUCT_DEFINITION_FORMATION_WITH_SPECIFIED_SOURCE ( 'ANY', '', #16881, .NOT_KNOWN. ) ;
#10869=DIRECTION ( 'NONE',  ( 0.000000000000000000, -1.000000000000000000, 0.000000000000000000 ) ) ;
#10873=DIRECTION ( 'NONE',  ( 0.000000000000000000, 0.000000000000000000, 1.000000000000000000 ) ) ;
#10874=VERTEX_POINT ( 'NONE', #22473 ) ;
#10876=ORIENTED_EDGE ( 'NONE', *, *, #20889, .T. ) ;
#10878=CARTESIAN_POINT ( 'NONE',  ( 116.8400000000000034, -3670.300000000000182, 2247.392000000000280 ) ) ;
#10881=VERTEX_POINT ( 'NONE', #2916 ) ;
#10885=ORIENTED_EDGE ( 'NONE', *, *, #13682, .F. ) ;
#10886=CARTESIAN_POINT ( 'NONE',  ( 35.56000000000000227, -3670.300000000000182, 2247.392000000000280 ) ) ;
#10887=CARTESIAN_POINT ( 'NONE',  ( 12.69999999999999929, -3659.504999999999654, 2272.030000000000200 ) ) ;
#10889=CARTESIAN_POINT ( 'NONE',  ( 137.7858121020460942, -3581.599504553262250, 2248.159153896805492 ) ) ;
#10895=VERTEX_POINT ( 'NONE', #11397 ) ;
#10900=CARTESIAN_POINT ( 'NONE',  ( 139.2273618935608681, -3576.688940672205717, 2249.230374461885276 ) ) ;
#10902=CIRCLE ( 'NONE', #22860, 3.606799999998994366 ) ;
#10903=CARTESIAN_POINT ( 'NONE',  ( 134.2331161326757751, -3577.829566977919512, 2244.740127772773121 ) ) ;
#10904=CIRCLE ( 'NONE', #14660, 2.844799999998998796 ) ;
#10905=CARTESIAN_POINT ( 'NONE',  ( 101.5999999999999943, -3568.700000000000273, 2259.837999999999738 ) ) ;
#10913=ORIENTED_EDGE ( 'NONE', *, *, #22168, .T. ) ;
#10914=FACE_OUTER_BOUND ( 'NONE', #20847, .T. ) ;
#10916=CARTESIAN_POINT ( 'NONE',  ( 116.8400000000000034, -3568.700000000000273, 2244.547199999999975 ) ) ;
#10920=ORIENTED_EDGE ( 'NONE', *, *, #20232, .F. ) ;
#10921=TOROIDAL_SURFACE ( 'NONE', #13918, 3.606799999999999784, 0.7620000000000000107 ) ;
#10924=ORIENTED_EDGE ( 'NONE', *, *, #16148, .T. ) ;
#10926=CARTESIAN_POINT ( 'NONE',  ( 137.4644108502616291, -3657.744905272460983, 2248.928881783665020 ) ) ;
#10927=EDGE_LOOP ( 'NONE', ( #9698, #7770 ) ) ;
#10929=CARTESIAN_POINT ( 'NONE',  ( 140.8259220789218205, -3662.117874465443492, 2249.436863160725807 ) ) ;
#10931=VERTEX_POINT ( 'NONE', #1148 ) ;
#10932=AXIS2_PLACEMENT_3D ( 'NONE', #22040, #15447, #6005 ) ;
#10934=CIRCLE ( 'NONE', #13190, 2.844799999999994444 ) ;
#10938=CARTESIAN_POINT ( 'NONE',  ( 117.9067999999989951, -3644.899999999999636, 2259.837999999999738 ) ) ;
#10940=CARTESIAN_POINT ( 'NONE',  ( 10.16000000000000014, -3660.786127253999894, 2255.774000000000342 ) ) ;
#10941=ORIENTED_EDGE ( 'NONE', *, *, #7926, .T. ) ;
#10943=EDGE_CURVE ( 'NONE', #14640, #7743, #8863, .T. ) ;
#10944=DIRECTION ( 'NONE',  ( 0.000000000000000000, 0.000000000000000000, 1.000000000000000000 ) ) ;
#10947=CARTESIAN_POINT ( 'NONE',  ( 57.14999999999999858, -3670.300000000000182, 2247.392000000000280 ) ) ;
#10948=CIRCLE ( 'NONE', #831, 0.7619999999999987894 ) ;
#10950=EDGE_CURVE ( 'NONE', #22478, #5090, #14839, .T. ) ;
#10951=ORIENTED_EDGE ( 'NONE', *, *, #1403, .T. ) ;
#10956=DIRECTION ( 'NONE',  ( 1.000000000000000000, 0.000000000000000000, 8.741913579724000206E-14 ) ) ;
#10957=CARTESIAN_POINT ( 'NONE',  ( 7.845716004698516599, -3662.521111503330303, 2245.835192429324707 ) ) ;
#10960=EDGE_CURVE ( 'NONE', #11664, #20457, #16338, .T. ) ;
#10963=AXIS2_PLACEMENT_3D ( 'NONE', #18876, #9966, #1059 ) ;
#10966=CARTESIAN_POINT ( 'NONE',  ( 18.01287425285000410, -3657.399152860999493, 2246.630000000000109 ) ) ;
#10968=CARTESIAN_POINT ( 'NONE',  ( 147.3359700947606825, -3694.748620250581098, 2260.560053407111354 ) ) ;
#10972=VECTOR ( 'NONE', #6834, 1000.000000000000000 ) ;
#10974=FACE_OUTER_BOUND ( 'NONE', #2892, .T. ) ;
#10975=CARTESIAN_POINT ( 'NONE',  ( 136.8581157282275740, -3695.591362401052720, 2255.017974340396904 ) ) ;
#10976=CARTESIAN_POINT ( 'NONE',  ( 7.166763845495746743, -3578.065052041517447, 2244.660461834260786 ) ) ;
#10979=EDGE_CURVE ( 'NONE', #9004, #4452, #699, .T. ) ;
#10983=CIRCLE ( 'NONE', #857, 2.844799999999994444 ) ;
#10990=DIRECTION ( 'NONE',  ( 1.000000000000000000, 0.000000000000000000, 0.000000000000000000 ) ) ;
#10993=ORIENTED_EDGE ( 'NONE', *, *, #12448, .T. ) ;
#10994=DIRECTION ( 'NONE',  ( -1.000000000000000000, 0.000000000000000000, 0.000000000000000000 ) ) ;
#10997=CARTESIAN_POINT ( 'NONE',  ( 8.520528180907378513, -3657.399153627112355, 2246.629997243945581 ) ) ;
#11001=FACE_OUTER_BOUND ( 'NONE', #8920, .T. ) ;
#11002=DIRECTION ( 'NONE',  ( 1.000000000000000000, 0.000000000000000000, 0.000000000000000000 ) ) ;
#11004=CARTESIAN_POINT ( 'NONE',  ( 137.1708602166628737, -3580.797675544396043, 2249.475566895118391 ) ) ;
#11010=DIRECTION ( 'NONE',  ( 0.000000000000000000, 0.000000000000000000, -1.000000000000000000 ) ) ;
#11011=CARTESIAN_POINT ( 'NONE',  ( 47.95519999999999783, -3670.300000000000182, 2239.771999999999935 ) ) ;
#11012=AXIS2_PLACEMENT_3D ( 'NONE', #3142, #22709, #3026 ) ;
#11014=DIRECTION ( 'NONE',  ( 0.000000000000000000, 0.000000000000000000, -1.000000000000000000 ) ) ;
#11015=CARTESIAN_POINT ( 'NONE',  ( 142.2803686719938128, -3578.294778489228975, 2250.180949407634216 ) ) ;
#11017=CARTESIAN_POINT ( 'NONE',  ( 134.8379986833869282, -3576.491331054022794, 2245.816465486069319 ) ) ;
#11018=ORIENTED_EDGE ( 'NONE', *, *, #14722, .F. ) ;
#11019=DIRECTION ( 'NONE',  ( -1.000000000000000000, 0.000000000000000000, 0.000000000000000000 ) ) ;
#11021=DIRECTION ( 'NONE',  ( 0.000000000000000000, 0.000000000000000000, 1.000000000000000000 ) ) ;
#11023=EDGE_CURVE ( 'NONE', #15874, #18712, #21919, .T. ) ;
#11025=EDGE_LOOP ( 'NONE', ( #645, #5783, #8923, #7554, #3201, #11914, #6826, #14668, #15462 ) ) ;
#11026=DIRECTION ( 'NONE',  ( 0.000000000000000000, 0.000000000000000000, 1.000000000000000000 ) ) ;
#11028=AXIS2_PLACEMENT_3D ( 'NONE', #11327, #22327, #14968 ) ;
#11033=CARTESIAN_POINT ( 'NONE',  ( 141.5863318965145652, -3581.624734270543740, 2246.715920429194739 ) ) ;
#11039=CARTESIAN_POINT ( 'NONE',  ( 116.8400000000000034, -3670.300000000000182, 2247.392000000000280 ) ) ;
#11042=CARTESIAN_POINT ( 'NONE',  ( 137.5807515951455855, -3657.607188378255159, 2248.687286021772707 ) ) ;
#11044=ORIENTED_EDGE ( 'NONE', *, *, #8454, .F. ) ;
#11046=CARTESIAN_POINT ( 'NONE',  ( 138.2235839798819370, -3661.937167866388336, 2249.597460511887220 ) ) ;
#11048=ORIENTED_EDGE ( 'NONE', *, *, #19172, .F. ) ;
#11050=EDGE_LOOP ( 'NONE', ( #16804, #16049, #13064, #6383 ) ) ;
#11052=DIRECTION ( 'NONE',  ( 0.000000000000000000, 0.000000000000000000, -1.000000000000000000 ) ) ;
#11054=ORIENTED_EDGE ( 'NONE', *, *, #2834, .F. ) ;
#11057=DIRECTION ( 'NONE',  ( -1.000000000000000000, 0.000000000000000000, 0.000000000000000000 ) ) ;
#11060=CIRCLE ( 'NONE', #10676, 1.269999999999882334 ) ;
#11061=DIRECTION ( 'NONE',  ( 1.000000000000000000, 0.000000000000000000, 0.000000000000000000 ) ) ;
#11064=CARTESIAN_POINT ( 'NONE',  ( 132.0441057203201467, -3544.084843163416281, 2260.510101400297117 ) ) ;
#11065=ORIENTED_EDGE ( 'NONE', *, *, #18440, .T. ) ;
#11068=DIRECTION ( 'NONE',  ( 0.000000000000000000, 0.000000000000000000, 1.000000000000000000 ) ) ;
#11069=EDGE_CURVE ( 'NONE', #5355, #12999, #4647, .T. ) ;
#11070=DIRECTION ( 'NONE',  ( 1.122008997397786234E-13, 0.000000000000000000, -1.000000000000000000 ) ) ;
#11071=AXIS2_PLACEMENT_3D ( 'NONE', #10340, #4830, #17486 ) ;
#11073=EDGE_LOOP ( 'NONE', ( #20209, #22902, #7885, #20709 ) ) ;
#11074=FACE_OUTER_BOUND ( 'NONE', #8193, .T. ) ;
#11076=ADVANCED_FACE ( 'NONE', ( #10295 ), #8550, .F. ) ;
#11077=AXIS2_PLACEMENT_3D ( 'NONE', #11640, #15409, #8259 ) ;
#11082=CYLINDRICAL_SURFACE ( 'NONE', #18883, 2.844800000000091700 ) ;
#11085=ORIENTED_EDGE ( 'NONE', *, *, #1813, .T. ) ;
#11087=FACE_OUTER_BOUND ( 'NONE', #4496, .T. ) ;
#11089=CARTESIAN_POINT ( 'NONE',  ( 147.4095600311624708, -3695.151712726811184, 2260.375808267130651 ) ) ;
#11090=DIRECTION ( 'NONE',  ( -1.000000000000000000, 0.000000000000000000, 0.000000000000000000 ) ) ;
#11091=VECTOR ( 'NONE', #14370, 1000.000000000000000 ) ;
#11093=AXIS2_PLACEMENT_3D ( 'NONE', #6806, #15704, #8447 ) ;
#11094=DIRECTION ( 'NONE',  ( -1.000000000000000000, 0.000000000000000000, 0.000000000000000000 ) ) ;
#11095=CARTESIAN_POINT ( 'NONE',  ( 92.50679999999999836, -3644.899999999999636, 2260.600000000000364 ) ) ;
#11097=DIRECTION ( 'NONE',  ( -1.000000000000000000, 0.000000000000000000, 0.000000000000000000 ) ) ;
#11098=CARTESIAN_POINT ( 'NONE',  ( 7.483768054671388725, -3577.160018264615701, 2245.111000847615287 ) ) ;
#11099=ORIENTED_EDGE ( 'NONE', *, *, #6677, .T. ) ;
#11102=EDGE_CURVE ( 'NONE', #9663, #13850, #4906, .T. ) ;
#11103=CARTESIAN_POINT ( 'NONE',  ( 95.25000000000000000, -3543.299999999999727, 2247.392000000000280 ) ) ;
#11105=DIRECTION ( 'NONE',  ( -1.224646799147353207E-16, 1.000000000000000000, 0.000000000000000000 ) ) ;
#11111=ORIENTED_EDGE ( 'NONE', *, *, #14831, .F. ) ;
#11118=ORIENTED_EDGE ( 'NONE', *, *, #21642, .T. ) ;
#11120=CIRCLE ( 'NONE', #12291, 0.7619999999999987894 ) ;
#11121=AXIS2_PLACEMENT_3D ( 'NONE', #4146, #1075, #18893 ) ;
#11123=CARTESIAN_POINT ( 'NONE',  ( 142.2706172139890839, -3694.866442832754728, 2255.697297438070564 ) ) ;
#11127=CARTESIAN_POINT ( 'NONE',  ( 137.5670226385637704, -3581.377374464106197, 2248.717048606296885 ) ) ;
#11128=EDGE_CURVE ( 'NONE', #5084, #5090, #16301, .T. ) ;
#11132=LINE ( 'NONE', #9372, #5983 ) ;
#11133=DIRECTION ( 'NONE',  ( 1.000000000000000000, 0.000000000000000000, 0.000000000000000000 ) ) ;
#11136=CARTESIAN_POINT ( 'NONE',  ( 140.2422887712748718, -3576.687509671706266, 2249.232688864233751 ) ) ;
#11138=CARTESIAN_POINT ( 'NONE',  ( 134.1907311445957589, -3577.975272958113692, 2244.688205607437339 ) ) ;
#11139=CIRCLE ( 'NONE', #19369, 0.7619999999999294005 ) ;
#11143=CARTESIAN_POINT ( 'NONE',  ( 15.55719817093123680, -3543.392327578681943, 2254.979458604820138 ) ) ;
#11145=ORIENTED_EDGE ( 'NONE', *, *, #11782, .F. ) ;
#11146=EDGE_CURVE ( 'NONE', #21667, #21114, #9929, .T. ) ;
#11147=CARTESIAN_POINT ( 'NONE',  ( 151.1299999999999955, -3694.430000000000291, 2240.279999999999745 ) ) ;
#11149=VERTEX_POINT ( 'NONE', #5260 ) ;
#11152=CARTESIAN_POINT ( 'NONE',  ( 10.66697763051307035, -3577.504112144065402, 2249.893375748385552 ) ) ;
#11154=FACE_BOUND ( 'NONE', #13, .T. ) ;
#11156=ORIENTED_EDGE ( 'NONE', *, *, #10390, .T. ) ;
#11157=CARTESIAN_POINT ( 'NONE',  ( 151.1299999999999955, -3694.430000000000291, 2239.009999999999764 ) ) ;
#11159=AXIS2_PLACEMENT_3D ( 'NONE', #9657, #22291, #16795 ) ;
#11169=CARTESIAN_POINT ( 'NONE',  ( 140.3978084557461443, -3662.263276882629725, 2249.285383685099077 ) ) ;
#11171=VERTEX_POINT ( 'NONE', #2099 ) ;
#11175=ORIENTED_EDGE ( 'NONE', *, *, #6869, .T. ) ;
#11178=EDGE_LOOP ( 'NONE', ( #19098, #19611, #22674, #11336 ) ) ;
#11181=CARTESIAN_POINT ( 'NONE',  ( 7.332978169984068373, -3581.459545042232548, 2246.234697006676925 ) ) ;
#11185=TOROIDAL_SURFACE ( 'NONE', #12674, 3.606799999999999784, 0.7620000000000000107 ) ;
#11187=ORIENTED_EDGE ( 'NONE', *, *, #5868, .F. ) ;
#11188=CARTESIAN_POINT ( 'NONE',  ( 7.052475312426777165, -3660.425490918647938, 2244.547175452708416 ) ) ;
#11189=ORIENTED_EDGE ( 'NONE', *, *, #16997, .F. ) ;
#11190=CARTESIAN_POINT ( 'NONE',  ( 10.16000000000000014, -3695.699999999999818, 2255.774000000000342 ) ) ;
#11192=FACE_OUTER_BOUND ( 'NONE', #17256, .T. ) ;
#11194=ORIENTED_EDGE ( 'NONE', *, *, #9487, .F. ) ;
#11195=CARTESIAN_POINT ( 'NONE',  ( 18.10176712835724189, -3657.638581454599716, 2246.036268407943226 ) ) ;
#11197=CARTESIAN_POINT ( 'NONE',  ( 147.4512129905548932, -3695.282573427842635, 2260.271345400768041 ) ) ;
#11203=DIRECTION ( 'NONE',  ( 0.000000000000000000, 0.000000000000000000, 1.000000000000000000 ) ) ;
#11205=CARTESIAN_POINT ( 'NONE',  ( 7.733373459861585530, -3576.666886843865541, 2245.578275576291617 ) ) ;
#11208=EDGE_CURVE ( 'NONE', #20939, #13646, #18554, .T. ) ;
#11209=VERTEX_POINT ( 'NONE', #9127 ) ;
#11210=CARTESIAN_POINT ( 'NONE',  ( 1.270000000000000018, -3544.570000000000164, 2259.329999999999927 ) ) ;
#11211=AXIS2_PLACEMENT_3D ( 'NONE', #21166, #8743, #14137 ) ;
#11212=EDGE_CURVE ( 'NONE', #1446, #16063, #3842, .T. ) ;
#11214=DIRECTION ( 'NONE',  ( -1.000000000000000000, 0.000000000000000000, 0.000000000000000000 ) ) ;
#11215=ORIENTED_EDGE ( 'NONE', *, *, #4541, .T. ) ;
#11216=CARTESIAN_POINT ( 'NONE',  ( 114.2999999999999972, -3644.899999999999636, 2239.771999999999935 ) ) ;
#11217=ORIENTED_EDGE ( 'NONE', *, *, #12705, .F. ) ;
#11218=CARTESIAN_POINT ( 'NONE',  ( 35.56000000000000227, -3568.700000000000273, 2247.392000000000280 ) ) ;
#11220=CYLINDRICAL_SURFACE ( 'NONE', #13301, 2.844799999998995244 ) ;
#11221=LINE ( 'NONE', #20026, #12952 ) ;
#11225=CIRCLE ( 'NONE', #7849, 4.114799999999974034 ) ;
#11227=VERTEX_POINT ( 'NONE', #331 ) ;
#11228=CARTESIAN_POINT ( 'NONE',  ( 114.2999999999999972, -3594.099999999999909, 2259.837999999999738 ) ) ;
#11229=CARTESIAN_POINT ( 'NONE',  ( 101.5999999999999943, -3619.500000000000000, 2259.837999999999738 ) ) ;
#11231=ORIENTED_EDGE ( 'NONE', *, *, #18822, .F. ) ;
#11232=EDGE_CURVE ( 'NONE', #3301, #4102, #9574, .T. ) ;
#11237=ADVANCED_FACE ( 'NONE', ( #18252 ), #8071, .T. ) ;
#11238=LINE ( 'NONE', #12768, #1481 ) ;
#11239=CARTESIAN_POINT ( 'NONE',  ( 18.24372733278048386, -3660.894223056912324, 2244.648543520397652 ) ) ;
#11240=AXIS2_PLACEMENT_3D ( 'NONE', #17660, #5253, #17779 ) ;
#11241=DIRECTION ( 'NONE',  ( -0.000000000000000000, -1.000000000000000000, -0.000000000000000000 ) ) ;
#11242=CARTESIAN_POINT ( 'NONE',  ( 145.4032257520333360, -3659.928912255530122, 2244.547217120886671 ) ) ;
#11244=CARTESIAN_POINT ( 'NONE',  ( 141.4814987657295546, -3577.276937191656998, 2249.755702771833512 ) ) ;
#11245=ORIENTED_EDGE ( 'NONE', *, *, #827, .F. ) ;
#11247=EDGE_LOOP ( 'NONE', ( #4468, #12813 ) ) ;
#11248=DIRECTION ( 'NONE',  ( -1.000000000000000000, 0.000000000000000000, 0.000000000000000000 ) ) ;
#11250=ORIENTED_EDGE ( 'NONE', *, *, #22157, .T. ) ;
#11251=EDGE_CURVE ( 'NONE', #15997, #9478, #12186, .T. ) ;
#11253=CARTESIAN_POINT ( 'NONE',  ( 15.41071740316960614, -3543.619369471847676, 2255.346357850129607 ) ) ;
#11254=ORIENTED_EDGE ( 'NONE', *, *, #5203, .T. ) ;
#11257=ORIENTED_EDGE ( 'NONE', *, *, #818, .F. ) ;
#11258=CYLINDRICAL_SURFACE ( 'NONE', #1992, 2.844799999999994444 ) ;
#11259=CARTESIAN_POINT ( 'NONE',  ( 12.00521842515822790, -3576.735947014849899, 2249.284512218476721 ) ) ;
#11268=CARTESIAN_POINT ( 'NONE',  ( 9.920099014910965352, -3578.890613119102454, 2250.236564201333294 ) ) ;
#11273=AXIS2_PLACEMENT_3D ( 'NONE', #288, #167, #5443 ) ;
#11274=EDGE_CURVE ( 'NONE', #13472, #8900, #10309, .T. ) ;
#11275=ORIENTED_EDGE ( 'NONE', *, *, #18272, .T. ) ;
#11276=CARTESIAN_POINT ( 'NONE',  ( 140.9395118823992448, -3662.065970330268556, 2249.485863044558755 ) ) ;
#11277=ORIENTED_EDGE ( 'NONE', *, *, #12155, .T. ) ;
#11279=VERTEX_POINT ( 'NONE', #21884 ) ;
#11280=DIRECTION ( 'NONE',  ( 0.000000000000000000, 1.000000000000000000, 0.000000000000000000 ) ) ;
#11284=DIRECTION ( 'NONE',  ( -1.000000000000000000, 0.000000000000000000, 0.000000000000000000 ) ) ;
#11285=B_SPLINE_CURVE_WITH_KNOTS ( 'NONE', 3,
 ( #12825, #11064, #14246, #17981, #16345, #16227, #1817, #21627, #8740, #5226, #10725, #7441, #19511, #17871, #3453, #3686, #18099, #19754, #5690, #14363, #16000, #12604, #5579, #10608, #23129 ),
 .UNSPECIFIED., .F., .F.,
 ( 4, 2, 2, 2, 1, 2, 2, 2, 2, 1, 1, 2, 2, 4 ),
 ( 0.000000000000000000, 0.2500000000093751118, 0.3750000000138445921, 0.4375000000160857438, 0.4687500000172130643, 0.4843750000177767800, 0.5000000000183404403, 0.6250000000212408979, 0.6875000000222054597, 0.7187500000228344010, 0.7343750000228381758, 0.7421875000224096297, 0.7500000000219809726, 1.000000000000000000 ),
 .UNSPECIFIED. ) ;
#11289=CARTESIAN_POINT ( 'NONE',  ( 7.021062793573091376, -3658.864052490032464, 2244.849304824781484 ) ) ;
#11290=FACE_BOUND ( 'NONE', #6247, .T. ) ;
#11291=DIRECTION ( 'NONE',  ( 1.000000000000000000, 0.000000000000000000, 0.000000000000000000 ) ) ;
#11292=DIRECTION ( 'NONE',  ( 0.000000000000000000, 0.000000000000000000, 1.000000000000000000 ) ) ;
#11294=DIRECTION ( 'NONE',  ( -0.000000000000000000, -1.000000000000000000, -0.000000000000000000 ) ) ;
#11295=CARTESIAN_POINT ( 'NONE',  ( 151.4000000000000057, -3578.860000000000127, 2247.392000000000280 ) ) ;
#11296=EDGE_CURVE ( 'NONE', #13554, #16048, #22661, .T. ) ;
#11298=VERTEX_POINT ( 'NONE', #7370 ) ;
#11299=AXIS2_PLACEMENT_3D ( 'NONE', #2612, #11294, #22287 ) ;
#11300=DIRECTION ( 'NONE',  ( -0.7249994335945012525, 0.000000000000000000, 0.6887494619146010688 ) ) ;
#11302=ORIENTED_EDGE ( 'NONE', *, *, #20749, .F. ) ;
#11304=CARTESIAN_POINT ( 'NONE',  ( 18.28735818472415886, -3658.298849057980078, 2245.218321525803276 ) ) ;
#11305=ORIENTED_EDGE ( 'NONE', *, *, #12436, .F. ) ;
#11306=FACE_OUTER_BOUND ( 'NONE', #2036, .T. ) ;
#11307=FACE_OUTER_BOUND ( 'NONE', #21960, .T. ) ;
#11310=ADVANCED_FACE ( 'NONE', ( #19669 ), #11220, .F. ) ;
#11314=AXIS2_PLACEMENT_3D ( 'NONE', #19832, #19724, #3536 ) ;
#11315=CARTESIAN_POINT ( 'NONE',  ( 7.220772795361150465, -3577.865013798726068, 2244.723500464976496 ) ) ;
#11320=DIRECTION ( 'NONE',  ( 0.000000000000000000, 0.000000000000000000, -1.000000000000000000 ) ) ;
#11324=CARTESIAN_POINT ( 'NONE',  ( 134.3616369522012235, -3661.583675183895139, 2244.919872097237203 ) ) ;
#11326=EDGE_LOOP ( 'NONE', ( #2112, #950 ) ) ;
#11327=CARTESIAN_POINT ( 'NONE',  ( 12.69999999999999929, -3579.494999999999891, 2239.771999999999935 ) ) ;
#11328=ORIENTED_EDGE ( 'NONE', *, *, #4229, .F. ) ;
#11330=CARTESIAN_POINT ( 'NONE',  ( 14.02072516994395990, -3662.024738521661675, 2249.522943300878978 ) ) ;
#11332=DIRECTION ( 'NONE',  ( 0.000000000000000000, 0.000000000000000000, -1.000000000000000000 ) ) ;
#11336=ORIENTED_EDGE ( 'NONE', *, *, #8733, .F. ) ;
#11337=DIRECTION ( 'NONE',  ( 0.000000000000000000, 0.000000000000000000, -1.000000000000000000 ) ) ;
#11339=AXIS2_PLACEMENT_3D ( 'NONE', #10782, #17693, #7160 ) ;
#11347=DIRECTION ( 'NONE',  ( -1.000000000000000000, 0.000000000000000000, 0.000000000000000000 ) ) ;
#11348=CARTESIAN_POINT ( 'NONE',  ( 18.03108505668890160, -3661.564694289580530, 2244.928212203581552 ) ) ;
#11352=CARTESIAN_POINT ( 'NONE',  ( 137.2845969902833190, -3577.991942408667001, 2250.101189474289185 ) ) ;
#11353=ORIENTED_EDGE ( 'NONE', *, *, #21324, .F. ) ;
#11354=AXIS2_PLACEMENT_3D ( 'NONE', #19348, #12317, #8914 ) ;
#11357=EDGE_LOOP ( 'NONE', ( #11065, #2626 ) ) ;
#11358=DIRECTION ( 'NONE',  ( 0.000000000000000000, 0.000000000000000000, -1.000000000000000000 ) ) ;
#11360=ADVANCED_FACE ( 'NONE', ( #9006 ), #16155, .T. ) ;
#11364=VERTEX_POINT ( 'NONE', #11554 ) ;
#11366=DIRECTION ( 'NONE',  ( 0.000000000000000000, -1.000000000000000000, 0.000000000000000000 ) ) ;
#11368=CARTESIAN_POINT ( 'NONE',  ( 123.3932000000010021, -3568.700000000000273, 2260.600000000000364 ) ) ;
#11369=CARTESIAN_POINT ( 'NONE',  ( 11.34078435016211017, -3576.994266383828744, 2249.540230614989923 ) ) ;
#11372=CARTESIAN_POINT ( 'NONE',  ( 142.4707046595244435, -3580.142024907966061, 2249.931733785477263 ) ) ;
#11374=CARTESIAN_POINT ( 'NONE',  ( 127.0000000000000000, -3578.860000000000127, 2250.236800000000130 ) ) ;
#11376=AXIS2_PLACEMENT_3D ( 'NONE', #19528, #8633, #10152 ) ;
#11377=FACE_OUTER_BOUND ( 'NONE', #4815, .T. ) ;
#11380=CARTESIAN_POINT ( 'NONE',  ( 20.54577294660182574, -3543.513261182326460, 2260.034604413234774 ) ) ;
#11382=ADVANCED_FACE ( 'NONE', ( #16829 ), #13324, .T. ) ;
#11386=ORIENTED_EDGE ( 'NONE', *, *, #13000, .F. ) ;
#11387=AXIS2_PLACEMENT_3D ( 'NONE', #879, #13197, #18477 ) ;
#11389=EDGE_CURVE ( 'NONE', #9827, #12111, #4260, .T. ) ;
#11390=DIRECTION ( 'NONE',  ( 0.000000000000000000, 0.000000000000000000, -1.000000000000000000 ) ) ;
#11391=VECTOR ( 'NONE', #4970, 999.9999999999998863 ) ;
#11395=ORIENTED_EDGE ( 'NONE', *, *, #18689, .F. ) ;
#11396=CARTESIAN_POINT ( 'NONE',  ( 7.081767858629972601, -3658.457637283788245, 2245.097076080513034 ) ) ;
#11397=CARTESIAN_POINT ( 'NONE',  ( 141.6126669512999854, -3657.399152860999493, 2246.630000000000109 ) ) ;
#11398=DIRECTION ( 'NONE',  ( -1.000000000000000000, 0.000000000000000000, 0.000000000000000000 ) ) ;
#11405=CARTESIAN_POINT ( 'NONE',  ( 142.3916810111898883, -3658.582482988547326, 2249.773500813597366 ) ) ;
#11406=CARTESIAN_POINT ( 'NONE',  ( 116.8400000000000034, -3694.430000000000291, 2244.547199999999975 ) ) ;
#11407=AXIS2_PLACEMENT_3D ( 'NONE', #4473, #955, #16893 ) ;
#11411=ORIENTED_EDGE ( 'NONE', *, *, #15098, .T. ) ;
#11412=CARTESIAN_POINT ( 'NONE',  ( 57.14999999999999858, -3568.700000000000273, 2244.547199999999975 ) ) ;
#11413=CARTESIAN_POINT ( 'NONE',  ( 63.50000000000000000, -3594.099999999999909, 2261.869999999999891 ) ) ;
#11414=ORIENTED_EDGE ( 'NONE', *, *, #4614, .T. ) ;
#11416=CARTESIAN_POINT ( 'NONE',  ( 111.4552000000009997, -3594.099999999999909, 2261.869999999999891 ) ) ;
#11418=CARTESIAN_POINT ( 'NONE',  ( 18.41499991942999870, -3579.495498070999474, 2244.618783703000190 ) ) ;
#11419=TOROIDAL_SURFACE ( 'NONE', #1692, 3.606799999999999784, 0.7620000000000000107 ) ;
#11420=CARTESIAN_POINT ( 'NONE',  ( 59.97894309125000234, -3694.430000000000291, 2175.874270430000252 ) ) ;
#11421=CIRCLE ( 'NONE', #22640, 1.269999999999882334 ) ;
#11425=CARTESIAN_POINT ( 'NONE',  ( 25.39999999999999858, -3670.300000000000182, 2259.837999999999738 ) ) ;
#11428=DIRECTION ( 'NONE',  ( -1.000000000000000000, 0.000000000000000000, 0.000000000000000000 ) ) ;
#11429=ORIENTED_EDGE ( 'NONE', *, *, #12407, .F. ) ;
#11435=AXIS2_PLACEMENT_3D ( 'NONE', #22447, #20477, #4426 ) ;
#11436=ORIENTED_EDGE ( 'NONE', *, *, #2274, .F. ) ;
#11439=CARTESIAN_POINT ( 'NONE',  ( 134.9016472537431639, -3662.609787423094076, 2245.979656123309724 ) ) ;
#11443=ORIENTED_EDGE ( 'NONE', *, *, #11567, .T. ) ;
#11444=CARTESIAN_POINT ( 'NONE',  ( 57.14999999999999858, -3695.699999999999818, 2251.506800000000112 ) ) ;
#11446=CARTESIAN_POINT ( 'NONE',  ( 14.25469908642767969, -3661.887822319809402, 2249.636899428696324 ) ) ;
#11447=CARTESIAN_POINT ( 'NONE',  ( 114.2999999999999972, -3594.099999999999909, 2259.837999999999738 ) ) ;
#11448=ORIENTED_EDGE ( 'NONE', *, *, #3375, .F. ) ;
#11449=VECTOR ( 'NONE', #19014, 1000.000000000000000 ) ;
#11450=DIRECTION ( 'NONE',  ( 0.000000000000000000, 0.000000000000000000, -1.000000000000000000 ) ) ;
#11452=FACE_BOUND ( 'NONE', #4471, .T. ) ;
#11454=DIRECTION ( 'NONE',  ( -1.000000000000000000, 0.000000000000000000, 0.000000000000000000 ) ) ;
#11456=CIRCLE ( 'NONE', #12591, 0.7619999999999987894 ) ;
#11457=ORIENTED_EDGE ( 'NONE', *, *, #22303, .T. ) ;
#11460=ORIENTED_EDGE ( 'NONE', *, *, #17519, .T. ) ;
#11461=CARTESIAN_POINT ( 'NONE',  ( 145.3965142458158653, -3579.956683882830021, 2244.766317903402069 ) ) ;
#11464=CARTESIAN_POINT ( 'NONE',  ( 145.3892580085656050, -3578.952152314642262, 2244.548477537923191 ) ) ;
#11465=DIRECTION ( 'NONE',  ( 0.000000000000000000, 0.000000000000000000, -1.000000000000000000 ) ) ;
#11471=VECTOR ( 'NONE', #9650, 1000.000000000000000 ) ;
#11472=DIRECTION ( 'NONE',  ( 0.000000000000000000, 0.000000000000000000, 1.000000000000000000 ) ) ;
#11473=ORIENTED_EDGE ( 'NONE', *, *, #10361, .T. ) ;
#11474=DIRECTION ( 'NONE',  ( 1.000000000000000000, 0.000000000000000000, -1.224646799147353207E-16 ) ) ;
#11475=VECTOR ( 'NONE', #12748, 1000.000000000000000 ) ;
#11476=CARTESIAN_POINT ( 'NONE',  ( 15.59711802843494510, -3543.356150272710238, 2254.879006054897218 ) ) ;
#11477=AXIS2_PLACEMENT_3D ( 'NONE', #22763, #21256, #8946 ) ;
#11478=ORIENTED_EDGE ( 'NONE', *, *, #6722, .T. ) ;
#11480=AXIS2_PLACEMENT_3D ( 'NONE', #16354, #19996, #3927 ) ;
#11482=CARTESIAN_POINT ( 'NONE',  ( 131.7757523116999891, -3544.570000000000164, 2260.600000000000364 ) ) ;
#11483=ORIENTED_EDGE ( 'NONE', *, *, #3771, .F. ) ;
#11486=CARTESIAN_POINT ( 'NONE',  ( 12.96979589339266781, -3576.650406904108877, 2249.183810675842324 ) ) ;
#11487=CARTESIAN_POINT ( 'NONE',  ( 142.5448000000000093, -3579.495004790000166, 2250.165035197999714 ) ) ;
#11491=VECTOR ( 'NONE', #22375, 1000.000000000000000 ) ;
#11492=EDGE_CURVE ( 'NONE', #724, #3211, #12149, .T. ) ;
#11495=ADVANCED_FACE ( 'NONE', ( #12617 ), #11082, .F. ) ;
#11497=AXIS2_PLACEMENT_3D ( 'NONE', #4238, #4353, #16651 ) ;
#11499=ORIENTED_EDGE ( 'NONE', *, *, #5806, .F. ) ;
#11500=CARTESIAN_POINT ( 'NONE',  ( 142.0922539695508249, -3661.044633775621151, 2250.089196751532199 ) ) ;
#11502=ORIENTED_EDGE ( 'NONE', *, *, #14589, .F. ) ;
#11506=DIRECTION ( 'NONE',  ( 0.000000000000000000, 0.000000000000000000, 1.000000000000000000 ) ) ;
#11507=CARTESIAN_POINT ( 'NONE',  ( 63.50000000000000000, -3594.099999999999909, 2239.009999999999764 ) ) ;
#11509=AXIS2_PLACEMENT_3D ( 'NONE', #15165, #2513, #20328 ) ;
#11510=CARTESIAN_POINT ( 'NONE',  ( 22.55520000000100111, -3670.300000000000182, 2239.771999999999935 ) ) ;
#11512=CARTESIAN_POINT ( 'NONE',  ( 88.90000000000000568, -3594.099999999999909, 2239.009999999999764 ) ) ;
#11517=CARTESIAN_POINT ( 'NONE',  ( 25.39999999999999858, -3619.500000000000000, 2239.771999999999935 ) ) ;
#11519=EDGE_CURVE ( 'NONE', #8062, #17093, #10848, .T. ) ;
#11521=AXIS2_PLACEMENT_3D ( 'NONE', #8363, #8823, #15501 ) ;
#11522=CYLINDRICAL_SURFACE ( 'NONE', #15637, 2.844799999999999773 ) ;
#11524=VERTEX_POINT ( 'NONE', #17761 ) ;
#11527=VERTEX_POINT ( 'NONE', #5591 ) ;
#11528=CARTESIAN_POINT ( 'NONE',  ( 50.79999999999999716, -3619.500000000000000, 2259.837999999999738 ) ) ;
#11537=CIRCLE ( 'NONE', #708, 1.269999999999882334 ) ;
#11538=DIRECTION ( 'NONE',  ( 0.000000000000000000, -1.000000000000000000, 0.000000000000000000 ) ) ;
#11543=DIRECTION ( 'NONE',  ( -1.000000000000000000, 0.000000000000000000, 0.000000000000000000 ) ) ;
#11550=CARTESIAN_POINT ( 'NONE',  ( 135.0294108980580177, -3576.200056266220145, 2246.372099701390198 ) ) ;
#11551=ORIENTED_EDGE ( 'NONE', *, *, #8742, .T. ) ;
#11552=AXIS2_PLACEMENT_3D ( 'NONE', #13183, #16589, #16921 ) ;
#11553=CARTESIAN_POINT ( 'NONE',  ( 25.39999999999999858, -3619.500000000000000, 2259.837999999999738 ) ) ;
#11554=CARTESIAN_POINT ( 'NONE',  ( 19.17699999999999960, -3579.494999999999891, 2239.009999999999764 ) ) ;
#11559=FACE_OUTER_BOUND ( 'NONE', #19955, .T. ) ;
#11561=DIRECTION ( 'NONE',  ( -0.000000000000000000, -1.000000000000000000, -0.000000000000000000 ) ) ;
#11566=CIRCLE ( 'NONE', #11211, 3.606799999998994366 ) ;
#11567=EDGE_CURVE ( 'NONE', #15816, #12211, #8792, .T. ) ;
#11568=ORIENTED_EDGE ( 'NONE', *, *, #16887, .T. ) ;
#11569=CIRCLE ( 'NONE', #22808, 3.606799999999993567 ) ;
#11573=CARTESIAN_POINT ( 'NONE',  ( 18.25703861352807067, -3660.839310627418854, 2244.634233714717993 ) ) ;
#11574=LINE ( 'NONE', #14767, #16353 ) ;
#11575=DIRECTION ( 'NONE',  ( 0.000000000000000000, -1.000000000000000000, 0.000000000000000000 ) ) ;
#11577=CARTESIAN_POINT ( 'NONE',  ( 25.39999999999999858, -3619.500000000000000, 2260.600000000000364 ) ) ;
#11578=ORIENTED_EDGE ( 'NONE', *, *, #7879, .F. ) ;
#11581=EDGE_LOOP ( 'NONE', ( #49, #7910, #14975, #1600 ) ) ;
#11584=CARTESIAN_POINT ( 'NONE',  ( 15.61212078344684251, -3543.344914976206383, 2254.841286577789560 ) ) ;
#11586=ORIENTED_EDGE ( 'NONE', *, *, #16996, .F. ) ;
#11589=ADVANCED_FACE ( 'NONE', ( #19638 ), #3582, .F. ) ;
#11591=LINE ( 'NONE', #20285, #10380 ) ;
#11592=CARTESIAN_POINT ( 'NONE',  ( 11.14473204099212467, -3577.112510630018278, 2249.637028564206048 ) ) ;
#11594=CARTESIAN_POINT ( 'NONE',  ( 141.9827405993179923, -3581.193534353457835, 2249.021006492486322 ) ) ;
#11598=AXIS2_PLACEMENT_3D ( 'NONE', #550, #18356, #18245 ) ;
#11601=CARTESIAN_POINT ( 'NONE',  ( 15.47291618100999955, -3660.140271294999820, 2250.236802488000194 ) ) ;
#11604=ORIENTED_EDGE ( 'NONE', *, *, #20736, .T. ) ;
#11609=FACE_OUTER_BOUND ( 'NONE', #11581, .T. ) ;
#11612=FACE_OUTER_BOUND ( 'NONE', #8832, .T. ) ;
#11615=ORIENTED_EDGE ( 'NONE', *, *, #11677, .T. ) ;
#11616=AXIS2_PLACEMENT_3D ( 'NONE', #17104, #10511, #15353 ) ;
#11617=DIRECTION ( 'NONE',  ( 1.000000000000000000, 0.000000000000000000, 0.000000000000000000 ) ) ;
#11619=FACE_OUTER_BOUND ( 'NONE', #8255, .T. ) ;
#11622=DIRECTION ( 'NONE',  ( -1.000000000000000000, 0.000000000000000000, 0.000000000000000000 ) ) ;
#11623=CARTESIAN_POINT ( 'NONE',  ( 25.39999999999999858, -3670.300000000000182, 2259.837999999999738 ) ) ;
#11627=CARTESIAN_POINT ( 'NONE',  ( 15.54478936534684941, -3659.505023738319323, 2250.165136749944850 ) ) ;
#11629=VERTEX_POINT ( 'NONE', #2734 ) ;
#11630=AXIS2_PLACEMENT_3D ( 'NONE', #20233, #20128, #15075 ) ;
#11632=TOROIDAL_SURFACE ( 'NONE', #22496, 3.606799999999999784, 0.7620000000000000107 ) ;
#11633=CARTESIAN_POINT ( 'NONE',  ( 18.37010631093954061, -3658.790234407184471, 2244.887790217552265 ) ) ;
#11635=ORIENTED_EDGE ( 'NONE', *, *, #21305, .F. ) ;
#11636=ORIENTED_EDGE ( 'NONE', *, *, #18297, .F. ) ;
#11638=ADVANCED_FACE ( 'NONE', ( #16577 ), #10642, .T. ) ;
#11640=CARTESIAN_POINT ( 'NONE',  ( 76.20000000000000284, -3670.300000000000182, 2259.837999999999738 ) ) ;
#11642=DIRECTION ( 'NONE',  ( 0.000000000000000000, 0.000000000000000000, -1.000000000000000000 ) ) ;
#11643=CARTESIAN_POINT ( 'NONE',  ( 142.2400000000000091, -3578.213872745999652, 2255.774000000000342 ) ) ;
#11646=EDGE_LOOP ( 'NONE', ( #3838, #4736, #17535, #8835 ) ) ;
#11650=CARTESIAN_POINT ( 'NONE',  ( 145.2383954616615256, -3658.097948180692583, 2245.407198740987951 ) ) ;
#11651=AXIS2_PLACEMENT_3D ( 'NONE', #20972, #4800, #8667 ) ;
#11656=DIRECTION ( 'NONE',  ( -1.000000000000000000, 0.000000000000000000, 0.000000000000000000 ) ) ;
#11658=CARTESIAN_POINT ( 'NONE',  ( 145.3796772601000100, -3660.139769217999856, 2244.548186305999934 ) ) ;
#11659=ORIENTED_EDGE ( 'NONE', *, *, #8301, .F. ) ;
#11660=LINE ( 'NONE', #2545, #989 ) ;
#11661=TOROIDAL_SURFACE ( 'NONE', #10563, 4.114799999999999791, 1.270000000000000018 ) ;
#11662=CARTESIAN_POINT ( 'NONE',  ( 14.54506894740048750, -3661.670460155497949, 2249.790026138201029 ) ) ;
#11664=VERTEX_POINT ( 'NONE', #6042 ) ;
#11666=DIRECTION ( 'NONE',  ( 1.000000000000000000, 0.000000000000000000, 0.000000000000000000 ) ) ;
#11671=DIRECTION ( 'NONE',  ( -1.000000000000000000, 0.000000000000000000, 0.000000000000000000 ) ) ;
#11675=ORIENTED_EDGE ( 'NONE', *, *, #22609, .T. ) ;
#11677=EDGE_CURVE ( 'NONE', #4249, #14725, #13289, .T. ) ;
#11683=DIRECTION ( 'NONE',  ( 0.000000000000000000, 0.000000000000000000, 1.000000000000000000 ) ) ;
#11684=CYLINDRICAL_SURFACE ( 'NONE', #6981, 2.844799999999999773 ) ;
#11685=B_SPLINE_CURVE_WITH_KNOTS ( 'NONE', 3,
 ( #18681, #17034, #6392, #11418 ),
 .UNSPECIFIED., .F., .F.,
 ( 4, 4 ),
 ( 0.000000000000000000, 1.000000000000000000 ),
 .UNSPECIFIED. ) ;
#11686=AXIS2_PLACEMENT_3D ( 'NONE', #7570, #16473, #21645 ) ;
#11688=CARTESIAN_POINT ( 'NONE',  ( 116.8400000000000034, -3670.300000000000182, 2247.392000000000280 ) ) ;
#11689=VECTOR ( 'NONE', #7917, 1000.000000000000000 ) ;
#11693=EDGE_CURVE ( 'NONE', #17073, #6769, #3527, .T. ) ;
#11695=CIRCLE ( 'NONE', #14716, 2.844800000000001550 ) ;
#11696=CARTESIAN_POINT ( 'NONE',  ( 92.50679999999999836, -3644.899999999999636, 2239.009999999999764 ) ) ;
#11697=ORIENTED_EDGE ( 'NONE', *, *, #12880, .T. ) ;
#11699=DIRECTION ( 'NONE',  ( 1.000000000000000000, 0.000000000000000000, 0.000000000000000000 ) ) ;
#11701=ORIENTED_EDGE ( 'NONE', *, *, #23005, .T. ) ;
#11703=ORIENTED_EDGE ( 'NONE', *, *, #337, .F. ) ;
#11706=VERTEX_POINT ( 'NONE', #15059 ) ;
#11710=EDGE_CURVE ( 'NONE', #17497, #8599, #13260, .T. ) ;
#11711=CARTESIAN_POINT ( 'NONE',  ( 10.28467484152444200, -3577.991815362053330, 2250.101148760488741 ) ) ;
#11714=CARTESIAN_POINT ( 'NONE',  ( 141.7756668328444505, -3581.440556889209802, 2248.589885061244786 ) ) ;
#11718=CARTESIAN_POINT ( 'NONE',  ( 116.8400000000000034, -3670.300000000000182, 2250.236800000000130 ) ) ;
#11719=DIRECTION ( 'NONE',  ( 0.000000000000000000, 0.000000000000000000, -1.000000000000000000 ) ) ;
#11724=ORIENTED_EDGE ( 'NONE', *, *, #10291, .T. ) ;
#11725=FACE_OUTER_BOUND ( 'NONE', #7509, .T. ) ;
#11726=EDGE_CURVE ( 'NONE', #1446, #12415, #12904, .T. ) ;
#11729=ADVANCED_FACE ( 'NONE', ( #18908 ), #10791, .F. ) ;
#11730=ORIENTED_EDGE ( 'NONE', *, *, #14955, .T. ) ;
#11731=ORIENTED_EDGE ( 'NONE', *, *, #9104, .T. ) ;
#11733=ORIENTED_EDGE ( 'NONE', *, *, #13960, .F. ) ;
#11735=B_SPLINE_CURVE_WITH_KNOTS ( 'NONE', 3,
 ( #22648, #19031, #2970, #6624, #11882, #1775, #19585, #14433, #4733, #8919, #10117, #17931, #14202, #10561, #20782, #19708, #17700, #17261, #12431, #17148, #16064, #1647, #3519, #8805 ),
 .UNSPECIFIED., .F., .F.,
 ( 4, 2, 2, 1, 1, 1, 2, 2, 2, 2, 1, 2, 2, 4 ),
 ( 0.000000000000000000, 0.1249999999999866773, 0.1875000000002543799, 0.2187499999999581168, 0.2343749999998102629, 0.2421874999995853595, 0.2460937499996319056, 0.2499999999996784517, 0.3749999999999907296, 0.4375000000003181899, 0.4687500000004818923, 0.4843750000003246847, 0.5000000000001674216, 1.000000000000000000 ),
 .UNSPECIFIED. ) ;
#11738=CARTESIAN_POINT ( 'NONE',  ( 7.259347590869622557, -3657.755355890642932, 2245.840513791162266 ) ) ;
#11740=DIRECTION ( 'NONE',  ( -1.000000000000000000, 0.000000000000000000, 0.000000000000000000 ) ) ;
#11743=CARTESIAN_POINT ( 'NONE',  ( 101.5999999999999943, -3568.700000000000273, 2239.771999999999935 ) ) ;
#11744=VERTEX_POINT ( 'NONE', #19146 ) ;
#11747=CARTESIAN_POINT ( 'NONE',  ( 141.9904798895065312, -3657.817844140880425, 2249.035397113753334 ) ) ;
#11751=EDGE_LOOP ( 'NONE', ( #22483, #18776, #18304, #4061, #4860 ) ) ;
#11754=FACE_OUTER_BOUND ( 'NONE', #19274, .T. ) ;
#11755=EDGE_LOOP ( 'NONE', ( #7381, #13421, #23032, #21501 ) ) ;
#11756=ORIENTED_EDGE ( 'NONE', *, *, #3482, .T. ) ;
#11761=ORIENTED_EDGE ( 'NONE', *, *, #3952, .F. ) ;
#11762=DIRECTION ( 'NONE',  ( 0.000000000000000000, 0.000000000000000000, 1.000000000000000000 ) ) ;
#11763=FACE_OUTER_BOUND ( 'NONE', #11073, .T. ) ;
#11765=CIRCLE ( 'NONE', #7660, 2.844800000000091700 ) ;
#11771=EDGE_CURVE ( 'NONE', #18027, #11171, #5810, .T. ) ;
#11772=EDGE_LOOP ( 'NONE', ( #5729, #11054, #10751, #19149 ) ) ;
#11775=DIRECTION ( 'NONE',  ( 0.000000000000000000, -1.000000000000000000, 0.000000000000000000 ) ) ;
#11779=ORIENTED_EDGE ( 'NONE', *, *, #17422, .F. ) ;
#11780=ORIENTED_EDGE ( 'NONE', *, *, #2566, .T. ) ;
#11781=DIRECTION ( 'NONE',  ( 0.000000000000000000, 0.000000000000000000, 1.000000000000000000 ) ) ;
#11782=EDGE_CURVE ( 'NONE', #13993, #16307, #11735, .T. ) ;
#11785=CARTESIAN_POINT ( 'NONE',  ( 144.3705891021011780, -3662.799943733657074, 2246.372099701068237 ) ) ;
#11787=DIRECTION ( 'NONE',  ( 1.000000000000000000, 0.000000000000000000, 0.000000000000000000 ) ) ;
#11789=CARTESIAN_POINT ( 'NONE',  ( 14.86903996120028992, -3661.345726835937057, 2249.968664091575192 ) ) ;
#11793=ORIENTED_EDGE ( 'NONE', *, *, #4614, .F. ) ;
#11794=ADVANCED_FACE ( 'NONE', ( #4613 ), #7288, .T. ) ;
#11795=CARTESIAN_POINT ( 'NONE',  ( 141.6126318482000102, -3581.600863517000107, 2246.630000000000109 ) ) ;
#11797=CARTESIAN_POINT ( 'NONE',  ( 133.9850000019999925, -3579.284332437912781, 2244.570779506149393 ) ) ;
#11799=CARTESIAN_POINT ( 'NONE',  ( 114.2999999999999972, -3644.899999999999636, 2259.837999999999738 ) ) ;
#11803=AXIS2_PLACEMENT_3D ( 'NONE', #18601, #1124, #8057 ) ;
#11804=ORIENTED_EDGE ( 'NONE', *, *, #12816, .T. ) ;
#11806=TOROIDAL_SURFACE ( 'NONE', #21558, 6.477000000000000313, 0.7620000000000000107 ) ;
#11818=ORIENTED_EDGE ( 'NONE', *, *, #5577, .F. ) ;
#11822=TOROIDAL_SURFACE ( 'NONE', #1731, 3.606799999998999695, 0.7620000000000000107 ) ;
#11825=CARTESIAN_POINT ( 'NONE',  ( 10.66409421166686045, -3657.517533168687805, 2248.495888785344960 ) ) ;
#11826=AXIS2_PLACEMENT_3D ( 'NONE', #9306, #7428, #7195 ) ;
#11830=CARTESIAN_POINT ( 'NONE',  ( 134.3229528927292336, -3581.431939766277537, 2246.174326570847370 ) ) ;
#11833=AXIS2_PLACEMENT_3D ( 'NONE', #16937, #11781, #1352 ) ;
#11836=CARTESIAN_POINT ( 'NONE',  ( 47.19319999999999737, -3568.700000000000273, 2239.771999999999935 ) ) ;
#11838=VECTOR ( 'NONE', #23137, 1000.000000000000000 ) ;
#11839=CARTESIAN_POINT ( 'NONE',  ( 142.1866385280289933, -3580.879155498138061, 2249.398837230915888 ) ) ;
#11841=CARTESIAN_POINT ( 'NONE',  ( 131.8826821606740225, -3695.435514547667026, 2260.105825662819370 ) ) ;
#11843=DIRECTION ( 'NONE',  ( 0.6887494619146551367, 0.000000000000000000, -0.7249994335944497381 ) ) ;
#11844=CARTESIAN_POINT ( 'NONE',  ( 14.78644416229590242, -3581.429898611652334, 2248.616548156125646 ) ) ;
#11845=CARTESIAN_POINT ( 'NONE',  ( 134.2737407819179793, -3657.711383914624548, 2245.910523936043319 ) ) ;
#11847=ORIENTED_EDGE ( 'NONE', *, *, #18090, .T. ) ;
#11849=CARTESIAN_POINT ( 'NONE',  ( 142.1146155143981105, -3661.009309353270964, 2250.100788259126602 ) ) ;
#11851=EDGE_CURVE ( 'NONE', #749, #8027, #12522, .T. ) ;
#11855=CARTESIAN_POINT ( 'NONE',  ( 25.39999999999999858, -3619.500000000000000, 2239.771999999999935 ) ) ;
#11856=DIRECTION ( 'NONE',  ( -1.000000000000000000, 0.000000000000000000, 0.000000000000000000 ) ) ;
#11859=CARTESIAN_POINT ( 'NONE',  ( 63.50000000000000000, -3644.899999999999636, 2259.837999999999738 ) ) ;
#11861=EDGE_CURVE ( 'NONE', #14115, #17865, #8406, .T. ) ;
#11867=CARTESIAN_POINT ( 'NONE',  ( 95.25000000000000000, -3544.570000000000164, 2247.392000000000280 ) ) ;
#11870=ADVANCED_FACE ( 'NONE', ( #12780 ), #20164, .F. ) ;
#11871=CIRCLE ( 'NONE', #7039, 2.844799999998998796 ) ;
#11872=FACE_OUTER_BOUND ( 'NONE', #12587, .T. ) ;
#11874=DIRECTION ( 'NONE',  ( 1.000000000000000000, 0.000000000000000000, 0.000000000000000000 ) ) ;
#11875=CARTESIAN_POINT ( 'NONE',  ( 142.0975596452481113, -3657.973835563076136, 2249.236080756626507 ) ) ;
#11877=VERTEX_POINT ( 'NONE', #362 ) ;
#11878=CARTESIAN_POINT ( 'NONE',  ( 137.1440651153584156, -3544.251379750218803, 2255.734039348538772 ) ) ;
#11881=ORIENTED_EDGE ( 'NONE', *, *, #13941, .T. ) ;
#11882=CARTESIAN_POINT ( 'NONE',  ( 4.722483775760038860, -3695.643849723204767, 2259.705165060028776 ) ) ;
#11885=AXIS2_PLACEMENT_3D ( 'NONE', #22151, #6238, #6123 ) ;
#11888=B_SPLINE_CURVE_WITH_KNOTS ( 'NONE', 3,
 ( #15236, #9495, #16633, #591 ),
 .UNSPECIFIED., .F., .F.,
 ( 4, 4 ),
 ( 0.000000000000000000, 1.000000000000000000 ),
 .UNSPECIFIED. ) ;
#11895=CARTESIAN_POINT ( 'NONE',  ( 35.56000000000000227, -3670.300000000000182, 2247.392000000000280 ) ) ;
#11897=CARTESIAN_POINT ( 'NONE',  ( 20.54573065161225287, -3695.486738824718486, 2260.034587513629049 ) ) ;
#11898=ORIENTED_EDGE ( 'NONE', *, *, #20562, .F. ) ;
#11901=VERTEX_POINT ( 'NONE', #20607 ) ;
#11903=CARTESIAN_POINT ( 'NONE',  ( 10.22015228523534702, -3580.889289654939603, 2249.386560310950699 ) ) ;
#11905=ORIENTED_EDGE ( 'NONE', *, *, #9831, .T. ) ;
#11907=FACE_BOUND ( 'NONE', #12619, .T. ) ;
#11908=DIRECTION ( 'NONE',  ( 1.000000000000000000, 0.000000000000000000, 0.000000000000000000 ) ) ;
#11910=DIRECTION ( 'NONE',  ( -1.000000000000000000, 0.000000000000000000, 0.000000000000000000 ) ) ;
#11913=DIRECTION ( 'NONE',  ( -1.000000000000000000, 0.000000000000000000, 0.000000000000000000 ) ) ;
#11914=ORIENTED_EDGE ( 'NONE', *, *, #4937, .F. ) ;
#11915=LINE ( 'NONE', #1244, #6152 ) ;
#11917=EDGE_CURVE ( 'NONE', #19732, #4416, #2921, .T. ) ;
#11918=DIRECTION ( 'NONE',  ( -1.000000000000000000, 0.000000000000000000, 0.000000000000000000 ) ) ;
#11921=ORIENTED_EDGE ( 'NONE', *, *, #16681, .T. ) ;
#11923=EDGE_CURVE ( 'NONE', #3271, #15794, #5434, .T. ) ;
#11924=EDGE_LOOP ( 'NONE', ( #5852, #3768, #13549, #7055 ) ) ;
#11926=ORIENTED_EDGE ( 'NONE', *, *, #15885, .T. ) ;
#11928=CARTESIAN_POINT ( 'NONE',  ( 97.99320000000000164, -3619.500000000000000, 2239.009999999999764 ) ) ;
#11929=LINE ( 'NONE', #3021, #1125 ) ;
#11930=DIRECTION ( 'NONE',  ( -1.000000000000000000, 0.000000000000000000, 0.000000000000000000 ) ) ;
#11931=AXIS2_PLACEMENT_3D ( 'NONE', #15093, #7947, #4195 ) ;
#11933=CARTESIAN_POINT ( 'NONE',  ( 88.90000000000000568, -3644.899999999999636, 2239.771999999999935 ) ) ;
#11938=DIRECTION ( 'NONE',  ( -1.000000000000000000, 0.000000000000000000, 0.000000000000000000 ) ) ;
#11939=ORIENTED_EDGE ( 'NONE', *, *, #7426, .T. ) ;
#11940=CARTESIAN_POINT ( 'NONE',  ( 18.40310581996000039, -3659.924389696708658, 2244.547177115724480 ) ) ;
#11941=CARTESIAN_POINT ( 'NONE',  ( 10.87600349139550993, -3657.321675656191928, 2247.788763825722071 ) ) ;
#11943=EDGE_CURVE ( 'NONE', #5168, #17725, #5059, .T. ) ;
#11945=CARTESIAN_POINT ( 'NONE',  ( 22.55520000000100111, -3568.700000000000273, 2261.869999999999891 ) ) ;
#11946=EDGE_CURVE ( 'NONE', #16187, #3108, #6150, .T. ) ;
#11948=ORIENTED_EDGE ( 'NONE', *, *, #15747, .T. ) ;
#11953=ORIENTED_EDGE ( 'NONE', *, *, #2226, .T. ) ;
#11954=CARTESIAN_POINT ( 'NONE',  ( 131.7444118345384823, -3695.625189109597613, 2259.759456293023959 ) ) ;
#11957=CARTESIAN_POINT ( 'NONE',  ( 15.31352823294669996, -3580.622497904614647, 2249.627690351728688 ) ) ;
#11959=CARTESIAN_POINT ( 'NONE',  ( 134.0820746908595140, -3658.455984731507215, 2245.098290645206362 ) ) ;
#11962=VERTEX_POINT ( 'NONE', #3032 ) ;
#11964=CARTESIAN_POINT ( 'NONE',  ( 15.61261851050921479, -3695.655085023901847, 2254.841485307673338 ) ) ;
#11966=EDGE_LOOP ( 'NONE', ( #5966, #659, #11697, #6743, #17117, #6825, #13568, #11578 ) ) ;
#11967=CARTESIAN_POINT ( 'NONE',  ( 63.50000000000000000, -3594.099999999999909, 2259.837999999999738 ) ) ;
#11969=ORIENTED_EDGE ( 'NONE', *, *, #12407, .T. ) ;
#11970=ORIENTED_EDGE ( 'NONE', *, *, #5162, .F. ) ;
#11971=DIRECTION ( 'NONE',  ( -1.000000000000000000, 0.000000000000000000, 0.000000000000000000 ) ) ;
#11973=CIRCLE ( 'NONE', #22089, 2.844799999999994444 ) ;
#11976=FACE_BOUND ( 'NONE', #9714, .T. ) ;
#11981=LINE ( 'NONE', #20769, #4734 ) ;
#11984=EDGE_CURVE ( 'NONE', #21686, #15874, #20393, .T. ) ;
#11985=PLANE ( 'NONE',  #8468 ) ;
#11988=CARTESIAN_POINT ( 'NONE',  ( 142.2710730780391941, -3658.284631445515060, 2249.551220062097855 ) ) ;
#11990=CARTESIAN_POINT ( 'NONE',  ( 136.8326944598556736, -3543.381058768859020, 2254.954196763766959 ) ) ;
#11997=CARTESIAN_POINT ( 'NONE',  ( 116.8400000000000034, -3544.570000000000164, 2244.547199999999975 ) ) ;
#12000=CARTESIAN_POINT ( 'NONE',  ( 4.762801830632181321, -3543.392327580375422, 2259.805458609068864 ) ) ;
#12001=CARTESIAN_POINT ( 'NONE',  ( 88.90000000000000568, -3644.899999999999636, 2239.009999999999764 ) ) ;
#12002=CARTESIAN_POINT ( 'NONE',  ( 146.1769999999999925, -3659.504999999999654, 2239.771999999999935 ) ) ;
#12003=EDGE_LOOP ( 'NONE', ( #6083, #2988 ) ) ;
#12006=CARTESIAN_POINT ( 'NONE',  ( 139.6999999999999886, -3659.504999999999654, 2255.774000000000342 ) ) ;
#12008=CARTESIAN_POINT ( 'NONE',  ( 18.34748010882359992, -3578.572769233774579, 2244.547227114076122 ) ) ;
#12010=EDGE_LOOP ( 'NONE', ( #13267, #18219, #7739, #6973 ) ) ;
#12013=EDGE_CURVE ( 'NONE', #12638, #9982, #16976, .T. ) ;
#12014=ORIENTED_EDGE ( 'NONE', *, *, #22986, .T. ) ;
#12018=CARTESIAN_POINT ( 'NONE',  ( 10.64300821491179683, -3581.461259321691614, 2248.549161679750796 ) ) ;
#12023=FACE_OUTER_BOUND ( 'NONE', #7838, .T. ) ;
#12024=CIRCLE ( 'NONE', #13885, 3.606800000000000228 ) ;
#12025=DIRECTION ( 'NONE',  ( 0.000000000000000000, 0.000000000000000000, -1.000000000000000000 ) ) ;
#12026=CARTESIAN_POINT ( 'NONE',  ( 144.9086821617023588, -3661.856755788642204, 2245.123591690442936 ) ) ;
#12028=ADVANCED_FACE ( 'NONE', ( #4445 ), #12169, .T. ) ;
#12029=CARTESIAN_POINT ( 'NONE',  ( 12.96232367102921579, -3662.340837267252027, 2249.194767252861766 ) ) ;
#12030=CARTESIAN_POINT ( 'NONE',  ( 147.4569745407331141, -3543.701815209187771, 2260.256976450936236 ) ) ;
#12031=ORIENTED_EDGE ( 'NONE', *, *, #6354, .F. ) ;
#12032=CARTESIAN_POINT ( 'NONE',  ( 142.5447999999993272, -3579.946214629432234, 2256.063560000000962 ) ) ;
#12035=CARTESIAN_POINT ( 'NONE',  ( 15.05256792404641075, -3657.905201311359178, 2249.153143157146587 ) ) ;
#12037=ORIENTED_EDGE ( 'NONE', *, *, #3248, .T. ) ;
#12041=ORIENTED_EDGE ( 'NONE', *, *, #16011, .F. ) ;
#12043=FACE_OUTER_BOUND ( 'NONE', #23079, .T. ) ;
#12044=CARTESIAN_POINT ( 'NONE',  ( 15.24000000000000021, -3695.699999999999818, 2255.774000000000342 ) ) ;
#12048=DIRECTION ( 'NONE',  ( 0.000000000000000000, 0.000000000000000000, 1.000000000000000000 ) ) ;
#12054=CIRCLE ( 'NONE', #6815, 3.606799999998994366 ) ;
#12058=CARTESIAN_POINT ( 'NONE',  ( 10.11254281055728299, -3658.322299598116388, 2249.580929887502862 ) ) ;
#12060=ORIENTED_EDGE ( 'NONE', *, *, #6221, .T. ) ;
#12061=DIRECTION ( 'NONE',  ( -1.000000000000000000, 0.000000000000000000, 0.000000000000000000 ) ) ;
#12068=CARTESIAN_POINT ( 'NONE',  ( 132.0226525136210967, -3695.032413813642052, 2260.455666005582316 ) ) ;
#12072=CARTESIAN_POINT ( 'NONE',  ( 21.79320000000099711, -3619.500000000000000, 2259.837999999999738 ) ) ;
#12073=CARTESIAN_POINT ( 'NONE',  ( 14.48688036290512038, -3581.708692406665250, 2247.466127284272716 ) ) ;
#12074=CARTESIAN_POINT ( 'NONE',  ( 134.2236363864670636, -3657.869847840709099, 2245.675467034049689 ) ) ;
#12075=EDGE_CURVE ( 'NONE', #9663, #16380, #13588, .T. ) ;
#12077=DIRECTION ( 'NONE',  ( 0.000000000000000000, 0.000000000000000000, -1.000000000000000000 ) ) ;
#12086=TOROIDAL_SURFACE ( 'NONE', #14344, 4.114799999999999791, 1.270000000000000018 ) ;
#12089=EDGE_CURVE ( 'NONE', #18860, #17851, #10289, .T. ) ;
#12090=CARTESIAN_POINT ( 'NONE',  ( 20.34169023495000062, -3544.202533098000458, 2260.545675974999995 ) ) ;
#12091=CARTESIAN_POINT ( 'NONE',  ( 134.0147555151665699, -3660.087502428663811, 2244.547653756476848 ) ) ;
#12093=FACE_BOUND ( 'NONE', #8123, .T. ) ;
#12094=CARTESIAN_POINT ( 'NONE',  ( 15.54478274856999853, -3659.614687031725680, 2250.189939678317842 ) ) ;
#12095=DIRECTION ( 'NONE',  ( 1.000000000000000000, 0.000000000000000000, 0.000000000000000000 ) ) ;
#12097=DIRECTION ( 'NONE',  ( 1.000000000000000000, 0.000000000000000000, 0.000000000000000000 ) ) ;
#12098=VECTOR ( 'NONE', #18502, 1000.000000000000000 ) ;
#12101=AXIS2_PLACEMENT_3D ( 'NONE', #10750, #4568, #17895 ) ;
#12103=CARTESIAN_POINT ( 'NONE',  ( 136.8552000000009912, -3579.494999999999891, 2272.030000000000200 ) ) ;
#12104=DIRECTION ( 'NONE',  ( -1.000000000000000000, 0.000000000000000000, 0.000000000000000000 ) ) ;
#12106=CARTESIAN_POINT ( 'NONE',  ( 141.7270126280175475, -3657.507999012949767, 2248.476214850042652 ) ) ;
#12108=EDGE_CURVE ( 'NONE', #13681, #14824, #8663, .T. ) ;
#12110=VERTEX_POINT ( 'NONE', #19559 ) ;
#12111=VERTEX_POINT ( 'NONE', #13939 ) ;
#12117=FACE_OUTER_BOUND ( 'NONE', #15468, .T. ) ;
#12118=CARTESIAN_POINT ( 'NONE',  ( 15.24000000000000021, -3580.776127254000130, 2255.774000000000342 ) ) ;
#12121=DIRECTION ( 'NONE',  ( 0.000000000000000000, 1.000000000000000000, 0.000000000000000000 ) ) ;
#12126=ORIENTED_EDGE ( 'NONE', *, *, #10277, .T. ) ;
#12129=TOROIDAL_SURFACE ( 'NONE', #17349, 4.114799999999999791, 1.270000000000000018 ) ;
#12130=CARTESIAN_POINT ( 'NONE',  ( 10.58260127282864538, -3581.394912766336802, 2248.683245035067102 ) ) ;
#12131=EDGE_LOOP ( 'NONE', ( #14346, #21823 ) ) ;
#12134=B_SPLINE_CURVE_WITH_KNOTS ( 'NONE', 3,
 ( #22846, #3054, #13846, #11964, #19114, #14079, #15608, #3291, #19234, #15, #17697, #19580, #13732, #14199, #17466, #22738, #15950, #5179, #8685, #12319, #7056, #6819, #10203, #17340 ),
 .UNSPECIFIED., .F., .F.,
 ( 4, 2, 2, 1, 1, 1, 2, 2, 2, 2, 1, 2, 2, 4 ),
 ( 0.000000000000000000, 0.1250000000064511452, 0.1875000000096775921, 0.2187500000117214016, 0.2343750000127438893, 0.2421875000132545364, 0.2460937500135104705, 0.2500000000137663769, 0.3750000000113288823, 0.4375000000103546061, 0.4687500000103158038, 0.4843750000103104192, 0.5000000000103050901, 1.000000000000000000 ),
 .UNSPECIFIED. ) ;
#12140=CARTESIAN_POINT ( 'NONE',  ( 11.42511155983525839, -3662.048141298665541, 2249.501989319668610 ) ) ;
#12142=ADVANCED_FACE ( 'NONE', ( #15809 ), #14250, .T. ) ;
#12144=ORIENTED_EDGE ( 'NONE', *, *, #11146, .T. ) ;
#12145=EDGE_CURVE ( 'NONE', #12156, #13472, #17794, .T. ) ;
#12146=B_SPLINE_CURVE_WITH_KNOTS ( 'NONE', 3,
 ( #16034, #12399, #5499, #7247 ),
 .UNSPECIFIED., .F., .F.,
 ( 4, 4 ),
 ( 0.000000000000000000, 1.000000000000000000 ),
 .UNSPECIFIED. ) ;
#12147=DIRECTION ( 'NONE',  ( 0.000000000000000000, 0.000000000000000000, 1.000000000000000000 ) ) ;
#12149=CIRCLE ( 'NONE', #14784, 3.606799999999993567 ) ;
#12151=VECTOR ( 'NONE', #17736, 1000.000000000000000 ) ;
#12152=CARTESIAN_POINT ( 'NONE',  ( 15.26350286127714284, -3658.268776985493332, 2249.537495782451060 ) ) ;
#12153=CARTESIAN_POINT ( 'NONE',  ( 40.94480000000000075, -3644.899999999999636, 2261.869999999999891 ) ) ;
#12154=EDGE_LOOP ( 'NONE', ( #687, #8625, #18730, #13321 ) ) ;
#12155=EDGE_CURVE ( 'NONE', #16634, #17242, #10533, .T. ) ;
#12156=VERTEX_POINT ( 'NONE', #14288 ) ;
#12158=EDGE_LOOP ( 'NONE', ( #14662, #6505, #20556, #15520 ) ) ;
#12159=DIRECTION ( 'NONE',  ( -1.000000000000000000, 0.000000000000000000, 0.000000000000000000 ) ) ;
#12161=EDGE_CURVE ( 'NONE', #4345, #5555, #5386, .T. ) ;
#12162=FACE_OUTER_BOUND ( 'NONE', #4277, .T. ) ;
#12165=DIRECTION ( 'NONE',  ( 0.000000000000000000, 0.000000000000000000, 1.000000000000000000 ) ) ;
#12168=DIRECTION ( 'NONE',  ( 0.000000000000000000, 0.000000000000000000, -1.000000000000000000 ) ) ;
#12169=TOROIDAL_SURFACE ( 'NONE', #19282, 3.606799999998999695, 0.7620000000000000107 ) ;
#12173=VERTEX_POINT ( 'NONE', #8554 ) ;
#12176=LINE ( 'NONE', #2211, #5453 ) ;
#12178=CARTESIAN_POINT ( 'NONE',  ( 8.088613972650000150, -3576.119152860999748, 2246.630000000000109 ) ) ;
#12179=CARTESIAN_POINT ( 'NONE',  ( 10.06210023420644184, -3658.439931164731206, 2249.672963766948669 ) ) ;
#12181=CARTESIAN_POINT ( 'NONE',  ( 132.0879339926999876, -3694.758336080999925, 2260.533847755999886 ) ) ;
#12183=ORIENTED_EDGE ( 'NONE', *, *, #14591, .F. ) ;
#12186=CIRCLE ( 'NONE', #14065, 1.269999999999882334 ) ;
#12188=ORIENTED_EDGE ( 'NONE', *, *, #23160, .F. ) ;
#12189=CARTESIAN_POINT ( 'NONE',  ( 131.9181769293102207, -3695.361398937724971, 2260.194562468291679 ) ) ;
#12192=CARTESIAN_POINT ( 'NONE',  ( 54.40679999999999694, -3670.300000000000182, 2239.771999999999935 ) ) ;
#12194=CARTESIAN_POINT ( 'NONE',  ( 133.9990844033331427, -3659.101433724999879, 2244.742833232057365 ) ) ;
#12199=DIRECTION ( 'NONE',  ( 0.000000000000000000, 0.000000000000000000, 1.000000000000000000 ) ) ;
#12200=CARTESIAN_POINT ( 'NONE',  ( 127.0000000000000000, -3568.700000000000273, 2259.837999999999738 ) ) ;
#12203=CIRCLE ( 'NONE', #10721, 3.606800000000000228 ) ;
#12205=DIRECTION ( 'NONE',  ( 1.000000000000000000, 0.000000000000000000, 0.000000000000000000 ) ) ;
#12206=CIRCLE ( 'NONE', #15204, 0.7619999999999294005 ) ;
#12207=VERTEX_POINT ( 'NONE', #3266 ) ;
#12209=CARTESIAN_POINT ( 'NONE',  ( 127.0000000000000000, -3619.500000000000000, 2260.600000000000364 ) ) ;
#12211=VERTEX_POINT ( 'NONE', #21211 ) ;
#12212=CARTESIAN_POINT ( 'NONE',  ( 10.16000000000000014, -3658.223872745999870, 2255.774000000000342 ) ) ;
#12213=CARTESIAN_POINT ( 'NONE',  ( 15.47556979461559123, -3660.128696051647694, 2250.236801090939025 ) ) ;
#12216=B_SPLINE_CURVE_WITH_KNOTS ( 'NONE', 3,
 ( #8498, #3092, #15643, #6979 ),
 .UNSPECIFIED., .F., .F.,
 ( 4, 4 ),
 ( 0.000000000000000000, 1.000000000000000000 ),
 .UNSPECIFIED. ) ;
#12217=DIRECTION ( 'NONE',  ( 0.000000000000000000, 0.000000000000000000, -1.000000000000000000 ) ) ;
#12219=EDGE_CURVE ( 'NONE', #15231, #11877, #3379, .T. ) ;
#12223=CARTESIAN_POINT ( 'NONE',  ( 18.37619926079141308, -3580.159608052614658, 2244.861392947899731 ) ) ;
#12226=CARTESIAN_POINT ( 'NONE',  ( 141.8375137957061156, -3657.627758956946764, 2248.726790701012305 ) ) ;
#12231=EDGE_LOOP ( 'NONE', ( #12917, #10556, #2995, #11969 ) ) ;
#12237=ORIENTED_EDGE ( 'NONE', *, *, #18401, .F. ) ;
#12238=DIRECTION ( 'NONE',  ( 0.000000000000000000, 1.000000000000000000, 0.000000000000000000 ) ) ;
#12240=DIRECTION ( 'NONE',  ( 0.000000000000000000, -1.000000000000000000, 0.000000000000000000 ) ) ;
#12241=CIRCLE ( 'NONE', #17846, 2.844800000000091700 ) ;
#12242=DIRECTION ( 'NONE',  ( 0.000000000000000000, 0.000000000000000000, -1.000000000000000000 ) ) ;
#12244=DIRECTION ( 'NONE',  ( 0.000000000000000000, 0.000000000000000000, 1.000000000000000000 ) ) ;
#12245=EDGE_CURVE ( 'NONE', #20246, #14593, #1299, .T. ) ;
#12247=DIRECTION ( 'NONE',  ( 0.000000000000000000, 0.000000000000000000, 1.000000000000000000 ) ) ;
#12249=CARTESIAN_POINT ( 'NONE',  ( 142.2400000000000091, -3660.786127253999894, 2255.774000000000342 ) ) ;
#12250=EDGE_CURVE ( 'NONE', #21408, #8087, #21161, .T. ) ;
#12256=CARTESIAN_POINT ( 'NONE',  ( 10.05562585061285219, -3580.543848469380919, 2249.684969000971705 ) ) ;
#12258=ORIENTED_EDGE ( 'NONE', *, *, #11274, .T. ) ;
#12259=DIRECTION ( 'NONE',  ( -1.000000000000000000, 0.000000000000000000, 0.000000000000000000 ) ) ;
#12262=AXIS2_PLACEMENT_3D ( 'NONE', #7133, #1971, #19548 ) ;
#12263=AXIS2_PLACEMENT_3D ( 'NONE', #9846, #18996, #10075 ) ;
#12264=ADVANCED_FACE ( 'NONE', ( #5263 ), #17911, .F. ) ;
#12266=CARTESIAN_POINT ( 'NONE',  ( 123.3932000000010021, -3670.300000000000182, 2239.771999999999935 ) ) ;
#12267=CARTESIAN_POINT ( 'NONE',  ( 11.02929805643817396, -3661.807647569477467, 2249.696627142566285 ) ) ;
#12272=AXIS2_PLACEMENT_3D ( 'NONE', #19021, #4486, #9344 ) ;
#12274=CARTESIAN_POINT ( 'NONE',  ( 14.66806072689505314, -3657.450396280145469, 2248.320112768498348 ) ) ;
#12277=DIRECTION ( 'NONE',  ( 0.000000000000000000, 1.000000000000000000, 1.224646799147353207E-16 ) ) ;
#12282=LINE ( 'NONE', #10516, #18253 ) ;
#12285=FACE_OUTER_BOUND ( 'NONE', #5586, .T. ) ;
#12287=DIRECTION ( 'NONE',  ( -1.000000000000000000, 0.000000000000000000, 0.000000000000000000 ) ) ;
#12291=AXIS2_PLACEMENT_3D ( 'NONE', #2372, #2590, #15135 ) ;
#12294=ORIENTED_EDGE ( 'NONE', *, *, #3343, .F. ) ;
#12297=ORIENTED_EDGE ( 'NONE', *, *, #22463, .F. ) ;
#12300=ADVANCED_FACE ( 'NONE', ( #448 ), #9130, .F. ) ;
#12301=ORIENTED_EDGE ( 'NONE', *, *, #5391, .F. ) ;
#12307=CYLINDRICAL_SURFACE ( 'NONE', #6460, 1.269999999999900320 ) ;
#12312=ADVANCED_FACE ( 'NONE', ( #336 ), #7683, .T. ) ;
#12313=CARTESIAN_POINT ( 'NONE',  ( 145.4150000000009868, -3579.494999999999891, 2239.771999999999935 ) ) ;
#12314=CARTESIAN_POINT ( 'NONE',  ( 15.06015184098700743, -3581.085670991564712, 2249.167371890592221 ) ) ;
#12316=DIRECTION ( 'NONE',  ( 0.000000000000000000, 0.000000000000000000, -1.000000000000000000 ) ) ;
#12317=DIRECTION ( 'NONE',  ( 0.000000000000000000, 0.000000000000000000, 1.000000000000000000 ) ) ;
#12319=CARTESIAN_POINT ( 'NONE',  ( 15.38815085373434322, -3695.327183877504467, 2255.402917874296691 ) ) ;
#12320=CARTESIAN_POINT ( 'NONE',  ( 97.99320000000000164, -3619.500000000000000, 2259.837999999999738 ) ) ;
#12321=ORIENTED_EDGE ( 'NONE', *, *, #5855, .F. ) ;
#12328=ORIENTED_EDGE ( 'NONE', *, *, #12145, .F. ) ;
#12329=CARTESIAN_POINT ( 'NONE',  ( 139.6999999999999886, -3579.494999999999891, 2239.771999999999935 ) ) ;
#12333=AXIS2_PLACEMENT_3D ( 'NONE', #10490, #17632, #1464 ) ;
#12337=AXIS2_PLACEMENT_3D ( 'NONE', #13053, #22172, #9529 ) ;
#12340=B_SPLINE_CURVE_WITH_KNOTS ( 'NONE', 3,
 ( #18941, #8278, #15200, #22439 ),
 .UNSPECIFIED., .F., .F.,
 ( 4, 4 ),
 ( 0.000000000000000000, 1.000000000000000000 ),
 .UNSPECIFIED. ) ;
#12344=ORIENTED_EDGE ( 'NONE', *, *, #1712, .F. ) ;
#12345=EDGE_LOOP ( 'NONE', ( #16980, #357, #21370 ) ) ;
#12346=CIRCLE ( 'NONE', #7481, 0.7619999999999294005 ) ;
#12349=VERTEX_POINT ( 'NONE', #20028 ) ;
#12351=CARTESIAN_POINT ( 'NONE',  ( 142.2400000000000091, -3660.786127253999894, 2255.774000000000342 ) ) ;
#12355=CARTESIAN_POINT ( 'NONE',  ( 47.19319999999999737, -3568.700000000000273, 2260.600000000000364 ) ) ;
#12356=EDGE_LOOP ( 'NONE', ( #22667, #4500, #6804, #21707 ) ) ;
#12358=FACE_BOUND ( 'NONE', #16437, .T. ) ;
#12363=CYLINDRICAL_SURFACE ( 'NONE', #9783, 1.269999999999882334 ) ;
#12364=AXIS2_PLACEMENT_3D ( 'NONE', #23155, #10758, #7131 ) ;
#12366=CARTESIAN_POINT ( 'NONE',  ( 10.10178836517258283, -3580.656260792020021, 2249.599788755271220 ) ) ;
#12370=VERTEX_POINT ( 'NONE', #108 ) ;
#12371=DIRECTION ( 'NONE',  ( 1.000000000000000000, 0.000000000000000000, 0.000000000000000000 ) ) ;
#12374=CARTESIAN_POINT ( 'NONE',  ( 0.000000000000000000, -3543.299999999999727, 2260.600000000000364 ) ) ;
#12375=CARTESIAN_POINT ( 'NONE',  ( 127.0000000000000000, -3619.500000000000000, 2239.771999999999935 ) ) ;
#12376=CARTESIAN_POINT ( 'NONE',  ( 10.58626199040230986, -3661.408970440582834, 2249.938111678748555 ) ) ;
#12382=DIRECTION ( 'NONE',  ( -1.000000000000000000, 0.000000000000000000, 0.000000000000000000 ) ) ;
#12384=CARTESIAN_POINT ( 'NONE',  ( 14.85465215501677605, -3657.647354326531513, 2248.763246533717393 ) ) ;
#12385=EDGE_CURVE ( 'NONE', #572, #17725, #22069, .T. ) ;
#12386=CARTESIAN_POINT ( 'NONE',  ( 136.8942325653789851, -3695.547111921297528, 2255.108514516369269 ) ) ;
#12390=CARTESIAN_POINT ( 'NONE',  ( 10.34103833421398377, -3577.903977763734019, 2250.071793175431594 ) ) ;
#12392=CARTESIAN_POINT ( 'NONE',  ( 132.1456718464000062, -3544.321224993999749, 2260.506484774000000 ) ) ;
#12394=CARTESIAN_POINT ( 'NONE',  ( 15.24000000000000021, -3660.786127253999894, 2255.774000000000342 ) ) ;
#12396=CIRCLE ( 'NONE', #2647, 2.844799999998998796 ) ;
#12399=CARTESIAN_POINT ( 'NONE',  ( 15.74606938694885550, -3657.399157459567505, 2246.629983459085906 ) ) ;
#12401=CARTESIAN_POINT ( 'NONE',  ( 95.25000000000000000, -3695.699999999999818, 2247.392000000000280 ) ) ;
#12402=LINE ( 'NONE', #1494, #16233 ) ;
#12406=CARTESIAN_POINT ( 'NONE',  ( 114.2999999999999972, -3644.899999999999636, 2239.771999999999935 ) ) ;
#12407=EDGE_CURVE ( 'NONE', #11149, #11279, #11421, .T. ) ;
#12408=DIRECTION ( 'NONE',  ( -0.000000000000000000, -1.000000000000000000, -0.000000000000000000 ) ) ;
#12412=ADVANCED_FACE ( 'NONE', ( #18029 ), #16387, .F. ) ;
#12415=VERTEX_POINT ( 'NONE', #8174 ) ;
#12417=CARTESIAN_POINT ( 'NONE',  ( 142.4730284656999970, -3660.140000970000074, 2250.236800000000130 ) ) ;
#12419=CARTESIAN_POINT ( 'NONE',  ( 136.8552000000000248, -3579.666931380626011, 2250.125652639312193 ) ) ;
#12420=ORIENTED_EDGE ( 'NONE', *, *, #14245, .F. ) ;
#12422=FACE_OUTER_BOUND ( 'NONE', #7354, .T. ) ;
#12424=CARTESIAN_POINT ( 'NONE',  ( 110.6932000000009992, -3644.899999999999636, 2239.009999999999764 ) ) ;
#12426=VECTOR ( 'NONE', #11366, 1000.000000000000000 ) ;
#12427=FACE_OUTER_BOUND ( 'NONE', #9091, .T. ) ;
#12428=ORIENTED_EDGE ( 'NONE', *, *, #5855, .T. ) ;
#12430=ORIENTED_EDGE ( 'NONE', *, *, #8253, .T. ) ;
#12431=CARTESIAN_POINT ( 'NONE',  ( 4.926382664726756566, -3695.340677395856801, 2260.215245127323669 ) ) ;
#12433=CIRCLE ( 'NONE', #16548, 2.844799999999961582 ) ;
#12435=EDGE_CURVE ( 'NONE', #16091, #17137, #20410, .T. ) ;
#12436=EDGE_CURVE ( 'NONE', #17069, #14185, #7327, .T. ) ;
#12437=FACE_OUTER_BOUND ( 'NONE', #15318, .T. ) ;
#12439=EDGE_CURVE ( 'NONE', #6183, #10881, #4323, .T. ) ;
#12441=AXIS2_PLACEMENT_3D ( 'NONE', #19339, #7044, #6808 ) ;
#12442=LINE ( 'NONE', #8815, #20043 ) ;
#12445=DIRECTION ( 'NONE',  ( 0.000000000000000000, 0.000000000000000000, -1.000000000000000000 ) ) ;
#12448=EDGE_CURVE ( 'NONE', #19621, #1443, #22357, .T. ) ;
#12455=VECTOR ( 'NONE', #17139, 1000.000000000000000 ) ;
#12457=CARTESIAN_POINT ( 'NONE',  ( 137.2370452280314055, -3658.078236828710487, 2249.356016053515305 ) ) ;
#12458=EDGE_CURVE ( 'NONE', #7639, #7043, #219, .T. ) ;
#12461=CARTESIAN_POINT ( 'NONE',  ( 47.19319999999999737, -3670.300000000000182, 2259.837999999999738 ) ) ;
#12462=TOROIDAL_SURFACE ( 'NONE', #15087, 3.606799999999999784, 0.7620000000000000107 ) ;
#12466=DIRECTION ( 'NONE',  ( 1.000000000000000000, 0.000000000000000000, 0.000000000000000000 ) ) ;
#12467=ORIENTED_EDGE ( 'NONE', *, *, #20599, .F. ) ;
#12469=CARTESIAN_POINT ( 'NONE',  ( 1.270000000000000018, -3694.430000000000291, 2259.329999999999927 ) ) ;
#12475=FACE_BOUND ( 'NONE', #3407, .T. ) ;
#12478=DIRECTION ( 'NONE',  ( 0.000000000000000000, 1.000000000000000000, 0.000000000000000000 ) ) ;
#12481=AXIS2_PLACEMENT_3D ( 'NONE', #1297, #22966, #15486 ) ;
#12482=ORIENTED_EDGE ( 'NONE', *, *, #12075, .T. ) ;
#12483=CARTESIAN_POINT ( 'NONE',  ( 9.855390812759999619, -3579.528596999999991, 2250.157115725000040 ) ) ;
#12484=FACE_OUTER_BOUND ( 'NONE', #12693, .T. ) ;
#12485=PLANE ( 'NONE',  #20931 ) ;
#12488=DIRECTION ( 'NONE',  ( 0.000000000000000000, 0.000000000000000000, 1.000000000000000000 ) ) ;
#12489=LINE ( 'NONE', #3578, #21158 ) ;
#12494=CARTESIAN_POINT ( 'NONE',  ( 147.7813569001403380, -3543.300000000019736, 2259.444513955824277 ) ) ;
#12495=ORIENTED_EDGE ( 'NONE', *, *, #10421, .F. ) ;
#12497=DIRECTION ( 'NONE',  ( -1.000000000000000000, 0.000000000000000000, 0.000000000000000000 ) ) ;
#12500=CARTESIAN_POINT ( 'NONE',  ( 14.98249584125296430, -3657.807061604205046, 2249.020059837405825 ) ) ;
#12503=CARTESIAN_POINT ( 'NONE',  ( 9.855200000000998273, -3659.504999999999654, 2256.063560000000052 ) ) ;
#12506=CARTESIAN_POINT ( 'NONE',  ( 132.3005794017000198, -3544.570000000000164, 2260.390449568000349 ) ) ;
#12508=FACE_OUTER_BOUND ( 'NONE', #20212, .T. ) ;
#12512=CARTESIAN_POINT ( 'NONE',  ( 92.50679999999999836, -3644.899999999999636, 2239.771999999999935 ) ) ;
#12513=LINE ( 'NONE', #19660, #15952 ) ;
#12515=CARTESIAN_POINT ( 'NONE',  ( 91.74479999999999791, -3644.899999999999636, 2259.837999999999738 ) ) ;
#12516=ADVANCED_FACE ( 'NONE', ( #1010 ), #4530, .F. ) ;
#12517=EDGE_LOOP ( 'NONE', ( #12549, #19214, #1796, #4298 ) ) ;
#12518=DIRECTION ( 'NONE',  ( 0.000000000000000000, 0.000000000000000000, 1.000000000000000000 ) ) ;
#12519=ORIENTED_EDGE ( 'NONE', *, *, #5347, .F. ) ;
#12521=CARTESIAN_POINT ( 'NONE',  ( 95.25000000000000000, -3544.570000000000164, 2243.277199999999993 ) ) ;
#12522=CIRCLE ( 'NONE', #2421, 3.606800000000000228 ) ;
#12523=CARTESIAN_POINT ( 'NONE',  ( 25.39999999999999858, -3578.860000000000127, 2247.392000000000280 ) ) ;
#12526=DIRECTION ( 'NONE',  ( 0.000000000000000000, 0.000000000000000000, -1.000000000000000000 ) ) ;
#12528=CARTESIAN_POINT ( 'NONE',  ( 142.5418463402332634, -3695.591362400878552, 2255.017959195591175 ) ) ;
#12529=ORIENTED_EDGE ( 'NONE', *, *, #690, .T. ) ;
#12531=CARTESIAN_POINT ( 'NONE',  ( 137.4922034527655512, -3581.289558263637446, 2248.872981960140805 ) ) ;
#12533=ORIENTED_EDGE ( 'NONE', *, *, #17556, .T. ) ;
#12535=TOROIDAL_SURFACE ( 'NONE', #6200, 3.606799999999999784, 0.7620000000000000107 ) ;
#12536=ADVANCED_FACE ( 'NONE', ( #11559 ), #15547, .T. ) ;
#12539=ADVANCED_FACE ( 'NONE', ( #13676 ), #18482, .T. ) ;
#12540=AXIS2_PLACEMENT_3D ( 'NONE', #21031, #15517, #3322 ) ;
#12541=DIRECTION ( 'NONE',  ( 1.000000000000000000, -0.000000000000000000, -0.000000000000000000 ) ) ;
#12545=DIRECTION ( 'NONE',  ( 0.000000000000000000, 0.000000000000000000, -1.000000000000000000 ) ) ;
#12547=CARTESIAN_POINT ( 'NONE',  ( 134.6666709697134650, -3576.788180027481758, 2245.442509231440454 ) ) ;
#12549=ORIENTED_EDGE ( 'NONE', *, *, #18815, .F. ) ;
#12550=AXIS2_PLACEMENT_3D ( 'NONE', #18428, #13386, #838 ) ;
#12554=DIRECTION ( 'NONE',  ( -1.000000000000000000, 0.000000000000000000, 0.000000000000000000 ) ) ;
#12558=CARTESIAN_POINT ( 'NONE',  ( 88.90000000000000568, -3644.899999999999636, 2239.771999999999935 ) ) ;
#12563=FACE_BOUND ( 'NONE', #12003, .T. ) ;
#12564=LINE ( 'NONE', #19720, #9606 ) ;
#12568=CARTESIAN_POINT ( 'NONE',  ( 9.842801829194641527, -3695.607672421227107, 2254.979458605150285 ) ) ;
#12569=EDGE_LOOP ( 'NONE', ( #21830, #1681, #8927, #22574 ) ) ;
#12573=ADVANCED_FACE ( 'NONE', ( #9693 ), #22610, .T. ) ;
#12575=CIRCLE ( 'NONE', #1717, 2.844799999999994444 ) ;
#12576=EDGE_CURVE ( 'NONE', #4163, #9004, #16252, .T. ) ;
#12581=ORIENTED_EDGE ( 'NONE', *, *, #13517, .T. ) ;
#12586=ORIENTED_EDGE ( 'NONE', *, *, #19769, .T. ) ;
#12587=EDGE_LOOP ( 'NONE', ( #10009, #375, #8490, #6738 ) ) ;
#12591=AXIS2_PLACEMENT_3D ( 'NONE', #9770, #16914, #859 ) ;
#12592=FACE_OUTER_BOUND ( 'NONE', #9136, .T. ) ;
#12596=CARTESIAN_POINT ( 'NONE',  ( 151.1299999999999955, -3578.860000000000127, 2244.547199999999975 ) ) ;
#12599=CARTESIAN_POINT ( 'NONE',  ( 7.048736936763374317, -3580.386377785101104, 2244.978268890040454 ) ) ;
#12603=ORIENTED_EDGE ( 'NONE', *, *, #6677, .F. ) ;
#12604=CARTESIAN_POINT ( 'NONE',  ( 131.7384701241167022, -3543.369601860909370, 2259.744672092661858 ) ) ;
#12605=ORIENTED_EDGE ( 'NONE', *, *, #13453, .F. ) ;
#12606=CARTESIAN_POINT ( 'NONE',  ( 66.34479999999999222, -3594.099999999999909, 2259.837999999999738 ) ) ;
#12608=CARTESIAN_POINT ( 'NONE',  ( 66.34479999999999222, -3644.899999999999636, 2261.869999999999891 ) ) ;
#12611=AXIS2_PLACEMENT_3D ( 'NONE', #2394, #20529, #20319 ) ;
#12613=LINE ( 'NONE', #14256, #11838 ) ;
#12614=AXIS2_PLACEMENT_3D ( 'NONE', #15688, #15451, #15572 ) ;
#12615=DIRECTION ( 'NONE',  ( 1.000000000000000000, 0.000000000000000000, 0.000000000000000000 ) ) ;
#12617=FACE_OUTER_BOUND ( 'NONE', #2269, .T. ) ;
#12618=DIRECTION ( 'NONE',  ( -1.000000000000000000, 0.000000000000000000, 0.000000000000000000 ) ) ;
#12619=EDGE_LOOP ( 'NONE', ( #16860, #3553 ) ) ;
#12620=CARTESIAN_POINT ( 'NONE',  ( 147.4427463453449718, -3695.258941567852162, 2260.292568422380100 ) ) ;
#12621=DIRECTION ( 'NONE',  ( -1.000000000000000000, 0.000000000000000000, 0.000000000000000000 ) ) ;
#12623=CARTESIAN_POINT ( 'NONE',  ( 142.5448000000000093, -3579.282532373467347, 2250.213677521736827 ) ) ;
#12624=CARTESIAN_POINT ( 'NONE',  ( 142.4037490354116926, -3543.632335306846016, 2255.363857416194605 ) ) ;
#12625=CARTESIAN_POINT ( 'NONE',  ( 136.6529205195000145, -3695.699999999999818, 2254.503999999999905 ) ) ;
#12626=VERTEX_POINT ( 'NONE', #10621 ) ;
#12627=CARTESIAN_POINT ( 'NONE',  ( 50.79999999999999716, -3568.700000000000273, 2259.837999999999738 ) ) ;
#12630=CARTESIAN_POINT ( 'NONE',  ( 9.998032641076921578, -3543.639179023070028, 2255.368368629587167 ) ) ;
#12633=TOROIDAL_SURFACE ( 'NONE', #4033, 6.477000000001000402, 0.7620000000000000107 ) ;
#12635=CARTESIAN_POINT ( 'NONE',  ( 116.8400000000000034, -3568.700000000000273, 2247.392000000000280 ) ) ;
#12636=CARTESIAN_POINT ( 'NONE',  ( 151.4000000000000057, -3544.570000000000164, 2259.329999999999927 ) ) ;
#12637=DIRECTION ( 'NONE',  ( -0.000000000000000000, 1.000000000000000000, 0.000000000000000000 ) ) ;
#12638=VERTEX_POINT ( 'NONE', #19183 ) ;
#12640=TOROIDAL_SURFACE ( 'NONE', #22354, 3.606799999998999695, 0.7620000000000000107 ) ;
#12641=EDGE_CURVE ( 'NONE', #14185, #17069, #14017, .T. ) ;
#12646=CARTESIAN_POINT ( 'NONE',  ( 142.3028687989565526, -3695.048176945954765, 2255.616383243821019 ) ) ;
#12647=DIRECTION ( 'NONE',  ( 0.000000000000000000, 0.000000000000000000, 1.000000000000000000 ) ) ;
#12648=EDGE_LOOP ( 'NONE', ( #143, #4319, #5578, #18513 ) ) ;
#12649=CARTESIAN_POINT ( 'NONE',  ( 137.1922541308920813, -3580.838518559781278, 2249.436926605831559 ) ) ;
#12650=ORIENTED_EDGE ( 'NONE', *, *, #7703, .F. ) ;
#12651=DIRECTION ( 'NONE',  ( -1.000000000000000000, 0.000000000000000000, 0.000000000000000000 ) ) ;
#12656=CARTESIAN_POINT ( 'NONE',  ( 116.8400000000000034, -3568.700000000000273, 2244.547199999999975 ) ) ;
#12658=DIRECTION ( 'NONE',  ( 0.000000000000000000, 0.000000000000000000, 1.000000000000000000 ) ) ;
#12659=CARTESIAN_POINT ( 'NONE',  ( 141.8559770206331621, -3577.638865271226223, 2249.961452083505264 ) ) ;
#12660=ORIENTED_EDGE ( 'NONE', *, *, #15533, .F. ) ;
#12661=CARTESIAN_POINT ( 'NONE',  ( 134.1130506821819779, -3578.283485894974547, 2244.602361446803570 ) ) ;
#12663=ORIENTED_EDGE ( 'NONE', *, *, #3476, .F. ) ;
#12664=FACE_OUTER_BOUND ( 'NONE', #12914, .T. ) ;
#12665=ORIENTED_EDGE ( 'NONE', *, *, #1334, .F. ) ;
#12668=VERTEX_POINT ( 'NONE', #1594 ) ;
#12670=EDGE_CURVE ( 'NONE', #17227, #15883, #17000, .T. ) ;
#12672=DIRECTION ( 'NONE',  ( -0.6723379328325259641, -0.7402443543009875615, 0.000000000000000000 ) ) ;
#12674=AXIS2_PLACEMENT_3D ( 'NONE', #13331, #2657, #2552 ) ;
#12675=ORIENTED_EDGE ( 'NONE', *, *, #22429, .F. ) ;
#12680=B_SPLINE_CURVE_WITH_KNOTS ( 'NONE', 3,
 ( #4948, #12213, #21245, #3182, #2954, #17351, #13976, #10216, #12094, #15732 ),
 .UNSPECIFIED., .F., .F.,
 ( 4, 2, 1, 1, 2, 4 ),
 ( 0.000000000000000000, 0.06250000000002454981, 0.1250000000000490996, 0.2500000000000422440, 0.5000000000000285327, 1.000000000000000000 ),
 .UNSPECIFIED. ) ;
#12682=DIRECTION ( 'NONE',  ( 0.000000000000000000, 0.000000000000000000, -1.000000000000000000 ) ) ;
#12685=CARTESIAN_POINT ( 'NONE',  ( 9.738066884983357596, -3695.684982104192841, 2254.716481487530018 ) ) ;
#12686=EDGE_LOOP ( 'NONE', ( #3690, #11551 ) ) ;
#12687=CARTESIAN_POINT ( 'NONE',  ( 18.07271388913700250, -3581.449656630049049, 2246.178647457765692 ) ) ;
#12689=CARTESIAN_POINT ( 'NONE',  ( 137.6157805523781690, -3657.568573254816783, 2248.609408014333439 ) ) ;
#12692=CARTESIAN_POINT ( 'NONE',  ( 140.1748344546939506, -3662.310676981497636, 2249.230826604551567 ) ) ;
#12693=EDGE_LOOP ( 'NONE', ( #15172, #12717, #18747, #18907 ) ) ;
#12694=ORIENTED_EDGE ( 'NONE', *, *, #5643, .F. ) ;
#12699=CARTESIAN_POINT ( 'NONE',  ( 142.2400000000000091, -3660.786127253999894, 2255.774000000000342 ) ) ;
#12703=DIRECTION ( 'NONE',  ( -1.000000000000000000, 0.000000000000000000, 0.000000000000000000 ) ) ;
#12705=EDGE_CURVE ( 'NONE', #923, #10278, #164, .T. ) ;
#12708=DIRECTION ( 'NONE',  ( 0.000000000000000000, 0.000000000000000000, 1.000000000000000000 ) ) ;
#12710=CARTESIAN_POINT ( 'NONE',  ( 7.375511700031431417, -3581.571545880435679, 2246.524605943541246 ) ) ;
#12715=ORIENTED_EDGE ( 'NONE', *, *, #15817, .T. ) ;
#12717=ORIENTED_EDGE ( 'NONE', *, *, #9997, .F. ) ;
#12718=EDGE_CURVE ( 'NONE', #16380, #16556, #11915, .T. ) ;
#12723=DIRECTION ( 'NONE',  ( 0.000000000000000000, 1.000000000000000000, 0.000000000000000000 ) ) ;
#12725=CYLINDRICAL_SURFACE ( 'NONE', #9570, 2.844799999999999773 ) ;
#12727=CARTESIAN_POINT ( 'NONE',  ( 147.3506313851963228, -3694.866442831903896, 2260.523303096903874 ) ) ;
#12729=CARTESIAN_POINT ( 'NONE',  ( 1.270000000000000018, -3544.570000000000164, 2239.009999999999764 ) ) ;
#12731=CARTESIAN_POINT ( 'NONE',  ( 54.40679999999999694, -3670.300000000000182, 2260.600000000000364 ) ) ;
#12732=CARTESIAN_POINT ( 'NONE',  ( 142.5947367361206943, -3543.355825690155598, 2254.886265305463439 ) ) ;
#12734=CARTESIAN_POINT ( 'NONE',  ( 7.827395171519881067, -3576.508546973163902, 2245.790855086235297 ) ) ;
#12738=CARTESIAN_POINT ( 'NONE',  ( 41.70680000000000121, -3644.899999999999636, 2260.600000000000364 ) ) ;
#12739=TOROIDAL_SURFACE ( 'NONE', #21684, 3.606799999999999784, 0.7620000000000000107 ) ;
#12744=FACE_OUTER_BOUND ( 'NONE', #20922, .T. ) ;
#12746=EDGE_CURVE ( 'NONE', #21153, #10346, #7456, .T. ) ;
#12747=ADVANCED_FACE ( 'NONE', ( #14611 ), #8778, .T. ) ;
#12748=DIRECTION ( 'NONE',  ( -1.000000000000000000, -2.186138625658999988E-13, 0.000000000000000000 ) ) ;
#12749=LINE ( 'NONE', #21660, #1637 ) ;
#12753=ORIENTED_EDGE ( 'NONE', *, *, #12865, .F. ) ;
#12757=CIRCLE ( 'NONE', #11616, 2.844799999999009010 ) ;
#12759=CARTESIAN_POINT ( 'NONE',  ( 142.4037675250975781, -3695.367664690104903, 2255.363864802005537 ) ) ;
#12761=ORIENTED_EDGE ( 'NONE', *, *, #11861, .F. ) ;
#12763=CARTESIAN_POINT ( 'NONE',  ( 137.5699719362845883, -3581.380703542814899, 2248.710691103632143 ) ) ;
#12768=CARTESIAN_POINT ( 'NONE',  ( 25.39999999999999858, -3578.860000000000127, 2250.236800000000130 ) ) ;
#12770=DIRECTION ( 'NONE',  ( 0.000000000000000000, 0.000000000000000000, -1.000000000000000000 ) ) ;
#12772=CARTESIAN_POINT ( 'NONE',  ( 141.8954864283250572, -3577.685780687507759, 2249.983218200938154 ) ) ;
#12775=CARTESIAN_POINT ( 'NONE',  ( 134.8860662734080051, -3576.414507136522843, 2245.937534930719721 ) ) ;
#12780=FACE_OUTER_BOUND ( 'NONE', #19191, .T. ) ;
#12782=ORIENTED_EDGE ( 'NONE', *, *, #7283, .T. ) ;
#12783=LINE ( 'NONE', #1887, #15028 ) ;
#12787=DIRECTION ( 'NONE',  ( 0.000000000000000000, 0.000000000000000000, 1.000000000000000000 ) ) ;
#12794=AXIS2_PLACEMENT_3D ( 'NONE', #11147, #141, #9390 ) ;
#12796=CARTESIAN_POINT ( 'NONE',  ( 1.270000000000000018, -3543.299999999999727, 2259.329999999999927 ) ) ;
#12800=EDGE_CURVE ( 'NONE', #4712, #15879, #17755, .T. ) ;
#12802=CARTESIAN_POINT ( 'NONE',  ( 137.7992377516491729, -3657.388364312606882, 2248.114380174669350 ) ) ;
#12803=ORIENTED_EDGE ( 'NONE', *, *, #1625, .F. ) ;
#12804=EDGE_LOOP ( 'NONE', ( #9779, #1427 ) ) ;
#12806=CARTESIAN_POINT ( 'NONE',  ( 138.7492288098038955, -3662.186786022434262, 2249.367902486606908 ) ) ;
#12808=ORIENTED_EDGE ( 'NONE', *, *, #3409, .F. ) ;
#12811=VECTOR ( 'NONE', #18952, 1000.000000000000000 ) ;
#12813=ORIENTED_EDGE ( 'NONE', *, *, #1967, .T. ) ;
#12815=CARTESIAN_POINT ( 'NONE',  ( 95.25000000000000000, -3670.300000000000182, 2247.392000000000280 ) ) ;
#12816=EDGE_CURVE ( 'NONE', #2862, #1856, #12891, .T. ) ;
#12821=CARTESIAN_POINT ( 'NONE',  ( 7.279738514679607420, -3581.306672009827253, 2245.940466658847527 ) ) ;
#12822=DIRECTION ( 'NONE',  ( 0.000000000000000000, -1.000000000000000000, 0.000000000000000000 ) ) ;
#12823=AXIS2_PLACEMENT_3D ( 'NONE', #521, #2614, #4266 ) ;
#12825=CARTESIAN_POINT ( 'NONE',  ( 132.0583097651000060, -3544.202533098000458, 2260.545675974999995 ) ) ;
#12827=CIRCLE ( 'NONE', #2709, 2.844800000000091700 ) ;
#12832=DIRECTION ( 'NONE',  ( 0.000000000000000000, -1.000000000000000000, 0.000000000000000000 ) ) ;
#12835=DIRECTION ( 'NONE',  ( 0.000000000000000000, 1.000000000000000000, 0.000000000000000000 ) ) ;
#12836=AXIS2_PLACEMENT_3D ( 'NONE', #8265, #11428, #8034 ) ;
#12837=AXIS2_PLACEMENT_3D ( 'NONE', #5284, #12658, #16058 ) ;
#12839=VERTEX_POINT ( 'NONE', #14843 ) ;
#12846=AXIS2_PLACEMENT_3D ( 'NONE', #8689, #19006, #4704 ) ;
#12847=DIRECTION ( 'NONE',  ( 0.9999999999969670927, 2.462891091727920355E-06, 0.000000000000000000 ) ) ;
#12848=CARTESIAN_POINT ( 'NONE',  ( 142.3391676994775707, -3543.814512434918015, 2255.525709086601182 ) ) ;
#12850=CARTESIAN_POINT ( 'NONE',  ( 7.338124605662116551, -3577.517127564773546, 2244.882856471110699 ) ) ;
#12851=ORIENTED_EDGE ( 'NONE', *, *, #7703, .T. ) ;
#12854=FACE_OUTER_BOUND ( 'NONE', #22576, .T. ) ;
#12865=EDGE_CURVE ( 'NONE', #7211, #16324, #19632, .T. ) ;
#12867=VERTEX_POINT ( 'NONE', #21640 ) ;
#12868=CARTESIAN_POINT ( 'NONE',  ( 136.8551999999999964, -3579.494999999999891, 2256.063560000000052 ) ) ;
#12869=ORIENTED_EDGE ( 'NONE', *, *, #19465, .T. ) ;
#12871=ORIENTED_EDGE ( 'NONE', *, *, #14939, .F. ) ;
#12872=ADVANCED_FACE ( 'NONE', ( #78 ), #10644, .T. ) ;
#12876=DIRECTION ( 'NONE',  ( 0.000000000000000000, 0.000000000000000000, -1.000000000000000000 ) ) ;
#12879=ORIENTED_EDGE ( 'NONE', *, *, #17396, .F. ) ;
#12880=EDGE_CURVE ( 'NONE', #22049, #5314, #11685, .T. ) ;
#12881=CARTESIAN_POINT ( 'NONE',  ( 137.6646844684655662, -3581.483553633650899, 2248.496591272957176 ) ) ;
#12882=VERTEX_POINT ( 'NONE', #18574 ) ;
#12891=CIRCLE ( 'NONE', #20746, 3.606799999998994366 ) ;
#12892=CARTESIAN_POINT ( 'NONE',  ( 137.9713325200793292, -3577.235569966525418, 2249.727464718754163 ) ) ;
#12894=CARTESIAN_POINT ( 'NONE',  ( 134.4866660653693202, -3577.153554363255353, 2245.115832528504598 ) ) ;
#12895=FACE_OUTER_BOUND ( 'NONE', #18182, .T. ) ;
#12904=CIRCLE ( 'NONE', #15144, 5.715000000001027480 ) ;
#12905=FACE_OUTER_BOUND ( 'NONE', #15173, .T. ) ;
#12906=FACE_OUTER_BOUND ( 'NONE', #18491, .T. ) ;
#12908=CARTESIAN_POINT ( 'NONE',  ( 116.8400000000000034, -3568.700000000000273, 2247.392000000000280 ) ) ;
#12913=DIRECTION ( 'NONE',  ( 0.000000000000000000, -1.000000000000000000, 0.000000000000000000 ) ) ;
#12914=EDGE_LOOP ( 'NONE', ( #9133, #18039, #700, #21923 ) ) ;
#12915=CARTESIAN_POINT ( 'NONE',  ( 18.17636274929951057, -3581.130155322544852, 2245.675470980243063 ) ) ;
#12917=ORIENTED_EDGE ( 'NONE', *, *, #5932, .F. ) ;
#12921=CARTESIAN_POINT ( 'NONE',  ( 139.1601031653451344, -3662.312941375153969, 2249.232129089474256 ) ) ;
#12923=AXIS2_PLACEMENT_3D ( 'NONE', #17322, #11474, #22362 ) ;
#12928=VERTEX_POINT ( 'NONE', #7913 ) ;
#12933=DIRECTION ( 'NONE',  ( -1.000000000000000000, 0.000000000000000000, 0.000000000000000000 ) ) ;
#12935=AXIS2_PLACEMENT_3D ( 'NONE', #20381, #2679, #9826 ) ;
#12943=CARTESIAN_POINT ( 'NONE',  ( 142.5260164572884491, -3659.173939949165742, 2250.068209961469165 ) ) ;
#12944=CARTESIAN_POINT ( 'NONE',  ( 7.603979357582005605, -3662.088066489251560, 2245.312755012078469 ) ) ;
#12945=B_SPLINE_CURVE_WITH_KNOTS ( 'NONE', 3,
 ( #2908, #11268, #5782, #17077 ),
 .UNSPECIFIED., .F., .F.,
 ( 4, 4 ),
 ( 0.000000000000000000, 1.000000000000000000 ),
 .UNSPECIFIED. ) ;
#12952=VECTOR ( 'NONE', #13095, 1000.000000000000000 ) ;
#12953=DIRECTION ( 'NONE',  ( 0.000000000000000000, 0.000000000000000000, 1.000000000000000000 ) ) ;
#12956=CARTESIAN_POINT ( 'NONE',  ( 147.6246907140292706, -3543.405519448600899, 2259.836836426394711 ) ) ;
#12959=CARTESIAN_POINT ( 'NONE',  ( 147.6218842717319717, -3695.591362401009519, 2259.843974340487421 ) ) ;
#12964=EDGE_CURVE ( 'NONE', #22920, #7890, #4272, .T. ) ;
#12965=AXIS2_PLACEMENT_3D ( 'NONE', #18819, #2889, #11910 ) ;
#12967=DIRECTION ( 'NONE',  ( -1.000000000000000000, 0.000000000000000000, 0.000000000000000000 ) ) ;
#12973=CARTESIAN_POINT ( 'NONE',  ( 145.0128742528000032, -3657.399152860999493, 2246.630000000000109 ) ) ;
#12980=ORIENTED_EDGE ( 'NONE', *, *, #10113, .T. ) ;
#12981=AXIS2_PLACEMENT_3D ( 'NONE', #3925, #642, #7335 ) ;
#12983=CIRCLE ( 'NONE', #2870, 0.7619999999999294005 ) ;
#12984=ORIENTED_EDGE ( 'NONE', *, *, #10137, .T. ) ;
#12986=ORIENTED_EDGE ( 'NONE', *, *, #21752, .F. ) ;
#12989=ORIENTED_EDGE ( 'NONE', *, *, #17658, .T. ) ;
#12991=AXIS2_PLACEMENT_3D ( 'NONE', #352, #1761, #11133 ) ;
#12992=DIRECTION ( 'NONE',  ( 0.000000000000000000, 1.000000000000000000, 0.000000000000000000 ) ) ;
#12995=DIRECTION ( 'NONE',  ( 0.000000000000000000, 0.000000000000000000, -1.000000000000000000 ) ) ;
#12998=CIRCLE ( 'NONE', #18242, 4.114799999999974034 ) ;
#12999=VERTEX_POINT ( 'NONE', #752 ) ;
#13000=EDGE_CURVE ( 'NONE', #2800, #18918, #16723, .T. ) ;
#13002=DIRECTION ( 'NONE',  ( 0.000000000000000000, 0.000000000000000000, -1.000000000000000000 ) ) ;
#13005=CARTESIAN_POINT ( 'NONE',  ( 145.3885918142797777, -3580.043763408794803, 2244.804994013378746 ) ) ;
#13008=DIRECTION ( 'NONE',  ( 0.000000000000000000, -1.000000000000000000, 0.000000000000000000 ) ) ;
#13013=CARTESIAN_POINT ( 'NONE',  ( 141.9354122741817150, -3577.734584490984162, 2250.005152421867933 ) ) ;
#13015=ADVANCED_FACE ( 'NONE', ( #11307 ), #18458, .F. ) ;
#13018=DIRECTION ( 'NONE',  ( 0.000000000000000000, 0.000000000000000000, 1.000000000000000000 ) ) ;
#13019=ORIENTED_EDGE ( 'NONE', *, *, #12245, .T. ) ;
#13023=AXIS2_PLACEMENT_3D ( 'NONE', #16448, #19980, #16342 ) ;
#13024=LINE ( 'NONE', #10416, #2678 ) ;
#13026=EDGE_LOOP ( 'NONE', ( #1889, #11436, #5159, #18695 ) ) ;
#13028=ADVANCED_FACE ( 'NONE', ( #1449 ), #5214, .T. ) ;
#13029=CARTESIAN_POINT ( 'NONE',  ( 14.48098936461540553, -3577.276529815265349, 2249.755429883363831 ) ) ;
#13031=CARTESIAN_POINT ( 'NONE',  ( 147.3199999999999932, -3695.699999999999818, 2260.600000000000364 ) ) ;
#13033=CARTESIAN_POINT ( 'NONE',  ( 95.25000000000000000, -3544.570000000000164, 2247.392000000000280 ) ) ;
#13037=DIRECTION ( 'NONE',  ( 0.000000000000000000, 0.000000000000000000, -1.000000000000000000 ) ) ;
#13039=CARTESIAN_POINT ( 'NONE',  ( 136.9337416949390729, -3658.818840990081753, 2249.918292882339756 ) ) ;
#13040=ORIENTED_EDGE ( 'NONE', *, *, #2901, .F. ) ;
#13041=CARTESIAN_POINT ( 'NONE',  ( 141.3692361696618320, -3661.808694985247257, 2249.696048052667720 ) ) ;
#13045=VERTEX_POINT ( 'NONE', #22770 ) ;
#13047=ORIENTED_EDGE ( 'NONE', *, *, #8678, .T. ) ;
#13052=CARTESIAN_POINT ( 'NONE',  ( 7.091956865061221471, -3658.404132852121620, 2245.137126576677019 ) ) ;
#13053=CARTESIAN_POINT ( 'NONE',  ( 101.5999999999999943, -3670.300000000000182, 2259.837999999999738 ) ) ;
#13055=CARTESIAN_POINT ( 'NONE',  ( 129.8447999999989975, -3619.500000000000000, 2239.771999999999935 ) ) ;
#13058=FACE_OUTER_BOUND ( 'NONE', #13740, .T. ) ;
#13059=ORIENTED_EDGE ( 'NONE', *, *, #15440, .F. ) ;
#13060=CIRCLE ( 'NONE', #10050, 2.844799999998995244 ) ;
#13062=ORIENTED_EDGE ( 'NONE', *, *, #4521, .F. ) ;
#13063=CARTESIAN_POINT ( 'NONE',  ( 130.6067999999989979, -3670.300000000000182, 2239.771999999999935 ) ) ;
#13064=ORIENTED_EDGE ( 'NONE', *, *, #6012, .T. ) ;
#13065=CYLINDRICAL_SURFACE ( 'NONE', #22309, 2.844800000000091700 ) ;
#13070=CARTESIAN_POINT ( 'NONE',  ( 147.5857674342917960, -3695.547111920908719, 2259.934514517091884 ) ) ;
#13072=CARTESIAN_POINT ( 'NONE',  ( 127.0000000000000000, -3670.300000000000182, 2239.009999999999764 ) ) ;
#13074=CARTESIAN_POINT ( 'NONE',  ( 142.7013568988404018, -3543.300000000001091, 2254.618513959080701 ) ) ;
#13076=CARTESIAN_POINT ( 'NONE',  ( 7.152845350294700033, -3578.119350159317491, 2244.644855890406689 ) ) ;
#13082=CARTESIAN_POINT ( 'NONE',  ( 57.14999999999999858, -3544.570000000000164, 2247.392000000000280 ) ) ;
#13083=EDGE_CURVE ( 'NONE', #20229, #2094, #23001, .T. ) ;
#13086=EDGE_CURVE ( 'NONE', #22481, #12839, #17503, .T. ) ;
#13087=CIRCLE ( 'NONE', #2977, 2.844800000000091700 ) ;
#13088=ORIENTED_EDGE ( 'NONE', *, *, #12436, .T. ) ;
#13089=CARTESIAN_POINT ( 'NONE',  ( 134.8457231033459038, -3662.521201777085935, 2245.835328354021385 ) ) ;
#13090=EDGE_CURVE ( 'NONE', #19652, #12370, #5047, .T. ) ;
#13093=ORIENTED_EDGE ( 'NONE', *, *, #20045, .F. ) ;
#13095=DIRECTION ( 'NONE',  ( 0.000000000000000000, 0.000000000000000000, -1.000000000000000000 ) ) ;
#13097=ADVANCED_FACE ( 'NONE', ( #17619 ), #6741, .F. ) ;
#13100=CIRCLE ( 'NONE', #19070, 3.606799999998994366 ) ;
#13103=DIRECTION ( 'NONE',  ( 0.000000000000000000, 0.000000000000000000, -1.000000000000000000 ) ) ;
#13105=VERTEX_POINT ( 'NONE', #10240 ) ;
#13108=DIRECTION ( 'NONE',  ( -1.000000000000000000, 0.000000000000000000, 0.000000000000000000 ) ) ;
#13112=CARTESIAN_POINT ( 'NONE',  ( 50.79999999999999716, -3619.500000000000000, 2260.600000000000364 ) ) ;
#13113=CARTESIAN_POINT ( 'NONE',  ( 17.81852837919641175, -3662.046892928622128, 2245.280258281285114 ) ) ;
#13115=CARTESIAN_POINT ( 'NONE',  ( 132.0286848278999798, -3544.241664856000170, 2260.557504477000293 ) ) ;
#13116=EDGE_CURVE ( 'NONE', #7066, #7706, #10595, .T. ) ;
#13119=CARTESIAN_POINT ( 'NONE',  ( 141.3710085595040198, -3577.190797867237961, 2249.696701696144373 ) ) ;
#13122=LINE ( 'NONE', #4103, #5809 ) ;
#13126=ORIENTED_EDGE ( 'NONE', *, *, #5118, .F. ) ;
#13127=VERTEX_POINT ( 'NONE', #19500 ) ;
#13131=CARTESIAN_POINT ( 'NONE',  ( 15.31109373216002645, -3578.363233960815251, 2250.193977524520051 ) ) ;
#13133=CARTESIAN_POINT ( 'NONE',  ( 141.5105608045840881, -3581.689302659061013, 2247.699634051008616 ) ) ;
#13138=DIRECTION ( 'NONE',  ( 0.000000000000000000, 1.000000000000000000, 0.000000000000000000 ) ) ;
#13140=ORIENTED_EDGE ( 'NONE', *, *, #896, .T. ) ;
#13141=CARTESIAN_POINT ( 'NONE',  ( 20.68901695980001421, -3543.347945942427032, 2259.675964649152775 ) ) ;
#13142=CIRCLE ( 'NONE', #6426, 2.844799999999009010 ) ;
#13143=CARTESIAN_POINT ( 'NONE',  ( 17.31138602735000021, -3576.119152860999748, 2246.630000000000109 ) ) ;
#13146=CARTESIAN_POINT ( 'NONE',  ( 141.9481709719357525, -3661.250240185189796, 2250.012217711370795 ) ) ;
#13149=EDGE_LOOP ( 'NONE', ( #21277, #7417, #2389, #14874 ) ) ;
#13150=ADVANCED_FACE ( 'NONE', ( #12117 ), #19265, .T. ) ;
#13152=CARTESIAN_POINT ( 'NONE',  ( 57.14999999999999858, -3544.570000000000164, 2247.392000000000280 ) ) ;
#13154=CARTESIAN_POINT ( 'NONE',  ( 88.90000000000000568, -3594.099999999999909, 2260.600000000000364 ) ) ;
#13155=CYLINDRICAL_SURFACE ( 'NONE', #1699, 2.844799999998995244 ) ;
#13156=EDGE_CURVE ( 'NONE', #21069, #20114, #19272, .T. ) ;
#13159=CARTESIAN_POINT ( 'NONE',  ( 7.023553847508563486, -3658.842518250462035, 2244.860302287378090 ) ) ;
#13170=CARTESIAN_POINT ( 'NONE',  ( 137.1599999999999966, -3695.699999999999818, 2255.774000000000342 ) ) ;
#13171=AXIS2_PLACEMENT_3D ( 'NONE', #8902, #340, #14408 ) ;
#13176=CYLINDRICAL_SURFACE ( 'NONE', #20390, 2.844800000000001550 ) ;
#13180=CARTESIAN_POINT ( 'NONE',  ( 20.34169023495000062, -3694.797466901999996, 2260.545675974999995 ) ) ;
#13183=CARTESIAN_POINT ( 'NONE',  ( 25.39999999999999858, -3568.700000000000273, 2259.837999999999738 ) ) ;
#13185=CARTESIAN_POINT ( 'NONE',  ( 151.1299999999999955, -3660.140000000000327, 2247.392000000000280 ) ) ;
#13188=VERTEX_POINT ( 'NONE', #8496 ) ;
#13190=AXIS2_PLACEMENT_3D ( 'NONE', #19797, #20032, #3967 ) ;
#13191=LINE ( 'NONE', #9896, #19517 ) ;
#13196=CARTESIAN_POINT ( 'NONE',  ( 135.0886139726000010, -3662.880847139000252, 2246.630000000000109 ) ) ;
#13197=DIRECTION ( 'NONE',  ( 0.000000000000000000, 0.000000000000000000, 1.000000000000000000 ) ) ;
#13201=CARTESIAN_POINT ( 'NONE',  ( 14.84616252414837945, -3661.372340446721864, 2249.956039958307429 ) ) ;
#13206=CARTESIAN_POINT ( 'NONE',  ( 25.39999999999999858, -3568.700000000000273, 2239.771999999999935 ) ) ;
#13211=EDGE_CURVE ( 'NONE', #3211, #724, #15146, .T. ) ;
#13212=EDGE_LOOP ( 'NONE', ( #13230, #17747, #15350, #20392 ) ) ;
#13213=VECTOR ( 'NONE', #5402, 1000.000000000000000 ) ;
#13223=CARTESIAN_POINT ( 'NONE',  ( 17.91765463811091763, -3661.836797945709804, 2245.108621132138069 ) ) ;
#13224=DIRECTION ( 'NONE',  ( 0.000000000000000000, 0.000000000000000000, -1.000000000000000000 ) ) ;
#13225=CARTESIAN_POINT ( 'NONE',  ( 72.59320000000001016, -3568.700000000000273, 2259.837999999999738 ) ) ;
#13227=ORIENTED_EDGE ( 'NONE', *, *, #4197, .T. ) ;
#13229=DIRECTION ( 'NONE',  ( 0.000000000000000000, 0.000000000000000000, 1.000000000000000000 ) ) ;
#13230=ORIENTED_EDGE ( 'NONE', *, *, #9066, .F. ) ;
#13232=CARTESIAN_POINT ( 'NONE',  ( 15.66193311550068046, -3543.315017895616620, 2254.716481486307202 ) ) ;
#13234=VERTEX_POINT ( 'NONE', #21840 ) ;
#13235=EDGE_CURVE ( 'NONE', #22306, #16307, #18204, .T. ) ;
#13239=EDGE_CURVE ( 'NONE', #572, #16435, #2791, .T. ) ;
#13241=ADVANCED_FACE ( 'NONE', ( #17973 ), #561, .T. ) ;
#13242=DIRECTION ( 'NONE',  ( -1.000000000000000000, 0.000000000000000000, 0.000000000000000000 ) ) ;
#13243=CARTESIAN_POINT ( 'NONE',  ( 15.04722453113185132, -3577.885471855124251, 2250.065661091934544 ) ) ;
#13244=CARTESIAN_POINT ( 'NONE',  ( 141.7948968975624950, -3581.419701962929139, 2248.633431646152076 ) ) ;
#13246=CARTESIAN_POINT ( 'NONE',  ( 151.1299999999999955, -3695.699999999999818, 2240.279999999999745 ) ) ;
#13250=FACE_OUTER_BOUND ( 'NONE', #3751, .T. ) ;
#13251=CARTESIAN_POINT ( 'NONE',  ( 20.34169023495000062, -3544.202533098000458, 2260.545675974999995 ) ) ;
#13253=ADVANCED_FACE ( 'NONE', ( #14697 ), #17769, .T. ) ;
#13254=ORIENTED_EDGE ( 'NONE', *, *, #17458, .F. ) ;
#13260=CIRCLE ( 'NONE', #22608, 2.844800000000001550 ) ;
#13262=AXIS2_PLACEMENT_3D ( 'NONE', #12001, #2976, #6977 ) ;
#13264=ORIENTED_EDGE ( 'NONE', *, *, #9304, .T. ) ;
#13266=DIRECTION ( 'NONE',  ( 1.000000000000000000, 0.000000000000000000, 0.000000000000000000 ) ) ;
#13267=ORIENTED_EDGE ( 'NONE', *, *, #10943, .F. ) ;
#13268=ADVANCED_FACE ( 'NONE', ( #14581 ), #20089, .F. ) ;
#13269=CARTESIAN_POINT ( 'NONE',  ( 7.011289150263468883, -3658.957678416667932, 2244.804336643922852 ) ) ;
#13270=FACE_OUTER_BOUND ( 'NONE', #20020, .T. ) ;
#13275=EDGE_CURVE ( 'NONE', #7984, #473, #7200, .T. ) ;
#13276=CARTESIAN_POINT ( 'NONE',  ( 73.35520000000001062, -3670.300000000000182, 2239.771999999999935 ) ) ;
#13289=LINE ( 'NONE', #11412, #1286 ) ;
#13291=CARTESIAN_POINT ( 'NONE',  ( 18.26100162526913806, -3658.187271764459638, 2245.323245018173566 ) ) ;
#13292=EDGE_LOOP ( 'NONE', ( #327, #9892, #17876, #16302 ) ) ;
#13293=EDGE_LOOP ( 'NONE', ( #10763, #4068, #14535, #8693 ) ) ;
#13296=CARTESIAN_POINT ( 'NONE',  ( 127.0000000000000000, -3670.300000000000182, 2239.771999999999935 ) ) ;
#13297=VECTOR ( 'NONE', #22134, 1000.000000000000000 ) ;
#13300=FACE_OUTER_BOUND ( 'NONE', #8493, .T. ) ;
#13301=AXIS2_PLACEMENT_3D ( 'NONE', #1857, #18362, #557 ) ;
#13304=CYLINDRICAL_SURFACE ( 'NONE', #12836, 1.269999999999882334 ) ;
#13308=ADVANCED_FACE ( 'NONE', ( #17858 ), #1920, .T. ) ;
#13314=B_SPLINE_CURVE_WITH_KNOTS ( 'NONE', 3,
 ( #3682, #12710, #14585, #11181, #2044, #16447, #9194, #21730, #515, #12821, #399, #19977, #21845, #7654, #5686, #5802, #14816, #16222, #12599, #5919, #16110, #14358 ),
 .UNSPECIFIED., .F., .F.,
 ( 4, 2, 2, 1, 2, 2, 2, 1, 2, 2, 2, 4 ),
 ( 0.000000000000000000, 0.1250000000017447987, 0.1875000000025351665, 0.2187500000028428926, 0.2343750000029967695, 0.2500000000031506464, 0.3750000000040985548, 0.4375000000042824078, 0.4687500000042232329, 0.5000000000041640025, 0.7500000000020820012, 1.000000000000000000 ),
 .UNSPECIFIED. ) ;
#13315=ORIENTED_EDGE ( 'NONE', *, *, #6085, .F. ) ;
#13317=FACE_BOUND ( 'NONE', #3491, .T. ) ;
#13320=CARTESIAN_POINT ( 'NONE',  ( 134.1946444147164925, -3577.961207644249043, 2244.692860678807392 ) ) ;
#13321=ORIENTED_EDGE ( 'NONE', *, *, #1346, .T. ) ;
#13324=CYLINDRICAL_SURFACE ( 'NONE', #19301, 0.7619999999999294005 ) ;
#13326=CIRCLE ( 'NONE', #4398, 2.844799999998842033 ) ;
#13327=ORIENTED_EDGE ( 'NONE', *, *, #8095, .F. ) ;
#13331=CARTESIAN_POINT ( 'NONE',  ( 38.10000000000000142, -3644.899999999999636, 2239.771999999999935 ) ) ;
#13334=AXIS2_PLACEMENT_3D ( 'NONE', #18116, #14500, #21641 ) ;
#13339=ORIENTED_EDGE ( 'NONE', *, *, #13388, .T. ) ;
#13344=CARTESIAN_POINT ( 'NONE',  ( 15.24000000000000021, -3694.430000000000291, 2255.774000000000342 ) ) ;
#13347=DIRECTION ( 'NONE',  ( 0.000000000000000000, 0.000000000000000000, -1.000000000000000000 ) ) ;
#13350=TOROIDAL_SURFACE ( 'NONE', #21228, 3.606799999999999784, 0.7620000000000000107 ) ;
#13351=DIRECTION ( 'NONE',  ( 0.000000000000000000, 0.000000000000000000, -1.000000000000000000 ) ) ;
#13352=VERTEX_POINT ( 'NONE', #10826 ) ;
#13353=DIRECTION ( 'NONE',  ( 0.000000000000000000, -1.000000000000000000, 0.000000000000000000 ) ) ;
#13354=CIRCLE ( 'NONE', #21952, 0.7619999999999294005 ) ;
#13357=ORIENTED_EDGE ( 'NONE', *, *, #516, .F. ) ;
#13359=AXIS2_PLACEMENT_3D ( 'NONE', #3235, #17523, #15779 ) ;
#13360=EDGE_LOOP ( 'NONE', ( #9496, #7282, #19193, #5286, #2495, #4240, #11636, #8373 ) ) ;
#13364=CARTESIAN_POINT ( 'NONE',  ( 11.80730815183341420, -3576.792673990085859, 2249.346535258006043 ) ) ;
#13366=CARTESIAN_POINT ( 'NONE',  ( 141.7296139770200512, -3581.488818245647053, 2248.480571682398477 ) ) ;
#13373=DIRECTION ( 'NONE',  ( 0.000000000000000000, -1.000000000000000000, 0.000000000000000000 ) ) ;
#13374=CARTESIAN_POINT ( 'NONE',  ( 131.5729205195000020, -3543.299999999999727, 2259.329999999999927 ) ) ;
#13378=EDGE_CURVE ( 'NONE', #11527, #12156, #18886, .T. ) ;
#13380=CARTESIAN_POINT ( 'NONE',  ( 50.79999999999999716, -3670.300000000000182, 2239.771999999999935 ) ) ;
#13381=EDGE_CURVE ( 'NONE', #16324, #7211, #5437, .T. ) ;
#13382=ORIENTED_EDGE ( 'NONE', *, *, #14973, .F. ) ;
#13385=CIRCLE ( 'NONE', #17889, 2.844799999998998796 ) ;
#13386=DIRECTION ( 'NONE',  ( 0.000000000000000000, 0.000000000000000000, -1.000000000000000000 ) ) ;
#13387=EDGE_LOOP ( 'NONE', ( #21507, #21892 ) ) ;
#13388=EDGE_CURVE ( 'NONE', #19496, #16546, #21529, .T. ) ;
#13395=ADVANCED_FACE ( 'NONE', ( #9525 ), #18522, .T. ) ;
#13401=CARTESIAN_POINT ( 'NONE',  ( 133.9850000806000025, -3659.504501929000071, 2244.618659328000376 ) ) ;
#13402=AXIS2_PLACEMENT_3D ( 'NONE', #14101, #20901, #13756 ) ;
#13405=CARTESIAN_POINT ( 'NONE',  ( 136.9962324742510305, -3543.632335308055644, 2255.363864800105603 ) ) ;
#13406=EDGE_CURVE ( 'NONE', #10444, #4163, #6560, .T. ) ;
#13407=EDGE_LOOP ( 'NONE', ( #7852, #16698, #10476, #8580 ) ) ;
#13411=CARTESIAN_POINT ( 'NONE',  ( 18.41519309055000164, -3659.504912144000173, 2244.618989493999834 ) ) ;
#13413=ORIENTED_EDGE ( 'NONE', *, *, #9487, .T. ) ;
#13414=DIRECTION ( 'NONE',  ( 1.000000000000000000, 0.000000000000000000, 0.000000000000000000 ) ) ;
#13417=CARTESIAN_POINT ( 'NONE',  ( 9.855200000000998273, -3579.494999999999891, 2256.063560000000052 ) ) ;
#13419=AXIS2_PLACEMENT_3D ( 'NONE', #8636, #17410, #8530 ) ;
#13420=CARTESIAN_POINT ( 'NONE',  ( 20.68889176940725605, -3695.652054061570652, 2259.675914647556056 ) ) ;
#13421=ORIENTED_EDGE ( 'NONE', *, *, #9265, .T. ) ;
#13423=CARTESIAN_POINT ( 'NONE',  ( 145.2144692705681450, -3658.007655502538455, 2245.504405415671954 ) ) ;
#13424=ADVANCED_FACE ( 'NONE', ( #6256 ), #13155, .F. ) ;
#13425=CARTESIAN_POINT ( 'NONE',  ( 9.908383082390907148, -3580.044228178761841, 2249.978629610284770 ) ) ;
#13427=ORIENTED_EDGE ( 'NONE', *, *, #5806, .T. ) ;
#13428=DIRECTION ( 'NONE',  ( 0.000000000000000000, 0.000000000000000000, -1.000000000000000000 ) ) ;
#13430=CARTESIAN_POINT ( 'NONE',  ( 145.1820664649105765, -3661.120306023109606, 2244.721041474187587 ) ) ;
#13434=CARTESIAN_POINT ( 'NONE',  ( 15.39811514000335713, -3660.419159658365061, 2250.226394777855148 ) ) ;
#13435=ADVANCED_FACE ( 'NONE', ( #4254 ), #16783, .F. ) ;
#13438=EDGE_CURVE ( 'NONE', #19601, #13554, #21163, .T. ) ;
#13442=CARTESIAN_POINT ( 'NONE',  ( 15.46655083684568055, -3658.835041740453107, 2249.921457276668207 ) ) ;
#13448=ORIENTED_EDGE ( 'NONE', *, *, #8843, .T. ) ;
#13451=CARTESIAN_POINT ( 'NONE',  ( 145.1237722701461337, -3581.296112608482872, 2245.922901420255130 ) ) ;
#13453=EDGE_CURVE ( 'NONE', #825, #11149, #1318, .T. ) ;
#13455=DIRECTION ( 'NONE',  ( 0.000000000000000000, 0.000000000000000000, -1.000000000000000000 ) ) ;
#13456=CARTESIAN_POINT ( 'NONE',  ( 18.13280299816700136, -3661.283447638940288, 2244.782395619060026 ) ) ;
#13458=DIRECTION ( 'NONE',  ( -1.000000000000000000, 0.000000000000000000, 0.000000000000000000 ) ) ;
#13464=ORIENTED_EDGE ( 'NONE', *, *, #526, .F. ) ;
#13467=CARTESIAN_POINT ( 'NONE',  ( 10.90866455802274082, -3657.294969492509153, 2247.463672662353474 ) ) ;
#13469=ORIENTED_EDGE ( 'NONE', *, *, #19387, .T. ) ;
#13472=VERTEX_POINT ( 'NONE', #21946 ) ;
#13475=CARTESIAN_POINT ( 'NONE',  ( 141.5633583212279234, -3581.644791717248609, 2247.976212405268598 ) ) ;
#13476=ORIENTED_EDGE ( 'NONE', *, *, #1779, .F. ) ;
#13477=LINE ( 'NONE', #13246, #18602 ) ;
#13482=DIRECTION ( 'NONE',  ( -1.000000000000000000, -1.202995631304000193E-14, 0.000000000000000000 ) ) ;
#13484=DIRECTION ( 'NONE',  ( -1.000000000000000000, 0.000000000000000000, 0.000000000000000000 ) ) ;
#13506=DIRECTION ( 'NONE',  ( 0.000000000000000000, 0.000000000000000000, 1.000000000000000000 ) ) ;
#13509=CARTESIAN_POINT ( 'NONE',  ( 141.8306442670041179, -3657.619971841161714, 2248.712053168803322 ) ) ;
#13514=CARTESIAN_POINT ( 'NONE',  ( 137.0287686657979407, -3543.717426572939530, 2255.445352725414068 ) ) ;
#13516=ORIENTED_EDGE ( 'NONE', *, *, #409, .F. ) ;
#13517=EDGE_CURVE ( 'NONE', #3735, #17090, #21172, .T. ) ;
#13518=ORIENTED_EDGE ( 'NONE', *, *, #6651, .F. ) ;
#13521=CIRCLE ( 'NONE', #4915, 3.606799999998994366 ) ;
#13525=FACE_OUTER_BOUND ( 'NONE', #14287, .T. ) ;
#13527=CARTESIAN_POINT ( 'NONE',  ( 35.56000000000000227, -3568.700000000000273, 2244.547199999999975 ) ) ;
#13529=CARTESIAN_POINT ( 'NONE',  ( 101.5999999999999943, -3670.300000000000182, 2239.771999999999935 ) ) ;
#13531=CARTESIAN_POINT ( 'NONE',  ( 17.85473721720958551, -3577.030903703768217, 2245.207284487792549 ) ) ;
#13533=CARTESIAN_POINT ( 'NONE',  ( 134.3871257470999865, -3581.600847139000052, 2246.630000000000109 ) ) ;
#13541=TOROIDAL_SURFACE ( 'NONE', #14677, 3.606799999998999695, 0.7620000000000000107 ) ;
#13542=CARTESIAN_POINT ( 'NONE',  ( 9.877889775156498686, -3579.858006066903272, 2250.056460527199306 ) ) ;
#13545=CYLINDRICAL_SURFACE ( 'NONE', #3218, 2.844799999998998796 ) ;
#13549=ORIENTED_EDGE ( 'NONE', *, *, #8556, .T. ) ;
#13550=DIRECTION ( 'NONE',  ( 0.8928571428573600643, -0.4503400076038009403, 0.000000000000000000 ) ) ;
#13554=VERTEX_POINT ( 'NONE', #19125 ) ;
#13556=B_SPLINE_CURVE_WITH_KNOTS ( 'NONE', 3,
 ( #18838, #15795, #13921, #8299, #4657, #14039, #17541, #21070, #1486, #22921, #18962, #2906, #15444, #10164, #17304, #8414, #5606, #12630, #7241, #16028, #3596, #21538, #23044, #10754 ),
 .UNSPECIFIED., .F., .F.,
 ( 4, 2, 2, 1, 1, 1, 2, 2, 2, 2, 1, 2, 2, 4 ),
 ( 0.000000000000000000, 0.1249999999954432839, 0.1874999999933733841, 0.2187499999923384342, 0.2343749999923080418, 0.2421874999926629524, 0.2460937499926816874, 0.2499999999927004501, 0.3749999999974015785, 0.4374999999999966138, 0.4687500000008462120, 0.4843750000012573276, 0.5000000000016684432, 1.000000000000000000 ),
 .UNSPECIFIED. ) ;
#13562=CARTESIAN_POINT ( 'NONE',  ( 15.52417949512691386, -3659.157734418582550, 2250.062346885889838 ) ) ;
#13564=ORIENTED_EDGE ( 'NONE', *, *, #14409, .F. ) ;
#13566=ORIENTED_EDGE ( 'NONE', *, *, #7701, .T. ) ;
#13568=ORIENTED_EDGE ( 'NONE', *, *, #2158, .F. ) ;
#13572=EDGE_CURVE ( 'NONE', #10769, #20632, #5061, .T. ) ;
#13573=DIRECTION ( 'NONE',  ( 1.000000000000000000, 0.000000000000000000, 0.000000000000000000 ) ) ;
#13575=CARTESIAN_POINT ( 'NONE',  ( 105.2067999999999870, -3619.500000000000000, 2260.600000000000364 ) ) ;
#13582=DIRECTION ( 'NONE',  ( 0.000000000000000000, 0.000000000000000000, -1.000000000000000000 ) ) ;
#13583=EDGE_CURVE ( 'NONE', #4126, #5555, #19284, .T. ) ;
#13585=CARTESIAN_POINT ( 'NONE',  ( 7.387125747152000876, -3657.399152860999493, 2246.630000000000109 ) ) ;
#13586=CYLINDRICAL_SURFACE ( 'NONE', #14436, 2.844799999998995244 ) ;
#13587=ORIENTED_EDGE ( 'NONE', *, *, #19543, .F. ) ;
#13588=LINE ( 'NONE', #20853, #8809 ) ;
#13589=CARTESIAN_POINT ( 'NONE',  ( 10.23711275231256579, -3658.078120033774667, 2249.355894016820912 ) ) ;
#13590=EDGE_CURVE ( 'NONE', #17865, #553, #10679, .T. ) ;
#13592=ADVANCED_FACE ( 'NONE', ( #14090 ), #5189, .F. ) ;
#13593=ORIENTED_EDGE ( 'NONE', *, *, #13869, .T. ) ;
#13594=CARTESIAN_POINT ( 'NONE',  ( 134.2318573182560897, -3581.156156794382241, 2245.707491121732346 ) ) ;
#13595=EDGE_LOOP ( 'NONE', ( #21491, #14220, #18954, #12328 ) ) ;
#13598=DIRECTION ( 'NONE',  ( -0.000000000000000000, -1.000000000000000000, -0.000000000000000000 ) ) ;
#13600=CARTESIAN_POINT ( 'NONE',  ( 142.0697870230637818, -3581.068730170725303, 2249.184906718528509 ) ) ;
#13606=CARTESIAN_POINT ( 'NONE',  ( 20.82707948048999924, -3543.299999999999727, 2259.329999999999927 ) ) ;
#13608=CARTESIAN_POINT ( 'NONE',  ( 134.1359104811938892, -3658.200395526626835, 2245.310932276000585 ) ) ;
#13609=EDGE_LOOP ( 'NONE', ( #15474, #5382, #19771, #9799 ) ) ;
#13611=AXIS2_PLACEMENT_3D ( 'NONE', #7746, #14898, #22025 ) ;
#13615=EDGE_LOOP ( 'NONE', ( #23098, #21181, #5297, #20263, #12803, #499 ) ) ;
#13618=TOROIDAL_SURFACE ( 'NONE', #2752, 3.606799999998999695, 0.7620000000000000107 ) ;
#13623=CARTESIAN_POINT ( 'NONE',  ( 63.50000000000000000, -3594.099999999999909, 2239.771999999999935 ) ) ;
#13625=LINE ( 'NONE', #19254, #8076 ) ;
#13626=DIRECTION ( 'NONE',  ( 0.000000000000000000, 0.000000000000000000, -1.000000000000000000 ) ) ;
#13627=DIRECTION ( 'NONE',  ( 1.000000000000000000, 0.000000000000000000, 0.000000000000000000 ) ) ;
#13629=CARTESIAN_POINT ( 'NONE',  ( 141.4907929136770690, -3657.294513356050174, 2247.445207560118433 ) ) ;
#13633=CARTESIAN_POINT ( 'NONE',  ( 137.1599999998475425, -3544.490134410746577, 2255.773999999840271 ) ) ;
#13634=AXIS2_PLACEMENT_3D ( 'NONE', #10738, #17883, #1828 ) ;
#13638=DIRECTION ( 'NONE',  ( -1.000000000000000000, 0.000000000000000000, 0.000000000000000000 ) ) ;
#13639=EDGE_CURVE ( 'NONE', #2680, #2712, #3940, .T. ) ;
#13641=ORIENTED_EDGE ( 'NONE', *, *, #14366, .T. ) ;
#13644=DIRECTION ( 'NONE',  ( 0.000000000000000000, 0.000000000000000000, -1.000000000000000000 ) ) ;
#13646=VERTEX_POINT ( 'NONE', #7404 ) ;
#13647=CARTESIAN_POINT ( 'NONE',  ( 25.39999999999999858, -3660.140000000000327, 2247.392000000000280 ) ) ;
#13648=CARTESIAN_POINT ( 'NONE',  ( 139.6999999999999886, -3579.494999999999891, 2239.009999999999764 ) ) ;
#13650=AXIS2_PLACEMENT_3D ( 'NONE', #5937, #17149, #4279 ) ;
#13651=CARTESIAN_POINT ( 'NONE',  ( 35.56000000000000227, -3670.300000000000182, 2247.392000000000280 ) ) ;
#13652=CIRCLE ( 'NONE', #3544, 2.844800000000091700 ) ;
#13654=EDGE_LOOP ( 'NONE', ( #20546, #13059, #17269, #9200, #8785, #10805 ) ) ;
#13660=CARTESIAN_POINT ( 'NONE',  ( 10.79725788089033855, -3581.609851679345411, 2248.121171040608260 ) ) ;
#13662=VERTEX_POINT ( 'NONE', #14555 ) ;
#13665=B_SPLINE_CURVE_WITH_KNOTS ( 'NONE', 3,
 ( #10966, #14496, #16357, #3929, #19879, #2185, #11195, #310, #16241, #19770, #7342, #9331, #20115, #3811, #16466, #14724, #4049, #19640, #17885, #8979, #16127, #75, #2405, #16696, #13291, #18909, #11304, #17030, #747, #4162, #648, #15060, #18455, #11633, #2861, #4498, #15287, #18791, #13411 ),
 .UNSPECIFIED., .F., .F.,
 ( 4, 2, 2, 1, 1, 1, 2, 2, 2, 2, 2, 2, 1, 1, 2, 2, 2, 2, 1, 1, 2, 2, 4 ),
 ( 0.000000000000000000, 0.1250000000158134339, 0.1875000000236058673, 0.2187500000277668721, 0.2343750000298476244, 0.2421875000311433102, 0.2460937500318851334, 0.2500000000326269567, 0.3125000000339349104, 0.3750000000352428087, 0.4375000000365507624, 0.4687500000372124553, 0.4843750000373662767, 0.4921875000372503139, 0.4960937500371923048, 0.5000000000371342956, 0.6250000000314543946, 0.6875000000287884161, 0.7187500000274557044, 0.7343750000266703326, 0.7421875000260601540, 0.7500000000254499755, 1.000000000000000000 ),
 .UNSPECIFIED. ) ;
#13667=CARTESIAN_POINT ( 'NONE',  ( 145.1350961731654365, -3661.271952279658763, 2244.781081194931630 ) ) ;
#13674=AXIS2_PLACEMENT_3D ( 'NONE', #21241, #15376, #21001 ) ;
#13676=FACE_OUTER_BOUND ( 'NONE', #23114, .T. ) ;
#13678=CARTESIAN_POINT ( 'NONE',  ( 104.4447999999999865, -3670.300000000000182, 2259.837999999999738 ) ) ;
#13679=CARTESIAN_POINT ( 'NONE',  ( 15.54478936534684941, -3659.505023738319323, 2250.165136749944850 ) ) ;
#13681=VERTEX_POINT ( 'NONE', #9280 ) ;
#13682=EDGE_CURVE ( 'NONE', #10278, #13993, #1652, .T. ) ;
#13683=EDGE_LOOP ( 'NONE', ( #17707, #12301, #1670, #8351 ) ) ;
#13684=CARTESIAN_POINT ( 'NONE',  ( 116.8400000000000034, -3695.699999999999818, 2243.277199999999993 ) ) ;
#13685=EDGE_CURVE ( 'NONE', #12882, #20359, #12442, .T. ) ;
#13693=AXIS2_PLACEMENT_3D ( 'NONE', #10878, #15316, #22213 ) ;
#13694=DIRECTION ( 'NONE',  ( -0.000000000000000000, -1.000000000000000000, -0.000000000000000000 ) ) ;
#13699=CARTESIAN_POINT ( 'NONE',  ( 137.5031457249828577, -3577.685606708022533, 2249.984038353326014 ) ) ;
#13701=DIRECTION ( 'NONE',  ( 0.000000000000000000, 0.000000000000000000, -1.000000000000000000 ) ) ;
#13707=DIRECTION ( 'NONE',  ( 0.000000000000000000, 0.000000000000000000, -1.000000000000000000 ) ) ;
#13711=AXIS2_PLACEMENT_3D ( 'NONE', #58, #12708, #9077 ) ;
#13714=CARTESIAN_POINT ( 'NONE',  ( 123.3932000000010021, -3670.300000000000182, 2259.837999999999738 ) ) ;
#13721=CARTESIAN_POINT ( 'NONE',  ( 15.74707948048999917, -3543.299999999999727, 2254.503999999999905 ) ) ;
#13723=CARTESIAN_POINT ( 'NONE',  ( 131.7496328904776988, -3695.620464488476500, 2259.772527316505148 ) ) ;
#13726=CARTESIAN_POINT ( 'NONE',  ( 14.61268103042000099, -3581.600842893000390, 2246.630000000000109 ) ) ;
#13728=CARTESIAN_POINT ( 'NONE',  ( 134.2666750161357072, -3657.732842303892539, 2245.875864816541252 ) ) ;
#13730=ORIENTED_EDGE ( 'NONE', *, *, #1463, .F. ) ;
#13731=CIRCLE ( 'NONE', #12981, 2.844799999998998796 ) ;
#13732=CARTESIAN_POINT ( 'NONE',  ( 15.51380746874810335, -3695.561367820956548, 2255.088321283119967 ) ) ;
#13736=ORIENTED_EDGE ( 'NONE', *, *, #5992, .T. ) ;
#13738=EDGE_CURVE ( 'NONE', #7229, #12882, #19665, .T. ) ;
#13739=DIRECTION ( 'NONE',  ( 0.000000000000000000, 0.000000000000000000, -1.000000000000000000 ) ) ;
#13740=EDGE_LOOP ( 'NONE', ( #1006, #9727 ) ) ;
#13741=ORIENTED_EDGE ( 'NONE', *, *, #22969, .T. ) ;
#13743=DIRECTION ( 'NONE',  ( 0.000000000000000000, -1.000000000000000000, 0.000000000000000000 ) ) ;
#13744=AXIS2_PLACEMENT_3D ( 'NONE', #3511, #123, #3980 ) ;
#13745=ORIENTED_EDGE ( 'NONE', *, *, #17387, .T. ) ;
#13746=AXIS2_PLACEMENT_3D ( 'NONE', #9047, #9288, #4009 ) ;
#13747=PLANE ( 'NONE',  #3102 ) ;
#13750=FACE_OUTER_BOUND ( 'NONE', #7378, .T. ) ;
#13751=CARTESIAN_POINT ( 'NONE',  ( 136.9269754645999910, -3578.860002036999958, 2250.236803302000226 ) ) ;
#13755=CARTESIAN_POINT ( 'NONE',  ( 14.61268103042000099, -3581.600842893000390, 2246.630000000000109 ) ) ;
#13756=DIRECTION ( 'NONE',  ( -1.000000000000000000, 0.000000000000000000, 0.000000000000000000 ) ) ;
#13758=CARTESIAN_POINT ( 'NONE',  ( 142.1353304486877391, -3658.034425628051395, 2249.305387334696661 ) ) ;
#13759=VERTEX_POINT ( 'NONE', #17706 ) ;
#13760=CARTESIAN_POINT ( 'NONE',  ( 136.8684679650089038, -3543.420329759140259, 2255.043779574668406 ) ) ;
#13765=VECTOR ( 'NONE', #19759, 1000.000000000000000 ) ;
#13766=DIRECTION ( 'NONE',  ( 0.000000000000000000, 0.000000000000000000, 1.000000000000000000 ) ) ;
#13768=ORIENTED_EDGE ( 'NONE', *, *, #16938, .F. ) ;
#13769=CARTESIAN_POINT ( 'NONE',  ( 4.743095773629126377, -3543.373434456934774, 2259.755879528988771 ) ) ;
#13770=CARTESIAN_POINT ( 'NONE',  ( 76.20000000000000284, -3670.300000000000182, 2260.600000000000364 ) ) ;
#13775=DIRECTION ( 'NONE',  ( -0.8928571428563427670, 0.4503400076058181045, 0.000000000000000000 ) ) ;
#13779=ORIENTED_EDGE ( 'NONE', *, *, #18021, .F. ) ;
#13784=CARTESIAN_POINT ( 'NONE',  ( 10.79145926739417760, -3581.604639450296872, 2248.140541687839232 ) ) ;
#13786=DIRECTION ( 'NONE',  ( 0.000000000000000000, 0.000000000000000000, 1.000000000000000000 ) ) ;
#13787=VERTEX_POINT ( 'NONE', #19592 ) ;
#13788=DIRECTION ( 'NONE',  ( -1.000000000000000000, 0.000000000000000000, 0.000000000000000000 ) ) ;
#13792=CARTESIAN_POINT ( 'NONE',  ( 11.20651475058533464, -3661.926271786974212, 2249.606089457644430 ) ) ;
#13793=CARTESIAN_POINT ( 'NONE',  ( 147.4346858863133320, -3543.765301129279123, 2260.312744311644565 ) ) ;
#13799=CARTESIAN_POINT ( 'NONE',  ( 136.8551930556999991, -3659.717490576542787, 2250.213681781542618 ) ) ;
#13800=CARTESIAN_POINT ( 'NONE',  ( 14.61266695128000137, -3657.399152860999493, 2246.630000000000109 ) ) ;
#13822=CARTESIAN_POINT ( 'NONE',  ( 101.5999999999999943, -3670.300000000000182, 2259.837999999999738 ) ) ;
#13823=VERTEX_POINT ( 'NONE', #18951 ) ;
#13825=DIRECTION ( 'NONE',  ( -1.000000000000000000, 0.000000000000000000, 0.000000000000000000 ) ) ;
#13826=CARTESIAN_POINT ( 'NONE',  ( 151.1299999999999955, -3578.860000000000127, 2250.236800000000130 ) ) ;
#13831=DIRECTION ( 'NONE',  ( -1.000000000000000000, 0.000000000000000000, 0.000000000000000000 ) ) ;
#13832=CARTESIAN_POINT ( 'NONE',  ( 21.19471181662999726, -3544.570000000000164, 2259.679250718999810 ) ) ;
#13839=FACE_OUTER_BOUND ( 'NONE', #19374, .T. ) ;
#13840=AXIS2_PLACEMENT_3D ( 'NONE', #21449, #5397, #14419 ) ;
#13841=CARTESIAN_POINT ( 'NONE',  ( 134.1558484328602390, -3658.117549335799595, 2245.390303089542158 ) ) ;
#13846=CARTESIAN_POINT ( 'NONE',  ( 15.66246403760665196, -3695.684982104464325, 2254.716693470072187 ) ) ;
#13848=CYLINDRICAL_SURFACE ( 'NONE', #18823, 2.844800000000091700 ) ;
#13849=CARTESIAN_POINT ( 'NONE',  ( 15.54479999999999862, -3579.494999999999891, 2256.063560000000052 ) ) ;
#13850=VERTEX_POINT ( 'NONE', #8176 ) ;
#13854=ORIENTED_EDGE ( 'NONE', *, *, #16885, .F. ) ;
#13856=CARTESIAN_POINT ( 'NONE',  ( 135.5205281809360827, -3657.399153614157967, 2246.629997290541269 ) ) ;
#13860=CARTESIAN_POINT ( 'NONE',  ( 50.79999999999999716, -3619.500000000000000, 2239.009999999999764 ) ) ;
#13863=DIRECTION ( 'NONE',  ( -1.000000000000000000, 0.000000000000000000, 0.000000000000000000 ) ) ;
#13865=B_SPLINE_CURVE_WITH_KNOTS ( 'NONE', 3,
 ( #316, #12623, #10745, #19530 ),
 .UNSPECIFIED., .F., .F.,
 ( 4, 4 ),
 ( 0.000000000000000000, 1.000000000000000000 ),
 .UNSPECIFIED. ) ;
#13867=CARTESIAN_POINT ( 'NONE',  ( 142.1532463573187215, -3658.064754788580103, 2249.338046269550887 ) ) ;
#13869=EDGE_CURVE ( 'NONE', #10418, #7999, #3565, .T. ) ;
#13870=ORIENTED_EDGE ( 'NONE', *, *, #4840, .F. ) ;
#13871=DIRECTION ( 'NONE',  ( -1.000000000000000000, 0.000000000000000000, 0.000000000000000000 ) ) ;
#13872=ORIENTED_EDGE ( 'NONE', *, *, #18195, .F. ) ;
#13874=EDGE_CURVE ( 'NONE', #12370, #2712, #19568, .T. ) ;
#13876=ORIENTED_EDGE ( 'NONE', *, *, #15138, .F. ) ;
#13878=VERTEX_POINT ( 'NONE', #4533 ) ;
#13880=DIRECTION ( 'NONE',  ( 0.000000000000000000, 0.000000000000000000, 1.000000000000000000 ) ) ;
#13883=EDGE_CURVE ( 'NONE', #6665, #5168, #2724, .T. ) ;
#13885=AXIS2_PLACEMENT_3D ( 'NONE', #8148, #8257, #22534 ) ;
#13886=CARTESIAN_POINT ( 'NONE',  ( 57.14999999999999858, -3694.430000000000291, 2244.547199999999975 ) ) ;
#13889=CARTESIAN_POINT ( 'NONE',  ( 101.5999999999999943, -3619.500000000000000, 2239.771999999999935 ) ) ;
#13892=ORIENTED_EDGE ( 'NONE', *, *, #17383, .T. ) ;
#13894=ORIENTED_EDGE ( 'NONE', *, *, #5272, .T. ) ;
#13895=DIRECTION ( 'NONE',  ( 0.000000000000000000, 0.000000000000000000, -1.000000000000000000 ) ) ;
#13897=DIRECTION ( 'NONE',  ( 0.000000000000000000, 0.000000000000000000, -1.000000000000000000 ) ) ;
#13901=AXIS2_PLACEMENT_3D ( 'NONE', #9343, #19892, #18126 ) ;
#13902=FACE_BOUND ( 'NONE', #19378, .T. ) ;
#13904=CARTESIAN_POINT ( 'NONE',  ( 29.00679999999900005, -3670.300000000000182, 2239.771999999999935 ) ) ;
#13905=CARTESIAN_POINT ( 'NONE',  ( 144.4335724592128258, -3662.708189880353530, 2246.166055327533286 ) ) ;
#13906=DIRECTION ( 'NONE',  ( -1.000000000000000000, 0.000000000000000000, 0.000000000000000000 ) ) ;
#13907=CARTESIAN_POINT ( 'NONE',  ( 10.99177528568289830, -3661.779950359641589, 2249.716450903262285 ) ) ;
#13908=CARTESIAN_POINT ( 'NONE',  ( 147.4191137077191627, -3543.814512432531501, 2260.351687526631849 ) ) ;
#13912=DIRECTION ( 'NONE',  ( 0.000000000000000000, 1.000000000000000000, 0.000000000000000000 ) ) ;
#13914=FACE_OUTER_BOUND ( 'NONE', #20705, .T. ) ;
#13916=TOROIDAL_SURFACE ( 'NONE', #18410, 3.606799999999999784, 0.7620000000000000107 ) ;
#13917=ORIENTED_EDGE ( 'NONE', *, *, #3504, .T. ) ;
#13918=AXIS2_PLACEMENT_3D ( 'NONE', #15588, #22723, #15701 ) ;
#13919=DIRECTION ( 'NONE',  ( 0.000000000000000000, 0.000000000000000000, 1.000000000000000000 ) ) ;
#13921=CARTESIAN_POINT ( 'NONE',  ( 9.737535961660340078, -3543.315017895228266, 2254.716693468255016 ) ) ;
#13923=CARTESIAN_POINT ( 'NONE',  ( 134.3871257472000025, -3657.399152860999493, 2246.630000000000109 ) ) ;
#13926=AXIS2_PLACEMENT_3D ( 'NONE', #6175, #4516, #8162 ) ;
#13931=DIRECTION ( 'NONE',  ( 0.000000000000000000, 0.000000000000000000, -1.000000000000000000 ) ) ;
#13932=ORIENTED_EDGE ( 'NONE', *, *, #13378, .T. ) ;
#13933=CIRCLE ( 'NONE', #19554, 0.7619999999999987894 ) ;
#13938=ORIENTED_EDGE ( 'NONE', *, *, #8593, .F. ) ;
#13939=CARTESIAN_POINT ( 'NONE',  ( 9.926995637850000165, -3660.140002548000211, 2250.236801297000056 ) ) ;
#13940=CARTESIAN_POINT ( 'NONE',  ( 10.80609603922892070, -3657.382216624303055, 2248.090589125378301 ) ) ;
#13941=EDGE_CURVE ( 'NONE', #14116, #15892, #3244, .T. ) ;
#13942=EDGE_LOOP ( 'NONE', ( #596, #1072, #21481, #397 ) ) ;
#13943=CARTESIAN_POINT ( 'NONE',  ( 132.2768405780999785, -3694.472271328999796, 2260.413001451000127 ) ) ;
#13944=CIRCLE ( 'NONE', #16919, 0.7619999999999294005 ) ;
#13948=DIRECTION ( 'NONE',  ( -0.7249994335944509594, 0.000000000000000000, 0.6887494619146539154 ) ) ;
#13950=CARTESIAN_POINT ( 'NONE',  ( 131.7385023306979406, -3695.630398139015142, 2259.744659233807397 ) ) ;
#13954=CARTESIAN_POINT ( 'NONE',  ( 15.11849031972590041, -3580.993088984551378, 2249.274435424331841 ) ) ;
#13955=CARTESIAN_POINT ( 'NONE',  ( 134.0922626992376081, -3658.402569313454933, 2245.138333345573756 ) ) ;
#13957=ORIENTED_EDGE ( 'NONE', *, *, #22733, .T. ) ;
#13958=AXIS2_PLACEMENT_3D ( 'NONE', #13225, #7845, #20159 ) ;
#13959=CARTESIAN_POINT ( 'NONE',  ( 142.2400000000000091, -3544.570000000000164, 2255.774000000000342 ) ) ;
#13960=EDGE_CURVE ( 'NONE', #20359, #13759, #12827, .T. ) ;
#13963=ADVANCED_FACE ( 'NONE', ( #317 ), #3098, .T. ) ;
#13964=FACE_OUTER_BOUND ( 'NONE', #2920, .T. ) ;
#13965=AXIS2_PLACEMENT_3D ( 'NONE', #17481, #5070, #22631 ) ;
#13966=EDGE_CURVE ( 'NONE', #7066, #19732, #216, .T. ) ;
#13967=ADVANCED_FACE ( 'NONE', ( #10974 ), #10207, .T. ) ;
#13970=EDGE_LOOP ( 'NONE', ( #7750, #11156, #17850, #17084 ) ) ;
#13974=EDGE_LOOP ( 'NONE', ( #10257, #11443 ) ) ;
#13975=FACE_BOUND ( 'NONE', #20336, .T. ) ;
#13976=CARTESIAN_POINT ( 'NONE',  ( 15.52082456645615238, -3659.877973396570724, 2250.225202194340000 ) ) ;
#13977=LINE ( 'NONE', #22981, #18588 ) ;
#13981=CARTESIAN_POINT ( 'NONE',  ( 6.985153502415999860, -3659.505556594000154, 2244.618656866000038 ) ) ;
#13982=DIRECTION ( 'NONE',  ( -1.000000000000000000, 0.000000000000000000, 0.000000000000000000 ) ) ;
#13983=CARTESIAN_POINT ( 'NONE',  ( 18.37871628331206608, -3580.137931053087868, 2244.850299910469857 ) ) ;
#13987=CARTESIAN_POINT ( 'NONE',  ( 141.4997331193342518, -3657.301708037173285, 2247.198575533412622 ) ) ;
#13988=VERTEX_POINT ( 'NONE', #14502 ) ;
#13991=ORIENTED_EDGE ( 'NONE', *, *, #16709, .F. ) ;
#13992=ORIENTED_EDGE ( 'NONE', *, *, #3070, .F. ) ;
#13993=VERTEX_POINT ( 'NONE', #16364 ) ;
#13997=VERTEX_POINT ( 'NONE', #11095 ) ;
#13998=ORIENTED_EDGE ( 'NONE', *, *, #16267, .F. ) ;
#13999=CARTESIAN_POINT ( 'NONE',  ( 4.618254035402077129, -3543.300000000021555, 2259.443539528608198 ) ) ;
#14001=DIRECTION ( 'NONE',  ( 1.000000000000000000, 0.000000000000000000, 0.000000000000000000 ) ) ;
#14003=ADVANCED_FACE ( 'NONE', ( #9338 ), #539, .F. ) ;
#14007=FACE_BOUND ( 'NONE', #11326, .T. ) ;
#14009=DIRECTION ( 'NONE',  ( 1.000000000000000000, 0.000000000000000000, 0.000000000000000000 ) ) ;
#14012=ORIENTED_EDGE ( 'NONE', *, *, #14688, .T. ) ;
#14013=EDGE_CURVE ( 'NONE', #650, #9827, #2302, .T. ) ;
#14015=CARTESIAN_POINT ( 'NONE',  ( 10.13694260842256689, -3580.732079930104646, 2249.536708023868414 ) ) ;
#14017=CIRCLE ( 'NONE', #15134, 3.606800000000000228 ) ;
#14020=DIRECTION ( 'NONE',  ( 0.000000000000000000, 0.000000000000000000, 1.000000000000000000 ) ) ;
#14024=CARTESIAN_POINT ( 'NONE',  ( 12.83072102879435405, -3662.349731445673115, 2249.183616308214823 ) ) ;
#14028=CIRCLE ( 'NONE', #179, 3.606799999999001027 ) ;
#14029=CARTESIAN_POINT ( 'NONE',  ( 76.20000000000000284, -3568.700000000000273, 2259.837999999999738 ) ) ;
#14032=CARTESIAN_POINT ( 'NONE',  ( 98.75520000000000209, -3619.500000000000000, 2259.837999999999738 ) ) ;
#14034=CARTESIAN_POINT ( 'NONE',  ( 15.14452126063228832, -3658.050008149689802, 2249.322202696583190 ) ) ;
#14035=CARTESIAN_POINT ( 'NONE',  ( 15.47299515201000020, -3578.859991782000179, 2250.236800948000109 ) ) ;
#14039=CARTESIAN_POINT ( 'NONE',  ( 9.822867848221497056, -3543.373434452745187, 2254.929970520540337 ) ) ;
#14042=DIRECTION ( 'NONE',  ( -1.000000000000000000, 0.000000000000000000, 0.000000000000000000 ) ) ;
#14044=TOROIDAL_SURFACE ( 'NONE', #5452, 6.477000000000000313, 0.7620000000000000107 ) ;
#14046=EDGE_CURVE ( 'NONE', #7103, #17227, #8298, .T. ) ;
#14047=FACE_OUTER_BOUND ( 'NONE', #6274, .T. ) ;
#14058=CARTESIAN_POINT ( 'NONE',  ( 133.9850000019999925, -3579.494756921999851, 2244.617465693000213 ) ) ;
#14061=EDGE_LOOP ( 'NONE', ( #17119, #13854, #5622, #22044 ) ) ;
#14065=AXIS2_PLACEMENT_3D ( 'NONE', #12521, #5383, #21776 ) ;
#14067=ORIENTED_EDGE ( 'NONE', *, *, #16236, .T. ) ;
#14068=CARTESIAN_POINT ( 'NONE',  ( 131.9781484670521081, -3695.197007937890248, 2260.344194844531557 ) ) ;
#14072=CARTESIAN_POINT ( 'NONE',  ( 15.35230487608980710, -3580.523739450907669, 2249.699608343330965 ) ) ;
#14075=AXIS2_PLACEMENT_3D ( 'NONE', #19390, #21032, #10360 ) ;
#14076=DIRECTION ( 'NONE',  ( 0.000000000000000000, 0.000000000000000000, 1.000000000000000000 ) ) ;
#14078=AXIS2_PLACEMENT_3D ( 'NONE', #5236, #21179, #23140 ) ;
#14079=CARTESIAN_POINT ( 'NONE',  ( 15.57713215129027340, -3695.626565546841903, 2254.929970521695395 ) ) ;
#14080=VECTOR ( 'NONE', #3601, 1000.000000000000000 ) ;
#14082=CARTESIAN_POINT ( 'NONE',  ( 28.24479999999899604, -3670.300000000000182, 2239.771999999999935 ) ) ;
#14085=AXIS2_PLACEMENT_3D ( 'NONE', #15352, #16642, #16869 ) ;
#14086=EDGE_LOOP ( 'NONE', ( #11460, #4780, #9332, #3445, #11386, #11483 ) ) ;
#14088=ORIENTED_EDGE ( 'NONE', *, *, #4996, .T. ) ;
#14089=LINE ( 'NONE', #17347, #16161 ) ;
#14090=FACE_OUTER_BOUND ( 'NONE', #11966, .T. ) ;
#14091=EDGE_LOOP ( 'NONE', ( #9158, #12014 ) ) ;
#14094=CARTESIAN_POINT ( 'NONE',  ( 0.000000000000000000, -3578.860000000000127, 2247.392000000000280 ) ) ;
#14100=CARTESIAN_POINT ( 'NONE',  ( 10.01415227263506580, -3695.321318630586120, 2255.408757311871341 ) ) ;
#14101=CARTESIAN_POINT ( 'NONE',  ( 25.39999999999999858, -3568.700000000000273, 2261.869999999999891 ) ) ;
#14102=ADVANCED_FACE ( 'NONE', ( #2529 ), #9672, .F. ) ;
#14103=AXIS2_PLACEMENT_3D ( 'NONE', #22527, #6497, #22296 ) ;
#14105=CARTESIAN_POINT ( 'NONE',  ( 137.3103389895218243, -3657.961604733812692, 2249.221652488155087 ) ) ;
#14109=ADVANCED_FACE ( 'NONE', ( #18799 ), #4960, .T. ) ;
#14111=ORIENTED_EDGE ( 'NONE', *, *, #3935, .T. ) ;
#14113=TOROIDAL_SURFACE ( 'NONE', #21596, 4.114799999999999791, 1.270000000000000018 ) ;
#14115=VERTEX_POINT ( 'NONE', #8032 ) ;
#14116=VERTEX_POINT ( 'NONE', #4402 ) ;
#14117=CARTESIAN_POINT ( 'NONE',  ( 4.572920519510000226, -3543.299999999999727, 2259.329999999999927 ) ) ;
#14118=EDGE_CURVE ( 'NONE', #5536, #13127, #14707, .T. ) ;
#14122=CIRCLE ( 'NONE', #7020, 0.7619999999999987894 ) ;
#14126=DIRECTION ( 'NONE',  ( 0.000000000000000000, -1.000000000000000000, 0.000000000000000000 ) ) ;
#14135=CARTESIAN_POINT ( 'NONE',  ( 10.77163876081882243, -3581.586621143886987, 2248.203750047890935 ) ) ;
#14136=AXIS2_PLACEMENT_3D ( 'NONE', #20400, #6348, #4235 ) ;
#14137=DIRECTION ( 'NONE',  ( 1.000000000000000000, 0.000000000000000000, 0.000000000000000000 ) ) ;
#14141=ADVANCED_FACE ( 'NONE', ( #11763 ), #17683, .T. ) ;
#14142=EDGE_CURVE ( 'NONE', #287, #15612, #21445, .T. ) ;
#14144=DIRECTION ( 'NONE',  ( -1.224646799147353207E-16, 1.000000000000000000, 0.000000000000000000 ) ) ;
#14147=CARTESIAN_POINT ( 'NONE',  ( 12.17149329490156084, -3662.301214434115991, 2249.242076774587986 ) ) ;
#14148=ORIENTED_EDGE ( 'NONE', *, *, #20279, .F. ) ;
#14151=ORIENTED_EDGE ( 'NONE', *, *, #14461, .T. ) ;
#14153=CARTESIAN_POINT ( 'NONE',  ( 142.5448000000000093, -3579.494999999999891, 2256.063560000000052 ) ) ;
#14155=VECTOR ( 'NONE', #436, 1000.000000000000000 ) ;
#14157=CARTESIAN_POINT ( 'NONE',  ( 14.97105788294492612, -3657.791708964490226, 2248.997938942161454 ) ) ;
#14158=CARTESIAN_POINT ( 'NONE',  ( 137.0704399687386115, -3695.151712727613813, 2255.549808266575383 ) ) ;
#14159=CARTESIAN_POINT ( 'NONE',  ( 9.993247422846968320, -3578.570632894392929, 2250.236801304443816 ) ) ;
#14160=ADVANCED_FACE ( 'NONE', ( #20344 ), #9103, .T. ) ;
#14161=ORIENTED_EDGE ( 'NONE', *, *, #21399, .F. ) ;
#14162=DIRECTION ( 'NONE',  ( 1.000000000000000000, 0.000000000000000000, 0.000000000000000000 ) ) ;
#14168=ORIENTED_EDGE ( 'NONE', *, *, #7827, .T. ) ;
#14169=CARTESIAN_POINT ( 'NONE',  ( 20.62424768829000143, -3544.570000000000164, 2260.600000000000364 ) ) ;
#14171=DIRECTION ( 'NONE',  ( 0.000000000000000000, 0.000000000000000000, -1.000000000000000000 ) ) ;
#14172=AXIS2_PLACEMENT_3D ( 'NONE', #20773, #2613, #9757 ) ;
#14173=ADVANCED_FACE ( 'NONE', ( #6746 ), #18442, .T. ) ;
#14174=EDGE_CURVE ( 'NONE', #22625, #3671, #15647, .T. ) ;
#14175=CARTESIAN_POINT ( 'NONE',  ( 38.10000000000000142, -3594.099999999999909, 2239.771999999999935 ) ) ;
#14179=ORIENTED_EDGE ( 'NONE', *, *, #19921, .F. ) ;
#14181=DIRECTION ( 'NONE',  ( 0.000000000000000000, 1.000000000000000000, 0.000000000000000000 ) ) ;
#14183=CARTESIAN_POINT ( 'NONE',  ( 142.7470794804999912, -3695.699999999999818, 2254.503999999999905 ) ) ;
#14184=CARTESIAN_POINT ( 'NONE',  ( 127.0000000000000000, -3568.700000000000273, 2239.009999999999764 ) ) ;
#14185=VERTEX_POINT ( 'NONE', #3096 ) ;
#14187=EDGE_LOOP ( 'NONE', ( #5995, #68, #6670, #18806 ) ) ;
#14190=EDGE_LOOP ( 'NONE', ( #9654, #8196 ) ) ;
#14191=DIRECTION ( 'NONE',  ( 0.000000000000000000, -1.000000000000000000, 0.000000000000000000 ) ) ;
#14193=CARTESIAN_POINT ( 'NONE',  ( 35.56000000000000227, -3568.700000000000273, 2247.392000000000280 ) ) ;
#14194=CARTESIAN_POINT ( 'NONE',  ( 15.15106812040523998, -3580.939163279126660, 2249.333860731847835 ) ) ;
#14196=DIRECTION ( 'NONE',  ( 1.224646799147353207E-16, 1.000000000000000000, -0.000000000000000000 ) ) ;
#14198=VERTEX_POINT ( 'NONE', #23125 ) ;
#14199=CARTESIAN_POINT ( 'NONE',  ( 15.48312395866995494, -3695.517456594313444, 2255.165366398894548 ) ) ;
#14202=CARTESIAN_POINT ( 'NONE',  ( 4.806192532568648978, -3695.561367818985218, 2259.914321287728399 ) ) ;
#14203=LINE ( 'NONE', #18055, #8752 ) ;
#14204=CARTESIAN_POINT ( 'NONE',  ( 20.25432815364000305, -3544.321224993999749, 2260.506484774000000 ) ) ;
#14209=DIRECTION ( 'NONE',  ( -1.000000000000000000, 0.000000000000000000, 0.000000000000000000 ) ) ;
#14210=DIRECTION ( 'NONE',  ( -0.6887494619146554697, 0.000000000000000000, -0.7249994335944496271 ) ) ;
#14211=DIRECTION ( 'NONE',  ( 0.000000000000000000, 0.000000000000000000, -1.000000000000000000 ) ) ;
#14213=CIRCLE ( 'NONE', #3341, 2.844799999999994444 ) ;
#14215=CARTESIAN_POINT ( 'NONE',  ( 9.787879217019574085, -3695.655085023491210, 2254.841286578994641 ) ) ;
#14217=DIRECTION ( 'NONE',  ( 0.000000000000000000, 0.000000000000000000, -1.000000000000000000 ) ) ;
#14219=CARTESIAN_POINT ( 'NONE',  ( 137.0543742791004149, -3658.459229904648510, 2249.687221467814197 ) ) ;
#14220=ORIENTED_EDGE ( 'NONE', *, *, #21889, .T. ) ;
#14223=ORIENTED_EDGE ( 'NONE', *, *, #4521, .T. ) ;
#14226=CIRCLE ( 'NONE', #21337, 3.606799999999993567 ) ;
#14227=CARTESIAN_POINT ( 'NONE',  ( 9.859719926546999247, -3579.298590683999919, 2250.205126089999794 ) ) ;
#14229=ORIENTED_EDGE ( 'NONE', *, *, #1965, .F. ) ;
#14235=CARTESIAN_POINT ( 'NONE',  ( 0.000000000000000000, -3695.699999999999818, 2260.600000000000364 ) ) ;
#14240=FACE_BOUND ( 'NONE', #4878, .T. ) ;
#14241=CARTESIAN_POINT ( 'NONE',  ( 25.39999999999999858, -3568.700000000000273, 2259.837999999999738 ) ) ;
#14245=EDGE_CURVE ( 'NONE', #20927, #15488, #18801, .T. ) ;
#14246=CARTESIAN_POINT ( 'NONE',  ( 132.0221669333815555, -3543.967586182882769, 2260.455859883436005 ) ) ;
#14248=DIRECTION ( 'NONE',  ( 0.000000000000000000, 1.000000000000000000, 0.000000000000000000 ) ) ;
#14250=CYLINDRICAL_SURFACE ( 'NONE', #8052, 1.269999999999993356 ) ;
#14253=LINE ( 'NONE', #5115, #11091 ) ;
#14256=CARTESIAN_POINT ( 'NONE',  ( 117.1447999999989946, -3644.899999999999636, 2261.869999999999891 ) ) ;
#14263=ADVANCED_FACE ( 'NONE', ( #8849 ), #7248, .T. ) ;
#14267=CARTESIAN_POINT ( 'NONE',  ( 14.91356650787898275, -3657.717498031156993, 2248.884953215802398 ) ) ;
#14268=CARTESIAN_POINT ( 'NONE',  ( 50.79999999999999716, -3619.500000000000000, 2261.869999999999891 ) ) ;
#14273=EDGE_LOOP ( 'NONE', ( #15717, #20803 ) ) ;
#14274=DIRECTION ( 'NONE',  ( 0.000000000000000000, 0.000000000000000000, 1.000000000000000000 ) ) ;
#14278=DIRECTION ( 'NONE',  ( 0.000000000000000000, 0.000000000000000000, 1.000000000000000000 ) ) ;
#14281=FACE_OUTER_BOUND ( 'NONE', #18704, .T. ) ;
#14284=ORIENTED_EDGE ( 'NONE', *, *, #17226, .T. ) ;
#14286=FACE_OUTER_BOUND ( 'NONE', #4984, .T. ) ;
#14287=EDGE_LOOP ( 'NONE', ( #2548, #14630, #1565, #19508 ) ) ;
#14288=CARTESIAN_POINT ( 'NONE',  ( 35.56000000000031491, -3568.700000000000273, 2250.236800000000130 ) ) ;
#14290=CIRCLE ( 'NONE', #7181, 2.844800000000091700 ) ;
#14292=CARTESIAN_POINT ( 'NONE',  ( 142.4828652621451681, -3695.514947976519579, 2255.165528820269174 ) ) ;
#14295=VERTEX_POINT ( 'NONE', #22662 ) ;
#14298=CARTESIAN_POINT ( 'NONE',  ( 136.9934899154386301, -3580.373043272544237, 2249.801989270562899 ) ) ;
#14300=DIRECTION ( 'NONE',  ( 0.000000000000000000, 0.000000000000000000, 1.000000000000000000 ) ) ;
#14303=CARTESIAN_POINT ( 'NONE',  ( 116.8400000000003160, -3568.700000000000273, 2250.236800000000130 ) ) ;
#14306=AXIS2_PLACEMENT_3D ( 'NONE', #8590, #964, #6726 ) ;
#14307=FACE_OUTER_BOUND ( 'NONE', #10481, .T. ) ;
#14309=CIRCLE ( 'NONE', #12794, 1.269999999999882334 ) ;
#14310=CARTESIAN_POINT ( 'NONE',  ( 76.20000000000000284, -3670.300000000000182, 2239.009999999999764 ) ) ;
#14312=CARTESIAN_POINT ( 'NONE',  ( 134.5774142888278391, -3576.960814571373248, 2245.272442446700552 ) ) ;
#14314=EDGE_CURVE ( 'NONE', #10278, #1882, #16583, .T. ) ;
#14315=FACE_OUTER_BOUND ( 'NONE', #15188, .T. ) ;
#14316=EDGE_LOOP ( 'NONE', ( #14617, #16051, #19567, #13327 ) ) ;
#14321=ORIENTED_EDGE ( 'NONE', *, *, #7805, .F. ) ;
#14322=LINE ( 'NONE', #14440, #7946 ) ;
#14325=CIRCLE ( 'NONE', #22898, 5.714999999999995417 ) ;
#14326=ORIENTED_EDGE ( 'NONE', *, *, #20668, .T. ) ;
#14332=DIRECTION ( 'NONE',  ( -0.000000000000000000, -1.000000000000000000, -0.000000000000000000 ) ) ;
#14335=DIRECTION ( 'NONE',  ( 0.000000000000000000, 0.000000000000000000, 1.000000000000000000 ) ) ;
#14336=DIRECTION ( 'NONE',  ( 0.000000000000000000, 0.000000000000000000, 1.000000000000000000 ) ) ;
#14339=AXIS2_PLACEMENT_3D ( 'NONE', #1554, #15859, #4606 ) ;
#14340=CARTESIAN_POINT ( 'NONE',  ( 137.0509968171786568, -3658.467794019345547, 2249.693473747279768 ) ) ;
#14341=VERTEX_POINT ( 'NONE', #2277 ) ;
#14343=CARTESIAN_POINT ( 'NONE',  ( 98.75520000000000209, -3670.300000000000182, 2239.771999999999935 ) ) ;
#14344=AXIS2_PLACEMENT_3D ( 'NONE', #13185, #2530, #16705 ) ;
#14346=ORIENTED_EDGE ( 'NONE', *, *, #16727, .T. ) ;
#14348=CYLINDRICAL_SURFACE ( 'NONE', #609, 2.844800000000091700 ) ;
#14349=ORIENTED_EDGE ( 'NONE', *, *, #7240, .F. ) ;
#14351=CARTESIAN_POINT ( 'NONE',  ( 123.3932000000010021, -3568.700000000000273, 2239.771999999999935 ) ) ;
#14354=CARTESIAN_POINT ( 'NONE',  ( 147.3199999999999932, -3694.430000000000291, 2260.600000000000364 ) ) ;
#14355=ORIENTED_EDGE ( 'NONE', *, *, #14891, .F. ) ;
#14358=CARTESIAN_POINT ( 'NONE',  ( 6.985000002048999512, -3579.494756921999851, 2244.617465693000213 ) ) ;
#14363=CARTESIAN_POINT ( 'NONE',  ( 131.7443772039423493, -3543.374810890516983, 2259.759470120345213 ) ) ;
#14365=LINE ( 'NONE', #19865, #6823 ) ;
#14366=EDGE_CURVE ( 'NONE', #5595, #3108, #14701, .T. ) ;
#14367=DIRECTION ( 'NONE',  ( 0.000000000000000000, 0.000000000000000000, -1.000000000000000000 ) ) ;
#14370=DIRECTION ( 'NONE',  ( 0.000000000000000000, -1.000000000000000000, 0.000000000000000000 ) ) ;
#14372=CARTESIAN_POINT ( 'NONE',  ( 9.956800000000452400, -3580.373257047480820, 2255.967039999999997 ) ) ;
#14374=DIRECTION ( 'NONE',  ( 0.000000000000000000, 0.000000000000000000, 1.000000000000000000 ) ) ;
#14375=CARTESIAN_POINT ( 'NONE',  ( 12.69999999999999929, -3579.494999999999891, 2272.030000000000200 ) ) ;
#14376=VERTEX_POINT ( 'NONE', #14476 ) ;
#14377=DIRECTION ( 'NONE',  ( 0.000000000000000000, 0.000000000000000000, 1.000000000000000000 ) ) ;
#14378=DIRECTION ( 'NONE',  ( -1.000000000000000000, 0.000000000000000000, -8.741913579724999851E-14 ) ) ;
#14380=DIRECTION ( 'NONE',  ( 0.000000000000000000, 0.000000000000000000, 1.000000000000000000 ) ) ;
#14381=CARTESIAN_POINT ( 'NONE',  ( 142.3546999974072378, -3543.765301130966236, 2255.486749947766384 ) ) ;
#14382=CARTESIAN_POINT ( 'NONE',  ( 136.8622528204724063, -3695.586719555755280, 2255.028339697612864 ) ) ;
#14384=CIRCLE ( 'NONE', #22589, 2.844800000000001550 ) ;
#14385=CARTESIAN_POINT ( 'NONE',  ( 7.181610858756661386, -3578.008765548840984, 2244.677489325244096 ) ) ;
#14386=ORIENTED_EDGE ( 'NONE', *, *, #14544, .T. ) ;
#14391=DIRECTION ( 'NONE',  ( -1.000000000000000000, 0.000000000000000000, 0.000000000000000000 ) ) ;
#14394=DIRECTION ( 'NONE',  ( 1.122008997397786234E-13, 0.000000000000000000, 1.000000000000000000 ) ) ;
#14396=CYLINDRICAL_SURFACE ( 'NONE', #21250, 2.844799999999994444 ) ;
#14402=DIRECTION ( 'NONE',  ( -0.6887494619146554697, 0.000000000000000000, -0.7249994335944496271 ) ) ;
#14403=AXIS2_PLACEMENT_3D ( 'NONE', #5097, #12240, #1685 ) ;
#14407=CARTESIAN_POINT ( 'NONE',  ( 142.5173730182035285, -3695.562642950982081, 2255.079208150718387 ) ) ;
#14408=DIRECTION ( 'NONE',  ( 0.000000000000000000, 0.000000000000000000, -1.000000000000000000 ) ) ;
#14409=EDGE_CURVE ( 'NONE', #4689, #10096, #4035, .T. ) ;
#14412=CARTESIAN_POINT ( 'NONE',  ( 137.9083009636803467, -3581.704713601686308, 2247.346194313388423 ) ) ;
#14418=AXIS2_PLACEMENT_3D ( 'NONE', #19010, #18889, #2833 ) ;
#14419=DIRECTION ( 'NONE',  ( 0.8928571428573600643, -0.4503400076038009403, 0.000000000000000000 ) ) ;
#14422=EDGE_CURVE ( 'NONE', #12415, #10003, #13314, .T. ) ;
#14424=CARTESIAN_POINT ( 'NONE',  ( 142.1563837964497168, -3578.059926228095264, 2250.122030119480769 ) ) ;
#14426=CARTESIAN_POINT ( 'NONE',  ( 134.7476930285313870, -3576.642325314609479, 2245.609748385880266 ) ) ;
#14430=EDGE_LOOP ( 'NONE', ( #14866, #9058, #1460, #7162, #18409, #21136, #9469, #18953, #809, #12037 ) ) ;
#14431=B_SPLINE_CURVE_WITH_KNOTS ( 'NONE', 3,
 ( #18512, #704, #13232, #11584, #11476, #4220, #804, #11143, #16523, #5990, #7617, #475, #9388, #4337, #18732, #22363, #11253, #9829, #16759, #18397, #6219, #14776, #9612, #21917 ),
 .UNSPECIFIED., .F., .F.,
 ( 4, 2, 2, 1, 1, 1, 2, 2, 2, 2, 1, 2, 2, 4 ),
 ( 0.000000000000000000, 0.1249999999974724663, 0.1874999999964171993, 0.2187499999956769026, 0.2343749999957942254, 0.2421874999958534558, 0.2460937499958825159, 0.2499999999959115482, 0.3749999999939945816, 0.4374999999928649852, 0.4687499999920584082, 0.4843749999916692750, 0.4999999999912801973, 1.000000000000000000 ),
 .UNSPECIFIED. ) ;
#14432=AXIS2_PLACEMENT_3D ( 'NONE', #20634, #9638, #16665 ) ;
#14433=CARTESIAN_POINT ( 'NONE',  ( 4.762728537569663523, -3695.607672419785104, 2259.805487872981303 ) ) ;
#14434=B_SPLINE_CURVE_WITH_KNOTS ( 'NONE', 3,
 ( #9933, #8306, #8189, #17431 ),
 .UNSPECIFIED., .F., .F.,
 ( 4, 4 ),
 ( 0.000000000000000000, 1.000000000000000000 ),
 .UNSPECIFIED. ) ;
#14435=CARTESIAN_POINT ( 'NONE',  ( 73.35520000000001062, -3568.700000000000273, 2261.869999999999891 ) ) ;
#14436=AXIS2_PLACEMENT_3D ( 'NONE', #18729, #19088, #17320 ) ;
#14440=CARTESIAN_POINT ( 'NONE',  ( 137.1599999999999966, -3694.430000000000291, 2255.774000000000342 ) ) ;
#14442=AXIS2_PLACEMENT_3D ( 'NONE', #17578, #3167, #20875 ) ;
#14447=DIRECTION ( 'NONE',  ( -1.000000000000000000, 0.000000000000000000, 0.000000000000000000 ) ) ;
#14451=CARTESIAN_POINT ( 'NONE',  ( 10.16000000000000014, -3694.430000000000291, 2255.774000000000342 ) ) ;
#14453=CARTESIAN_POINT ( 'NONE',  ( 18.22054351403157924, -3580.973142365039621, 2245.487016238938850 ) ) ;
#14454=CIRCLE ( 'NONE', #4335, 2.844799999999994444 ) ;
#14456=CARTESIAN_POINT ( 'NONE',  ( 137.5955831568913936, -3657.590698734706621, 2248.654663951603197 ) ) ;
#14457=AXIS2_PLACEMENT_3D ( 'NONE', #13647, #8847, #3094 ) ;
#14458=ORIENTED_EDGE ( 'NONE', *, *, #10084, .T. ) ;
#14459=VECTOR ( 'NONE', #3110, 1000.000000000000000 ) ;
#14460=CARTESIAN_POINT ( 'NONE',  ( 139.9704182635913128, -3662.340201044270998, 2249.195591307148334 ) ) ;
#14461=EDGE_CURVE ( 'NONE', #12349, #21351, #500, .T. ) ;
#14463=EDGE_LOOP ( 'NONE', ( #17237, #3246 ) ) ;
#14464=CARTESIAN_POINT ( 'NONE',  ( 9.855190710340998805, -3579.495000415000050, 2250.165025612000136 ) ) ;
#14466=ORIENTED_EDGE ( 'NONE', *, *, #19982, .T. ) ;
#14468=CIRCLE ( 'NONE', #11077, 2.844799999999994444 ) ;
#14470=CARTESIAN_POINT ( 'NONE',  ( 10.16000000000000014, -3694.430000000000291, 2255.774000000000342 ) ) ;
#14471=CARTESIAN_POINT ( 'NONE',  ( 127.0000000000000000, -3568.700000000000273, 2259.837999999999738 ) ) ;
#14472=ORIENTED_EDGE ( 'NONE', *, *, #2941, .T. ) ;
#14475=CARTESIAN_POINT ( 'NONE',  ( 10.16000000000000014, -3578.213872745999652, 2255.774000000000342 ) ) ;
#14476=CARTESIAN_POINT ( 'NONE',  ( 132.0583097651000060, -3544.202533098000458, 2260.545675974999995 ) ) ;
#14483=AXIS2_PLACEMENT_3D ( 'NONE', #10148, #673, #6071 ) ;
#14484=CARTESIAN_POINT ( 'NONE',  ( 57.14999999999999858, -3694.430000000000291, 2250.236800000000130 ) ) ;
#14488=ORIENTED_EDGE ( 'NONE', *, *, #10015, .T. ) ;
#14489=DIRECTION ( 'NONE',  ( 0.000000000000000000, 0.000000000000000000, -1.000000000000000000 ) ) ;
#14490=AXIS2_PLACEMENT_3D ( 'NONE', #10947, #9197, #4482 ) ;
#14496=CARTESIAN_POINT ( 'NONE',  ( 18.02447335878156665, -3657.428416424212173, 2246.524741530415668 ) ) ;
#14500=DIRECTION ( 'NONE',  ( 0.000000000000000000, 0.000000000000000000, -1.000000000000000000 ) ) ;
#14502=CARTESIAN_POINT ( 'NONE',  ( 124.1552000000010025, -3568.700000000000273, 2239.771999999999935 ) ) ;
#14503=CARTESIAN_POINT ( 'NONE',  ( 137.0197862866483831, -3695.306816721486484, 2255.422793245717912 ) ) ;
#14504=ORIENTED_EDGE ( 'NONE', *, *, #19140, .T. ) ;
#14505=CARTESIAN_POINT ( 'NONE',  ( 7.635186067085399486, -3576.847633590237820, 2245.381158637630051 ) ) ;
#14510=CARTESIAN_POINT ( 'NONE',  ( 25.39999999999999858, -3619.500000000000000, 2239.771999999999935 ) ) ;
#14512=CIRCLE ( 'NONE', #1018, 3.606799999998994366 ) ;
#14514=CARTESIAN_POINT ( 'NONE',  ( 131.5729205195000020, -3543.299999999999727, 2259.329999999999927 ) ) ;
#14515=DIRECTION ( 'NONE',  ( -1.000000000000000000, 0.000000000000000000, 0.000000000000000000 ) ) ;
#14516=AXIS2_PLACEMENT_3D ( 'NONE', #18742, #2808, #1049 ) ;
#14517=DIRECTION ( 'NONE',  ( 1.000000000000000000, 0.000000000000000000, 0.000000000000000000 ) ) ;
#14525=DIRECTION ( 'NONE',  ( 0.000000000000000000, 0.000000000000000000, 1.000000000000000000 ) ) ;
#14527=ADVANCED_FACE ( 'NONE', ( #13270 ), #22173, .T. ) ;
#14528=ORIENTED_EDGE ( 'NONE', *, *, #16323, .F. ) ;
#14529=CARTESIAN_POINT ( 'NONE',  ( 142.5056715281748154, -3695.547111919549934, 2255.108476226979292 ) ) ;
#14534=CARTESIAN_POINT ( 'NONE',  ( 137.5722701175336908, -3581.383294861765989, 2248.705728950628327 ) ) ;
#14535=ORIENTED_EDGE ( 'NONE', *, *, #11069, .F. ) ;
#14536=CARTESIAN_POINT ( 'NONE',  ( 47.19319999999999737, -3619.500000000000000, 2239.771999999999935 ) ) ;
#14539=DIRECTION ( 'NONE',  ( 1.000000000000000000, 0.000000000000000000, 0.000000000000000000 ) ) ;
#14543=DIRECTION ( 'NONE',  ( 0.000000000000000000, 0.000000000000000000, -1.000000000000000000 ) ) ;
#14544=EDGE_CURVE ( 'NONE', #9562, #22886, #138, .T. ) ;
#14545=CARTESIAN_POINT ( 'NONE',  ( 141.0188720128104762, -3576.974003297035779, 2249.521926086513304 ) ) ;
#14546=EDGE_LOOP ( 'NONE', ( #2801, #10924, #21020, #11145 ) ) ;
#14547=CARTESIAN_POINT ( 'NONE',  ( 134.4979089453188692, -3577.128741457883280, 2245.134603798921034 ) ) ;
#14549=DIRECTION ( 'NONE',  ( 1.000000000000000000, 0.000000000000000000, 0.000000000000000000 ) ) ;
#14550=EDGE_LOOP ( 'NONE', ( #17938, #4199, #1153, #12294 ) ) ;
#14555=CARTESIAN_POINT ( 'NONE',  ( 95.25000000000000000, -3695.699999999999818, 2251.506800000000112 ) ) ;
#14556=AXIS2_PLACEMENT_3D ( 'NONE', #7260, #16046, #10649 ) ;
#14558=VERTEX_POINT ( 'NONE', #630 ) ;
#14566=CARTESIAN_POINT ( 'NONE',  ( 18.41519309055000164, -3659.504912144000173, 2244.618989493999834 ) ) ;
#14567=EDGE_LOOP ( 'NONE', ( #16405, #8116, #14472, #18674 ) ) ;
#14569=CYLINDRICAL_SURFACE ( 'NONE', #2354, 2.844800000000091700 ) ;
#14572=ORIENTED_EDGE ( 'NONE', *, *, #6816, .F. ) ;
#14574=CARTESIAN_POINT ( 'NONE',  ( 140.5954651218877132, -3662.206385911813868, 2249.347528825103836 ) ) ;
#14575=VERTEX_POINT ( 'NONE', #14929 ) ;
#14581=FACE_OUTER_BOUND ( 'NONE', #21927, .T. ) ;
#14583=ORIENTED_EDGE ( 'NONE', *, *, #15419, .T. ) ;
#14585=CARTESIAN_POINT ( 'NONE',  ( 7.360523049854252875, -3581.533682375841181, 2246.411846944129593 ) ) ;
#14586=TOROIDAL_SURFACE ( 'NONE', #12337, 3.606799999999999784, 0.7620000000000000107 ) ;
#14587=CARTESIAN_POINT ( 'NONE',  ( 19.17699999999999960, -3659.504999999999654, 2239.009999999999764 ) ) ;
#14589=EDGE_CURVE ( 'NONE', #15032, #10446, #7893, .T. ) ;
#14591=EDGE_CURVE ( 'NONE', #16048, #13554, #15466, .T. ) ;
#14593=VERTEX_POINT ( 'NONE', #15154 ) ;
#14594=DIRECTION ( 'NONE',  ( 0.000000000000000000, 0.000000000000000000, -1.000000000000000000 ) ) ;
#14595=CARTESIAN_POINT ( 'NONE',  ( 19.17699999999999960, -3659.504999999999654, 2239.771999999999935 ) ) ;
#14604=DIRECTION ( 'NONE',  ( 1.000000000000000000, 0.000000000000000000, 0.000000000000000000 ) ) ;
#14607=EDGE_CURVE ( 'NONE', #3620, #4452, #21076, .T. ) ;
#14608=LINE ( 'NONE', #14840, #17050 ) ;
#14610=CARTESIAN_POINT ( 'NONE',  ( 7.387125747152000876, -3657.399152860999493, 2246.630000000000109 ) ) ;
#14611=FACE_OUTER_BOUND ( 'NONE', #1728, .T. ) ;
#14614=CARTESIAN_POINT ( 'NONE',  ( 142.5447279057234198, -3543.405519448513587, 2255.010851276078483 ) ) ;
#14615=DIRECTION ( 'NONE',  ( 0.000000000000000000, 1.000000000000000000, 0.000000000000000000 ) ) ;
#14616=CARTESIAN_POINT ( 'NONE',  ( 20.62424768829000143, -3544.570000000000164, 2260.600000000000364 ) ) ;
#14617=ORIENTED_EDGE ( 'NONE', *, *, #8253, .F. ) ;
#14619=CIRCLE ( 'NONE', #19473, 0.7619999999999987894 ) ;
#14626=CARTESIAN_POINT ( 'NONE',  ( 127.0000000000000000, -3670.300000000000182, 2239.771999999999935 ) ) ;
#14627=CARTESIAN_POINT ( 'NONE',  ( 57.14999999999999858, -3670.300000000000182, 2244.547199999999975 ) ) ;
#14628=AXIS2_PLACEMENT_3D ( 'NONE', #21124, #6719, #22751 ) ;
#14630=ORIENTED_EDGE ( 'NONE', *, *, #13211, .F. ) ;
#14632=ORIENTED_EDGE ( 'NONE', *, *, #16443, .F. ) ;
#14634=FACE_OUTER_BOUND ( 'NONE', #14546, .T. ) ;
#14635=ORIENTED_EDGE ( 'NONE', *, *, #11251, .T. ) ;
#14639=CIRCLE ( 'NONE', #10514, 1.269999999999882334 ) ;
#14640=VERTEX_POINT ( 'NONE', #15623 ) ;
#14641=CARTESIAN_POINT ( 'NONE',  ( 142.3546858854725201, -3695.234698869114709, 2255.486744312730025 ) ) ;
#14643=ORIENTED_EDGE ( 'NONE', *, *, #7154, .T. ) ;
#14645=CARTESIAN_POINT ( 'NONE',  ( 137.3238766226560301, -3581.059663267119049, 2249.196894471709129 ) ) ;
#14647=ORIENTED_EDGE ( 'NONE', *, *, #19519, .T. ) ;
#14648=FACE_OUTER_BOUND ( 'NONE', #22746, .T. ) ;
#14652=CARTESIAN_POINT ( 'NONE',  ( 136.6529205195000145, -3543.299999999999727, 2254.503999999999905 ) ) ;
#14653=CARTESIAN_POINT ( 'NONE',  ( 20.32000000000000028, -3695.699999999999818, 2260.600000000000364 ) ) ;
#14655=EDGE_CURVE ( 'NONE', #22478, #6888, #22752, .T. ) ;
#14656=CARTESIAN_POINT ( 'NONE',  ( 138.5749913602858499, -3576.881732504405591, 2249.436484161916269 ) ) ;
#14657=ORIENTED_EDGE ( 'NONE', *, *, #6520, .F. ) ;
#14659=ADVANCED_FACE ( 'NONE', ( #8355 ), #850, .T. ) ;
#14660=AXIS2_PLACEMENT_3D ( 'NONE', #7776, #11506, #2386 ) ;
#14661=DIRECTION ( 'NONE',  ( 1.224646799147353207E-16, 1.000000000000000000, -0.000000000000000000 ) ) ;
#14662=ORIENTED_EDGE ( 'NONE', *, *, #20404, .F. ) ;
#14663=CARTESIAN_POINT ( 'NONE',  ( 50.79999999999999716, -3670.300000000000182, 2239.009999999999764 ) ) ;
#14664=CARTESIAN_POINT ( 'NONE',  ( 136.9568000000001291, -3658.626742952567838, 2255.967039999999997 ) ) ;
#14667=DIRECTION ( 'NONE',  ( 1.000000000000000000, 0.000000000000000000, 0.000000000000000000 ) ) ;
#14668=ORIENTED_EDGE ( 'NONE', *, *, #22126, .F. ) ;
#14669=DIRECTION ( 'NONE',  ( -1.000000000000000000, 0.000000000000000000, 0.000000000000000000 ) ) ;
#14671=CARTESIAN_POINT ( 'NONE',  ( 141.5168031146254464, -3581.684176781325277, 2247.047623956332700 ) ) ;
#14672=ORIENTED_EDGE ( 'NONE', *, *, #8662, .T. ) ;
#14673=CIRCLE ( 'NONE', #14306, 1.269999999999882334 ) ;
#14677=AXIS2_PLACEMENT_3D ( 'NONE', #478, #7403, #14779 ) ;
#14678=DIRECTION ( 'NONE',  ( -1.000000000000000000, 0.000000000000000000, 0.000000000000000000 ) ) ;
#14679=DIRECTION ( 'NONE',  ( 0.000000000000000000, -1.000000000000000000, 0.000000000000000000 ) ) ;
#14682=DIRECTION ( 'NONE',  ( -0.9296367896483511695, 0.3684771897042033451, 0.000000000000000000 ) ) ;
#14683=ADVANCED_FACE ( 'NONE', ( #13750 ), #21008, .F. ) ;
#14686=CIRCLE ( 'NONE', #8321, 2.844800000000091700 ) ;
#14687=CARTESIAN_POINT ( 'NONE',  ( 138.3419138266048378, -3662.005144841253241, 2249.540250141421438 ) ) ;
#14688=EDGE_CURVE ( 'NONE', #17829, #3614, #15733, .T. ) ;
#14689=ORIENTED_EDGE ( 'NONE', *, *, #1529, .F. ) ;
#14691=ORIENTED_EDGE ( 'NONE', *, *, #634, .F. ) ;
#14693=CIRCLE ( 'NONE', #17297, 2.844799999998995244 ) ;
#14697=FACE_OUTER_BOUND ( 'NONE', #22845, .T. ) ;
#14698=ORIENTED_EDGE ( 'NONE', *, *, #2158, .T. ) ;
#14701=LINE ( 'NONE', #7437, #3113 ) ;
#14703=FACE_OUTER_BOUND ( 'NONE', #5323, .T. ) ;
#14706=VERTEX_POINT ( 'NONE', #19365 ) ;
#14707=CIRCLE ( 'NONE', #6113, 3.606799999998994366 ) ;
#14709=CARTESIAN_POINT ( 'NONE',  ( 151.4000000000000057, -3544.570000000000164, 2240.279999999999745 ) ) ;
#14714=PLANE ( 'NONE',  #242 ) ;
#14716=AXIS2_PLACEMENT_3D ( 'NONE', #17744, #17626, #8616 ) ;
#14718=DIRECTION ( 'NONE',  ( 0.000000000000000000, 0.000000000000000000, 1.000000000000000000 ) ) ;
#14722=EDGE_CURVE ( 'NONE', #7066, #7103, #10218, .T. ) ;
#14724=CARTESIAN_POINT ( 'NONE',  ( 18.17671024882161035, -3657.870959520586439, 2245.673873547450057 ) ) ;
#14725=VERTEX_POINT ( 'NONE', #9399 ) ;
#14726=CARTESIAN_POINT ( 'NONE',  ( 147.5974422321679072, -3695.562642951958424, 2259.905235783985518 ) ) ;
#14727=CARTESIAN_POINT ( 'NONE',  ( 127.0000000000000000, -3568.700000000000273, 2260.600000000000364 ) ) ;
#14729=DIRECTION ( 'NONE',  ( 0.000000000000000000, 0.000000000000000000, 1.000000000000000000 ) ) ;
#14730=CARTESIAN_POINT ( 'NONE',  ( 127.0000000000000000, -3568.700000000000273, 2261.869999999999891 ) ) ;
#14733=CARTESIAN_POINT ( 'NONE',  ( 7.036241622171066190, -3578.717921621798268, 2244.547188460646794 ) ) ;
#14736=ORIENTED_EDGE ( 'NONE', *, *, #16840, .F. ) ;
#14737=CARTESIAN_POINT ( 'NONE',  ( 132.0583097651000060, -3544.202533098000458, 2260.545675974999995 ) ) ;
#14739=AXIS2_PLACEMENT_3D ( 'NONE', #8153, #20672, #10130 ) ;
#14740=ADVANCED_FACE ( 'NONE', ( #2137 ), #14788, .F. ) ;
#14741=DIRECTION ( 'NONE',  ( 0.000000000000000000, 0.000000000000000000, 1.000000000000000000 ) ) ;
#14742=DIRECTION ( 'NONE',  ( 0.000000000000000000, 0.000000000000000000, -1.000000000000000000 ) ) ;
#14743=DIRECTION ( 'NONE',  ( 0.000000000000000000, 0.000000000000000000, 1.000000000000000000 ) ) ;
#14745=VERTEX_POINT ( 'NONE', #10916 ) ;
#14748=DIRECTION ( 'NONE',  ( -1.000000000000000000, 0.000000000000000000, 0.000000000000000000 ) ) ;
#14751=ORIENTED_EDGE ( 'NONE', *, *, #11693, .T. ) ;
#14752=CARTESIAN_POINT ( 'NONE',  ( 12.69999999999999929, -3579.494999999999891, 2239.771999999999935 ) ) ;
#14753=TOROIDAL_SURFACE ( 'NONE', #8761, 3.606799999999999784, 0.7620000000000000107 ) ;
#14757=DIRECTION ( 'NONE',  ( 0.000000000000000000, 0.000000000000000000, -1.000000000000000000 ) ) ;
#14759=CARTESIAN_POINT ( 'NONE',  ( 137.5719038287758451, -3581.382881717005603, 2248.706519082991235 ) ) ;
#14760=EDGE_LOOP ( 'NONE', ( #3177, #13768, #11948, #15756 ) ) ;
#14761=CARTESIAN_POINT ( 'NONE',  ( 145.2613662610192193, -3580.811168667689344, 2245.321774183717480 ) ) ;
#14763=ADVANCED_FACE ( 'NONE', ( #4006 ), #20068, .T. ) ;
#14764=CARTESIAN_POINT ( 'NONE',  ( 145.3808575608765068, -3578.871194572863715, 2244.547198930070408 ) ) ;
#14766=TOROIDAL_SURFACE ( 'NONE', #18500, 3.606799999999999784, 0.7620000000000000107 ) ;
#14767=CARTESIAN_POINT ( 'NONE',  ( 1.270000000000000018, -3544.570000000000164, 2239.009999999999764 ) ) ;
#14769=FACE_OUTER_BOUND ( 'NONE', #1744, .T. ) ;
#14770=AXIS2_PLACEMENT_3D ( 'NONE', #21865, #19773, #5826 ) ;
#14771=CARTESIAN_POINT ( 'NONE',  ( 138.6135835479743434, -3576.865461055983360, 2249.420587708207222 ) ) ;
#14776=CARTESIAN_POINT ( 'NONE',  ( 15.28733791996542735, -3543.933445093964110, 2255.655544454380106 ) ) ;
#14779=DIRECTION ( 'NONE',  ( -1.000000000000000000, 0.000000000000000000, 0.000000000000000000 ) ) ;
#14780=CIRCLE ( 'NONE', #21523, 0.7619999999999294005 ) ;
#14781=CARTESIAN_POINT ( 'NONE',  ( 135.5205845993333185, -3581.600849088022642, 2246.630007010045119 ) ) ;
#14783=ORIENTED_EDGE ( 'NONE', *, *, #3770, .F. ) ;
#14784=AXIS2_PLACEMENT_3D ( 'NONE', #7561, #21745, #3928 ) ;
#14786=CARTESIAN_POINT ( 'NONE',  ( 12.22806302161694347, -3576.688821853146237, 2249.230233872227018 ) ) ;
#14788=CYLINDRICAL_SURFACE ( 'NONE', #7992, 2.844800000000001550 ) ;
#14793=DIRECTION ( 'NONE',  ( 0.000000000000000000, 0.000000000000000000, -1.000000000000000000 ) ) ;
#14794=ORIENTED_EDGE ( 'NONE', *, *, #1830, .F. ) ;
#14796=CARTESIAN_POINT ( 'NONE',  ( 130.6067999999989979, -3568.700000000000273, 2259.837999999999738 ) ) ;
#14798=ORIENTED_EDGE ( 'NONE', *, *, #18689, .T. ) ;
#14800=CARTESIAN_POINT ( 'NONE',  ( 138.8666558583366566, -3662.225077533978492, 2249.327302760020757 ) ) ;
#14801=VECTOR ( 'NONE', #1619, 1000.000000000000000 ) ;
#14807=ADVANCED_FACE ( 'NONE', ( #12563, #11154, #2017 ), #18294, .T. ) ;
#14808=ORIENTED_EDGE ( 'NONE', *, *, #22463, .T. ) ;
#14816=CARTESIAN_POINT ( 'NONE',  ( 7.144342338834939632, -3580.833646875532850, 2245.342901023110699 ) ) ;
#14817=EDGE_CURVE ( 'NONE', #2318, #2712, #16196, .T. ) ;
#14822=AXIS2_PLACEMENT_3D ( 'NONE', #445, #104, #14748 ) ;
#14823=CARTESIAN_POINT ( 'NONE',  ( 142.2400000000000091, -3580.776127254000130, 2255.774000000000342 ) ) ;
#14824=VERTEX_POINT ( 'NONE', #18067 ) ;
#14825=CARTESIAN_POINT ( 'NONE',  ( 142.4504371321982887, -3658.772581173975141, 2249.888537610986077 ) ) ;
#14827=ADVANCED_FACE ( 'NONE', ( #9168 ), #5893, .F. ) ;
#14828=ORIENTED_EDGE ( 'NONE', *, *, #17721, .T. ) ;
#14830=CIRCLE ( 'NONE', #7716, 2.844800000000091700 ) ;
#14831=EDGE_CURVE ( 'NONE', #4249, #19682, #6828, .T. ) ;
#14833=LINE ( 'NONE', #20216, #10658 ) ;
#14835=AXIS2_PLACEMENT_3D ( 'NONE', #5321, #12466, #3552 ) ;
#14839=CIRCLE ( 'NONE', #18568, 2.844799999999994444 ) ;
#14840=CARTESIAN_POINT ( 'NONE',  ( 151.1299999999999955, -3694.430000000000291, 2260.600000000000364 ) ) ;
#14841=ORIENTED_EDGE ( 'NONE', *, *, #3083, .F. ) ;
#14842=DIRECTION ( 'NONE',  ( 1.224646799147353207E-16, 1.000000000000000000, -0.000000000000000000 ) ) ;
#14843=CARTESIAN_POINT ( 'NONE',  ( 98.75520000000000209, -3619.500000000000000, 2239.771999999999935 ) ) ;
#14847=CARTESIAN_POINT ( 'NONE',  ( 142.3029786115121453, -3543.951823054115266, 2255.616427089806621 ) ) ;
#14848=AXIS2_PLACEMENT_3D ( 'NONE', #8481, #10223, #1434 ) ;
#14850=DIRECTION ( 'NONE',  ( 1.000000000000000000, 0.000000000000000000, 0.000000000000000000 ) ) ;
#14854=DIRECTION ( 'NONE',  ( -1.224646799147353207E-16, 1.000000000000000000, 0.000000000000000000 ) ) ;
#14855=EDGE_CURVE ( 'NONE', #1443, #15832, #17634, .T. ) ;
#14856=CYLINDRICAL_SURFACE ( 'NONE', #9081, 2.844799999998995244 ) ;
#14858=CYLINDRICAL_SURFACE ( 'NONE', #8989, 2.844800000000091700 ) ;
#14859=AXIS2_PLACEMENT_3D ( 'NONE', #14653, #2229, #16510 ) ;
#14862=ORIENTED_EDGE ( 'NONE', *, *, #22015, .T. ) ;
#14864=CARTESIAN_POINT ( 'NONE',  ( 14.11996008720290874, -3661.970800930585483, 2249.569598517611666 ) ) ;
#14865=DIRECTION ( 'NONE',  ( 0.000000000000000000, 0.000000000000000000, 1.000000000000000000 ) ) ;
#14866=ORIENTED_EDGE ( 'NONE', *, *, #13235, .F. ) ;
#14870=VECTOR ( 'NONE', #15497, 1000.000000000000000 ) ;
#14871=ORIENTED_EDGE ( 'NONE', *, *, #9797, .F. ) ;
#14872=CARTESIAN_POINT ( 'NONE',  ( 116.8400000000000034, -3695.699999999999818, 2251.506800000000112 ) ) ;
#14874=ORIENTED_EDGE ( 'NONE', *, *, #2965, .T. ) ;
#14879=CARTESIAN_POINT ( 'NONE',  ( 145.3458854616064286, -3580.386202657235117, 2244.987819353762006 ) ) ;
#14883=ADVANCED_FACE ( 'NONE', ( #4804 ), #10310, .T. ) ;
#14886=CARTESIAN_POINT ( 'NONE',  ( 18.17520605051544891, -3661.148255213616721, 2244.728530265969766 ) ) ;
#14887=FACE_OUTER_BOUND ( 'NONE', #10708, .T. ) ;
#14890=CARTESIAN_POINT ( 'NONE',  ( 141.5683389801453416, -3577.348789367103109, 2249.802649695933724 ) ) ;
#14891=EDGE_CURVE ( 'NONE', #21069, #21998, #8436, .T. ) ;
#14892=VERTEX_POINT ( 'NONE', #13721 ) ;
#14893=AXIS2_PLACEMENT_3D ( 'NONE', #7697, #2540, #21992 ) ;
#14894=ORIENTED_EDGE ( 'NONE', *, *, #5955, .T. ) ;
#14895=DIRECTION ( 'NONE',  ( 0.000000000000000000, -1.000000000000000000, 1.319970543219000025E-14 ) ) ;
#14897=DIRECTION ( 'NONE',  ( 0.000000000000000000, 0.000000000000000000, -1.000000000000000000 ) ) ;
#14898=DIRECTION ( 'NONE',  ( 0.000000000000000000, 1.000000000000000000, 0.000000000000000000 ) ) ;
#14902=CARTESIAN_POINT ( 'NONE',  ( 141.6126318482000102, -3581.600863517000107, 2246.630000000000109 ) ) ;
#14906=CARTESIAN_POINT ( 'NONE',  ( 15.17514636921737647, -3578.092538392563711, 2250.131376828858265 ) ) ;
#14907=CARTESIAN_POINT ( 'NONE',  ( 142.4529136091622092, -3580.215257529047449, 2249.894017841437289 ) ) ;
#14909=B_SPLINE_CURVE_WITH_KNOTS ( 'NONE', 3,
 ( #1934, #23016, #1700, #12483 ),
 .UNSPECIFIED., .F., .F.,
 ( 4, 4 ),
 ( 0.000000000000000000, 1.000000000000000000 ),
 .UNSPECIFIED. ) ;
#14910=CARTESIAN_POINT ( 'NONE',  ( 25.39999999999999858, -3578.860000000000127, 2244.547199999999975 ) ) ;
#14912=CARTESIAN_POINT ( 'NONE',  ( 20.34169023495000062, -3694.797466901999996, 2260.545675974999995 ) ) ;
#14913=CARTESIAN_POINT ( 'NONE',  ( 38.10000000000000142, -3594.099999999999909, 2259.837999999999738 ) ) ;
#14914=CARTESIAN_POINT ( 'NONE',  ( 20.79047621426877512, -3543.300000000000637, 2259.421674283870743 ) ) ;
#14915=DIRECTION ( 'NONE',  ( 0.000000000000000000, 1.000000000000000000, 0.000000000000000000 ) ) ;
#14918=CARTESIAN_POINT ( 'NONE',  ( 141.8261614683892162, -3661.395196750292598, 2249.944974537677354 ) ) ;
#14919=ORIENTED_EDGE ( 'NONE', *, *, #1766, .F. ) ;
#14920=ORIENTED_EDGE ( 'NONE', *, *, #19987, .T. ) ;
#14921=DIRECTION ( 'NONE',  ( 0.000000000000000000, 0.000000000000000000, -1.000000000000000000 ) ) ;
#14922=ORIENTED_EDGE ( 'NONE', *, *, #9851, .F. ) ;
#14925=DIRECTION ( 'NONE',  ( 0.000000000000000000, 0.000000000000000000, 1.000000000000000000 ) ) ;
#14926=VERTEX_POINT ( 'NONE', #22951 ) ;
#14927=CARTESIAN_POINT ( 'NONE',  ( 7.269937948888002488, -3657.722882969321745, 2245.891767160526342 ) ) ;
#14928=FACE_OUTER_BOUND ( 'NONE', #1296, .T. ) ;
#14929=CARTESIAN_POINT ( 'NONE',  ( 53.64479999999999649, -3670.300000000000182, 2259.837999999999738 ) ) ;
#14933=VERTEX_POINT ( 'NONE', #20979 ) ;
#14938=DIRECTION ( 'NONE',  ( 1.000000000000000000, 0.000000000000000000, 0.000000000000000000 ) ) ;
#14939=EDGE_CURVE ( 'NONE', #12111, #16761, #1630, .T. ) ;
#14944=AXIS2_PLACEMENT_3D ( 'NONE', #6405, #13786, #9683 ) ;
#14945=ADVANCED_FACE ( 'NONE', ( #6918 ), #12307, .T. ) ;
#14946=DIRECTION ( 'NONE',  ( -1.000000000000000000, 0.000000000000000000, 0.000000000000000000 ) ) ;
#14954=DIRECTION ( 'NONE',  ( 0.000000000000000000, 0.000000000000000000, 1.000000000000000000 ) ) ;
#14955=EDGE_CURVE ( 'NONE', #17874, #13993, #3391, .T. ) ;
#14956=CARTESIAN_POINT ( 'NONE',  ( 29.00679999999900005, -3568.700000000000273, 2239.771999999999935 ) ) ;
#14958=ORIENTED_EDGE ( 'NONE', *, *, #8169, .F. ) ;
#14961=FACE_OUTER_BOUND ( 'NONE', #7524, .T. ) ;
#14968=DIRECTION ( 'NONE',  ( -1.000000000000000000, 0.000000000000000000, 0.000000000000000000 ) ) ;
#14970=CARTESIAN_POINT ( 'NONE',  ( 127.0000000000000000, -3578.860000000000127, 2244.547199999999975 ) ) ;
#14972=CARTESIAN_POINT ( 'NONE',  ( 14.45367585492360085, -3661.745009548058079, 2249.740799630053516 ) ) ;
#14973=EDGE_CURVE ( 'NONE', #10545, #8337, #9450, .T. ) ;
#14975=ORIENTED_EDGE ( 'NONE', *, *, #16709, .T. ) ;
#14976=DIRECTION ( 'NONE',  ( 1.000000000000000000, 0.000000000000000000, 0.000000000000000000 ) ) ;
#14977=DIRECTION ( 'NONE',  ( 0.000000000000000000, -1.000000000000000000, 0.000000000000000000 ) ) ;
#14979=CARTESIAN_POINT ( 'NONE',  ( 10.16000000000000014, -3694.430000000000291, 2255.774000000000342 ) ) ;
#14980=DIRECTION ( 'NONE',  ( -1.000000000000000000, 0.000000000000000000, 0.000000000000000000 ) ) ;
#14983=EDGE_LOOP ( 'NONE', ( #8328, #4935, #20144, #17537 ) ) ;
#14985=DIRECTION ( 'NONE',  ( 0.7249994335945011414, 0.000000000000000000, -0.6887494619146010688 ) ) ;
#14986=EDGE_CURVE ( 'NONE', #22471, #10418, #15398, .T. ) ;
#14988=CARTESIAN_POINT ( 'NONE',  ( 145.1629702012129144, -3581.174070081973241, 2245.736054072267962 ) ) ;
#14989=SHAPE_DEFINITION_REPRESENTATION ( #8109, #7730 ) ;
#14991=CARTESIAN_POINT ( 'NONE',  ( 17.78929153062866320, -3662.104870690277039, 2245.334605559830379 ) ) ;
#14994=CARTESIAN_POINT ( 'NONE',  ( 151.4000000000000057, -3543.329032635400836, 2260.600000000000364 ) ) ;
#14996=CARTESIAN_POINT ( 'NONE',  ( 137.5725893229727603, -3577.606221452492264, 2249.945671348400538 ) ) ;
#14997=ORIENTED_EDGE ( 'NONE', *, *, #1771, .T. ) ;
#15000=CIRCLE ( 'NONE', #22941, 0.7619999999999294005 ) ;
#15001=DIRECTION ( 'NONE',  ( 1.000000000000000000, 0.000000000000000000, 0.000000000000000000 ) ) ;
#15002=ORIENTED_EDGE ( 'NONE', *, *, #2131, .F. ) ;
#15007=AXIS2_PLACEMENT_3D ( 'NONE', #10938, #2271, #20196 ) ;
#15008=ADVANCED_FACE ( 'NONE', ( #2221 ), #2338, .T. ) ;
#15014=CARTESIAN_POINT ( 'NONE',  ( 14.97319837854892377, -3577.784037172878925, 2250.025725775317824 ) ) ;
#15016=CARTESIAN_POINT ( 'NONE',  ( 141.7599675853109886, -3581.457171778321481, 2248.553155654074999 ) ) ;
#15020=DIRECTION ( 'NONE',  ( -1.000000000000000000, 0.000000000000000000, 0.000000000000000000 ) ) ;
#15022=FACE_OUTER_BOUND ( 'NONE', #10590, .T. ) ;
#15023=ORIENTED_EDGE ( 'NONE', *, *, #7701, .F. ) ;
#15025=VECTOR ( 'NONE', #1107, 1000.000000000000000 ) ;
#15028=VECTOR ( 'NONE', #262, 1000.000000000000000 ) ;
#15030=ORIENTED_EDGE ( 'NONE', *, *, #22397, .F. ) ;
#15032=VERTEX_POINT ( 'NONE', #2331 ) ;
#15034=ADVANCED_FACE ( 'NONE', ( #16740 ), #5000, .T. ) ;
#15036=ORIENTED_EDGE ( 'NONE', *, *, #1029, .T. ) ;
#15038=DIRECTION ( 'NONE',  ( -0.000000000000000000, -1.000000000000000000, -0.000000000000000000 ) ) ;
#15041=CARTESIAN_POINT ( 'NONE',  ( 7.236841730867277889, -3657.826545604375497, 2245.735190626965050 ) ) ;
#15047=ORIENTED_EDGE ( 'NONE', *, *, #1195, .F. ) ;
#15049=EDGE_CURVE ( 'NONE', #6309, #5839, #9922, .T. ) ;
#15050=DIRECTION ( 'NONE',  ( 1.000000000000000000, 0.000000000000000000, -2.331176954593999892E-13 ) ) ;
#15051=CARTESIAN_POINT ( 'NONE',  ( 127.0000000000000000, -3578.860000000000127, 2244.547199999999975 ) ) ;
#15052=VECTOR ( 'NONE', #5167, 1000.000000000000000 ) ;
#15054=AXIS2_PLACEMENT_3D ( 'NONE', #3767, #1791, #9051 ) ;
#15056=TOROIDAL_SURFACE ( 'NONE', #13171, 4.114799999999999791, 1.270000000000000018 ) ;
#15059=CARTESIAN_POINT ( 'NONE',  ( 0.000000000000000000, -3694.430000000000291, 2240.279999999999745 ) ) ;
#15060=CARTESIAN_POINT ( 'NONE',  ( 18.36215345614126093, -3658.729285337897181, 2244.921339882903339 ) ) ;
#15062=VERTEX_POINT ( 'NONE', #20708 ) ;
#15063=DIRECTION ( 'NONE',  ( 0.000000000000000000, 0.000000000000000000, -1.000000000000000000 ) ) ;
#15069=VECTOR ( 'NONE', #6896, 1000.000000000000000 ) ;
#15070=AXIS2_PLACEMENT_3D ( 'NONE', #14730, #5832, #12967 ) ;
#15071=CARTESIAN_POINT ( 'NONE',  ( 8.088613972650000150, -3576.119152860999748, 2246.630000000000109 ) ) ;
#15075=DIRECTION ( 'NONE',  ( 0.000000000000000000, 0.000000000000000000, -1.000000000000000000 ) ) ;
#15080=B_SPLINE_CURVE_WITH_KNOTS ( 'NONE', 3,
 ( #18509, #5535, #9608, #19932 ),
 .UNSPECIFIED., .F., .F.,
 ( 4, 4 ),
 ( 0.000000000000000000, 1.000000000000000000 ),
 .UNSPECIFIED. ) ;
#15082=CARTESIAN_POINT ( 'NONE',  ( 134.8439533950256930, -3576.481706514296548, 2245.831027411355080 ) ) ;
#15087=AXIS2_PLACEMENT_3D ( 'NONE', #5773, #12787, #2015 ) ;
#15090=DIRECTION ( 'NONE',  ( 0.000000000000000000, 0.000000000000000000, 1.000000000000000000 ) ) ;
#15093=CARTESIAN_POINT ( 'NONE',  ( 12.69999999999999929, -3659.504999999999654, 2246.630000000000109 ) ) ;
#15094=DIRECTION ( 'NONE',  ( 0.000000000000000000, -1.000000000000000000, 0.000000000000000000 ) ) ;
#15095=VERTEX_POINT ( 'NONE', #7726 ) ;
#15098=EDGE_CURVE ( 'NONE', #7121, #20865, #22344, .T. ) ;
#15104=CARTESIAN_POINT ( 'NONE',  ( 145.2911534367045192, -3580.678095346821920, 2245.203709730261835 ) ) ;
#15107=CARTESIAN_POINT ( 'NONE',  ( 145.4149999194000316, -3579.495498070999474, 2244.618783703000190 ) ) ;
#15108=CARTESIAN_POINT ( 'NONE',  ( 17.36210096838674133, -3662.811570847525218, 2246.380819257733037 ) ) ;
#15110=CARTESIAN_POINT ( 'NONE',  ( 137.5890733217894706, -3577.587789889484611, 2249.936548038443561 ) ) ;
#15112=ORIENTED_EDGE ( 'NONE', *, *, #6732, .T. ) ;
#15113=AXIS2_PLACEMENT_3D ( 'NONE', #1413, #23078, #22961 ) ;
#15114=CARTESIAN_POINT ( 'NONE',  ( 7.276091043450246154, -3657.704285925716249, 2245.922240752401649 ) ) ;
#15115=LINE ( 'NONE', #6214, #7681 ) ;
#15119=CARTESIAN_POINT ( 'NONE',  ( 10.90808957415271685, -3657.295456685377758, 2247.303068057902237 ) ) ;
#15121=ORIENTED_EDGE ( 'NONE', *, *, #17836, .T. ) ;
#15122=ORIENTED_EDGE ( 'NONE', *, *, #19769, .F. ) ;
#15126=CARTESIAN_POINT ( 'NONE',  ( 11.73013214837809848, -3576.819306460322423, 2249.374504195262489 ) ) ;
#15128=CARTESIAN_POINT ( 'NONE',  ( 141.8118641587357160, -3581.401022134622963, 2248.671103578885777 ) ) ;
#15129=ORIENTED_EDGE ( 'NONE', *, *, #17133, .T. ) ;
#15131=VECTOR ( 'NONE', #20493, 1000.000000000000000 ) ;
#15134=AXIS2_PLACEMENT_3D ( 'NONE', #23033, #17294, #20940 ) ;
#15135=DIRECTION ( 'NONE',  ( -1.000000000000000000, 0.000000000000000000, 0.000000000000000000 ) ) ;
#15138=EDGE_CURVE ( 'NONE', #3669, #159, #18835, .T. ) ;
#15140=CARTESIAN_POINT ( 'NONE',  ( 79.04479999999999507, -3670.300000000000182, 2239.771999999999935 ) ) ;
#15141=ORIENTED_EDGE ( 'NONE', *, *, #19029, .T. ) ;
#15144=AXIS2_PLACEMENT_3D ( 'NONE', #8370, #8251, #7278 ) ;
#15146=CIRCLE ( 'NONE', #9539, 3.606799999999993567 ) ;
#15152=CARTESIAN_POINT ( 'NONE',  ( 7.137204922041744837, -3658.194885328095097, 2245.316081567704714 ) ) ;
#15154=CARTESIAN_POINT ( 'NONE',  ( 151.1299999999999955, -3544.570000000000164, 2239.009999999999764 ) ) ;
#15155=CARTESIAN_POINT ( 'NONE',  ( 151.1299999999999955, -3578.860000000000127, 2243.277199999999993 ) ) ;
#15165=CARTESIAN_POINT ( 'NONE',  ( 1.270000000000000018, -3660.140000000000327, 2247.392000000000280 ) ) ;
#15167=EDGE_LOOP ( 'NONE', ( #3798, #21862, #14920, #21049 ) ) ;
#15168=CARTESIAN_POINT ( 'NONE',  ( 136.8826269810293468, -3543.437357048151625, 2255.079208148982161 ) ) ;
#15172=ORIENTED_EDGE ( 'NONE', *, *, #7774, .F. ) ;
#15173=EDGE_LOOP ( 'NONE', ( #17928, #11429, #7727, #7786 ) ) ;
#15175=AXIS2_PLACEMENT_3D ( 'NONE', #6600, #13739, #11856 ) ;
#15178=CIRCLE ( 'NONE', #5079, 2.844800000000091700 ) ;
#15179=CYLINDRICAL_SURFACE ( 'NONE', #5492, 1.269999999999898099 ) ;
#15180=EDGE_CURVE ( 'NONE', #3518, #10484, #19182, .T. ) ;
#15183=CARTESIAN_POINT ( 'NONE',  ( 101.5999999999999943, -3568.700000000000273, 2239.009999999999764 ) ) ;
#15184=CARTESIAN_POINT ( 'NONE',  ( 88.90000000000000568, -3644.899999999999636, 2260.600000000000364 ) ) ;
#15188=EDGE_LOOP ( 'NONE', ( #21469, #11731, #4798, #3361 ) ) ;
#15189=DIRECTION ( 'NONE',  ( -1.000000000000000000, 0.000000000000000000, 0.000000000000000000 ) ) ;
#15192=AXIS2_PLACEMENT_3D ( 'NONE', #13072, #14729, #427 ) ;
#15195=CARTESIAN_POINT ( 'NONE',  ( 22.55520000000100111, -3568.700000000000273, 2239.771999999999935 ) ) ;
#15196=VECTOR ( 'NONE', #1608, 1000.000000000000000 ) ;
#15200=CARTESIAN_POINT ( 'NONE',  ( 15.54479999999932716, -3579.043785370524802, 2256.063560000000962 ) ) ;
#15201=AXIS2_PLACEMENT_3D ( 'NONE', #10258, #1002, #22435 ) ;
#15202=CARTESIAN_POINT ( 'NONE',  ( 14.93865131287260084, -3661.261308499835195, 2250.006918105073510 ) ) ;
#15204=AXIS2_PLACEMENT_3D ( 'NONE', #1159, #4802, #17450 ) ;
#15205=ORIENTED_EDGE ( 'NONE', *, *, #837, .F. ) ;
#15210=B_SPLINE_CURVE_WITH_KNOTS ( 'NONE', 3,
 ( #12417, #1752, #7042, #3499, #9135 ),
 .UNSPECIFIED., .F., .F.,
 ( 4, 1, 4 ),
 ( 0.000000000000000000, 0.5000000000000000000, 1.000000000000000000 ),
 .UNSPECIFIED. ) ;
#15215=ORIENTED_EDGE ( 'NONE', *, *, #3482, .F. ) ;
#15217=CARTESIAN_POINT ( 'NONE',  ( 145.0360689528194484, -3581.542328872695180, 2246.419514930312289 ) ) ;
#15219=FACE_OUTER_BOUND ( 'NONE', #15266, .T. ) ;
#15220=CARTESIAN_POINT ( 'NONE',  ( 17.56415751376727741, -3662.505169287860099, 2245.811216528392379 ) ) ;
#15223=DIRECTION ( 'NONE',  ( -1.000000000000000000, 0.000000000000000000, 0.000000000000000000 ) ) ;
#15227=CARTESIAN_POINT ( 'NONE',  ( 151.1299999999999955, -3660.140000000000327, 2251.506800000000112 ) ) ;
#15231=VERTEX_POINT ( 'NONE', #1251 ) ;
#15236=CARTESIAN_POINT ( 'NONE',  ( 142.2400000000000091, -3658.223872745999870, 2255.774000000000342 ) ) ;
#15239=VERTEX_POINT ( 'NONE', #22575 ) ;
#15243=CARTESIAN_POINT ( 'NONE',  ( 85.29320000000001301, -3644.899999999999636, 2259.837999999999738 ) ) ;
#15244=CARTESIAN_POINT ( 'NONE',  ( 10.88249034213936994, -3577.304564350549299, 2249.774856120668119 ) ) ;
#15246=EDGE_CURVE ( 'NONE', #4022, #9982, #9086, .T. ) ;
#15251=CIRCLE ( 'NONE', #13746, 0.7619999999999294005 ) ;
#15254=EDGE_CURVE ( 'NONE', #4127, #6665, #22919, .T. ) ;
#15255=TOROIDAL_SURFACE ( 'NONE', #17113, 3.606799999998999695, 0.7620000000000000107 ) ;
#15256=CARTESIAN_POINT ( 'NONE',  ( 146.1770000000009873, -3579.494999999999891, 2239.771999999999935 ) ) ;
#15258=VERTEX_POINT ( 'NONE', #13684 ) ;
#15262=ADVANCED_FACE ( 'NONE', ( #17302 ), #10190, .T. ) ;
#15265=DIRECTION ( 'NONE',  ( 0.000000000000000000, 0.000000000000000000, -1.000000000000000000 ) ) ;
#15266=EDGE_LOOP ( 'NONE', ( #11761, #6111, #21798, #17512 ) ) ;
#15269=ORIENTED_EDGE ( 'NONE', *, *, #3420, .T. ) ;
#15270=VECTOR ( 'NONE', #15943, 1000.000000000000000 ) ;
#15271=FACE_OUTER_BOUND ( 'NONE', #4315, .T. ) ;
#15273=DIRECTION ( 'NONE',  ( 0.000000000000000000, 0.000000000000000000, 1.000000000000000000 ) ) ;
#15276=CYLINDRICAL_SURFACE ( 'NONE', #3805, 2.844799999999009010 ) ;
#15281=DIRECTION ( 'NONE',  ( -1.000000000000000000, 0.000000000000000000, 0.000000000000000000 ) ) ;
#15283=CARTESIAN_POINT ( 'NONE',  ( 137.0372476977747738, -3543.741058433492071, 2255.466570801807393 ) ) ;
#15286=DIRECTION ( 'NONE',  ( 1.000000000000000000, 0.000000000000000000, 0.000000000000000000 ) ) ;
#15287=CARTESIAN_POINT ( 'NONE',  ( 18.40115537325064210, -3659.045393564460937, 2244.753257970025970 ) ) ;
#15289=EDGE_LOOP ( 'NONE', ( #21465, #4475, #21159, #2109 ) ) ;
#15290=DIRECTION ( 'NONE',  ( 0.000000000000000000, 0.000000000000000000, 1.000000000000000000 ) ) ;
#15291=DIRECTION ( 'NONE',  ( 0.000000000000000000, 0.000000000000000000, 1.000000000000000000 ) ) ;
#15293=EDGE_CURVE ( 'NONE', #2027, #18714, #4958, .T. ) ;
#15298=TOROIDAL_SURFACE ( 'NONE', #10814, 3.606799999999999784, 0.7620000000000000107 ) ;
#15300=ORIENTED_EDGE ( 'NONE', *, *, #17396, .T. ) ;
#15303=ORIENTED_EDGE ( 'NONE', *, *, #23023, .F. ) ;
#15312=CARTESIAN_POINT ( 'NONE',  ( 144.5381749684807744, -3662.547005267768327, 2245.875428656603162 ) ) ;
#15313=VERTEX_POINT ( 'NONE', #9115 ) ;
#15316=DIRECTION ( 'NONE',  ( 0.000000000000000000, -1.000000000000000000, 0.000000000000000000 ) ) ;
#15318=EDGE_LOOP ( 'NONE', ( #18198, #9174, #9489, #11245 ) ) ;
#15319=DIRECTION ( 'NONE',  ( 0.000000000000000000, 0.000000000000000000, -1.000000000000000000 ) ) ;
#15325=ORIENTED_EDGE ( 'NONE', *, *, #13156, .T. ) ;
#15326=ORIENTED_EDGE ( 'NONE', *, *, #4840, .T. ) ;
#15327=CIRCLE ( 'NONE', #18318, 2.844800000000091700 ) ;
#15332=DIRECTION ( 'NONE',  ( 1.122008997397786234E-13, 0.000000000000000000, 1.000000000000000000 ) ) ;
#15335=FACE_OUTER_BOUND ( 'NONE', #22118, .T. ) ;
#15336=CARTESIAN_POINT ( 'NONE',  ( 9.652920519510999497, -3695.699999999999818, 2254.503999999999905 ) ) ;
#15339=TOROIDAL_SURFACE ( 'NONE', #16096, 3.606799999998999695, 0.7620000000000000107 ) ;
#15342=VERTEX_POINT ( 'NONE', #12738 ) ;
#15344=CARTESIAN_POINT ( 'NONE',  ( 12.69999999999999929, -3659.504999999999654, 2246.630000000000109 ) ) ;
#15345=CARTESIAN_POINT ( 'NONE',  ( 10.57779571310348565, -3657.610496412460179, 2248.693734300258257 ) ) ;
#15346=ORIENTED_EDGE ( 'NONE', *, *, #20749, .T. ) ;
#15347=ORIENTED_EDGE ( 'NONE', *, *, #22284, .T. ) ;
#15349=DIRECTION ( 'NONE',  ( 1.000000000000000000, 0.000000000000000000, 0.000000000000000000 ) ) ;
#15350=ORIENTED_EDGE ( 'NONE', *, *, #22397, .T. ) ;
#15352=CARTESIAN_POINT ( 'NONE',  ( 76.20000000000000284, -3568.700000000000273, 2260.600000000000364 ) ) ;
#15353=DIRECTION ( 'NONE',  ( 1.000000000000000000, 0.000000000000000000, 0.000000000000000000 ) ) ;
#15355=CARTESIAN_POINT ( 'NONE',  ( 142.4352164564301688, -3580.278531256406040, 2249.858390971456629 ) ) ;
#15356=ORIENTED_EDGE ( 'NONE', *, *, #12385, .T. ) ;
#15361=LINE ( 'NONE', #11718, #21988 ) ;
#15363=CARTESIAN_POINT ( 'NONE',  ( 129.8447999999989975, -3619.500000000000000, 2261.869999999999891 ) ) ;
#15366=CARTESIAN_POINT ( 'NONE',  ( 134.2006755046125761, -3657.949543878901750, 2245.576349614068477 ) ) ;
#15370=ORIENTED_EDGE ( 'NONE', *, *, #18162, .T. ) ;
#15372=DIRECTION ( 'NONE',  ( 0.000000000000000000, 0.000000000000000000, -1.000000000000000000 ) ) ;
#15376=DIRECTION ( 'NONE',  ( 0.000000000000000000, 0.000000000000000000, 1.000000000000000000 ) ) ;
#15378=VERTEX_POINT ( 'NONE', #20012 ) ;
#15382=FACE_OUTER_BOUND ( 'NONE', #2248, .T. ) ;
#15384=AXIS2_PLACEMENT_3D ( 'NONE', #7455, #18229, #5939 ) ;
#15390=EDGE_CURVE ( 'NONE', #22006, #13646, #3034, .T. ) ;
#15391=EDGE_CURVE ( 'NONE', #17959, #9684, #10902, .T. ) ;
#15393=FACE_OUTER_BOUND ( 'NONE', #5592, .T. ) ;
#15398=B_SPLINE_CURVE_WITH_KNOTS ( 'NONE', 3,
 ( #5041, #12419, #3503, #10654, #17804, #8326, #14298, #17916, #2, #16050, #2111, #7380, #117, #11004, #12649, #7487, #21443, #7150, #5519, #19800, #10773, #9257, #18038, #14645, #1756, #5393, #3734, #12531, #19688, #3622, #18148, #19916, #11127, #12763, #14759, #14534, #1868, #12881, #7263, #9020, #16393, #344, #239, #10889, #21671, #3856, #1987, #21785, #456, #5627, #14412, #16166, #9139, #5747, #9368, #16279, #20034 ),
 .UNSPECIFIED., .F., .F.,
 ( 4, 2, 2, 1, 1, 2, 2, 2, 2, 1, 1, 1, 2, 2, 2, 2, 2, 2, 1, 1, 2, 2, 2, 2, 2, 2, 2, 2, 2, 2, 2, 4 ),
 ( 0.000000000000000000, 0.1249999999985798027, 0.1874999999980038745, 0.2187499999977179366, 0.2343749999975340836, 0.2421874999975122955, 0.2499999999974905074, 0.3124999999980864751, 0.3437499999984656163, 0.3593749999987312926, 0.3671874999987232990, 0.3710937499987121968, 0.3730468749987710386, 0.3749999999988298249, 0.4062499999969994557, 0.4374999999951690866, 0.4687499999933387174, 0.4843749999924235050, 0.4921874999918540161, 0.4960937499915020199, 0.4980468749914571114, 0.4999999999914122029, 0.5624999999926729721, 0.5937499999933033568, 0.6093749999936185491, 0.6249999999939337414, 0.6874999999948844254, 0.7499999999958351093, 0.8124999999967857933, 0.8437499999972610798, 0.8749999999977363663, 1.000000000000000000 ),
 .UNSPECIFIED. ) ;
#15399=EDGE_LOOP ( 'NONE', ( #21264, #11780, #8078, #5014 ) ) ;
#15404=ORIENTED_EDGE ( 'NONE', *, *, #16255, .F. ) ;
#15405=ORIENTED_EDGE ( 'NONE', *, *, #8801, .F. ) ;
#15406=LINE ( 'NONE', #11416, #7164 ) ;
#15407=EDGE_CURVE ( 'NONE', #8713, #6183, #20626, .T. ) ;
#15409=DIRECTION ( 'NONE',  ( 0.000000000000000000, 0.000000000000000000, -1.000000000000000000 ) ) ;
#15412=CARTESIAN_POINT ( 'NONE',  ( 142.5448000000000093, -3579.494999999999891, 2256.063560000000052 ) ) ;
#15413=LINE ( 'NONE', #4858, #21104 ) ;
#15414=CARTESIAN_POINT ( 'NONE',  ( 20.71779849188069633, -3695.670697890124757, 2259.603314403323111 ) ) ;
#15417=ORIENTED_EDGE ( 'NONE', *, *, #2965, .F. ) ;
#15419=EDGE_CURVE ( 'NONE', #13988, #8337, #13142, .T. ) ;
#15420=AXIS2_PLACEMENT_3D ( 'NONE', #3729, #11002, #1984 ) ;
#15421=CARTESIAN_POINT ( 'NONE',  ( 10.90591201611552918, -3581.702760788150499, 2247.525194624931828 ) ) ;
#15424=DIRECTION ( 'NONE',  ( -1.000000000000000000, 0.000000000000000000, 0.000000000000000000 ) ) ;
#15426=ADVANCED_FACE ( 'NONE', ( #9230 ), #16143, .T. ) ;
#15428=CARTESIAN_POINT ( 'NONE',  ( 144.9794953955964445, -3661.698965784566099, 2245.005495991907537 ) ) ;
#15430=CARTESIAN_POINT ( 'NONE',  ( 10.80273383056147729, -3661.626674884904787, 2249.818717145221399 ) ) ;
#15434=DIRECTION ( 'NONE',  ( -1.000000000000000000, 0.000000000000000000, 0.000000000000000000 ) ) ;
#15435=CIRCLE ( 'NONE', #9063, 3.606799999999993567 ) ;
#15439=CARTESIAN_POINT ( 'NONE',  ( 15.54479951278000094, -3579.494996001999880, 2250.165024905999871 ) ) ;
#15440=EDGE_CURVE ( 'NONE', #14376, #22036, #586, .T. ) ;
#15444=CARTESIAN_POINT ( 'NONE',  ( 9.886192531064313727, -3543.438632178772878, 2255.088321282487868 ) ) ;
#15446=CIRCLE ( 'NONE', #5351, 0.7619999999999294005 ) ;
#15447=DIRECTION ( 'NONE',  ( -1.000000000000000000, 0.000000000000000000, 0.000000000000000000 ) ) ;
#15448=DIRECTION ( 'NONE',  ( 0.000000000000000000, 0.000000000000000000, -1.000000000000000000 ) ) ;
#15451=DIRECTION ( 'NONE',  ( 0.000000000000000000, 0.000000000000000000, 1.000000000000000000 ) ) ;
#15453=AXIS2_PLACEMENT_3D ( 'NONE', #15620, #3417, #19363 ) ;
#15459=ORIENTED_EDGE ( 'NONE', *, *, #799, .T. ) ;
#15461=CARTESIAN_POINT ( 'NONE',  ( 10.79926234752687364, -3657.388342404155082, 2248.114296700302475 ) ) ;
#15462=ORIENTED_EDGE ( 'NONE', *, *, #4197, .F. ) ;
#15464=CARTESIAN_POINT ( 'NONE',  ( 133.9850000019999925, -3579.713624101472305, 2244.668992692525990 ) ) ;
#15465=B_SPLINE_CURVE_WITH_KNOTS ( 'NONE', 3,
 ( #18770, #514, #22395, #21950, #728, #13269, #18658, #11289, #13159, #9645, #2717, #16562, #5916, #11396, #13052, #4143, #18433, #843, #2605, #9866, #15152, #4593, #2390, #7891, #17012, #958, #9528, #18545, #7780, #15041, #2503, #11738, #2836, #14927, #16785, #6026, #15114, #17086, #6443, #20379, #13585 ),
 .UNSPECIFIED., .F., .F.,
 ( 4, 2, 2, 1, 1, 2, 2, 2, 2, 1, 1, 1, 2, 2, 2, 2, 2, 2, 2, 1, 1, 2, 2, 4 ),
 ( 0.000000000000000000, 0.1250000000095896624, 0.1875000000141738565, 0.2187500000162666269, 0.2343750000172133141, 0.2421875000176866854, 0.2500000000181600290, 0.3750000000202952655, 0.4375000000211895501, 0.4687500000216366924, 0.4843750000217365570, 0.4921875000216623386, 0.4960937500214908646, 0.5000000000213193907, 0.5625000000132820421, 0.5937500000092633679, 0.6250000000052446936, 0.6874999999972074560, 0.7187499999930718753, 0.7343749999908720794, 0.7421874999900024417, 0.7460937499899599201, 0.7499999999899172876, 1.000000000000000000 ),
 .UNSPECIFIED. ) ;
#15466=CIRCLE ( 'NONE', #6130, 5.714999999999998082 ) ;
#15467=EDGE_CURVE ( 'NONE', #23086, #20865, #13191, .T. ) ;
#15468=EDGE_LOOP ( 'NONE', ( #9471, #19008, #11926, #594 ) ) ;
#15471=CARTESIAN_POINT ( 'NONE',  ( 10.30698504218744382, -3577.956537814648073, 2250.089589229602097 ) ) ;
#15473=CARTESIAN_POINT ( 'NONE',  ( 25.39999999999999858, -3660.140000000000327, 2250.236800000000130 ) ) ;
#15474=ORIENTED_EDGE ( 'NONE', *, *, #132, .F. ) ;
#15475=CARTESIAN_POINT ( 'NONE',  ( 131.8036441032290895, -3695.561486999931276, 2259.907704032306810 ) ) ;
#15478=CARTESIAN_POINT ( 'NONE',  ( 14.52429522002816675, -3581.677980615632350, 2246.968202618275427 ) ) ;
#15480=CARTESIAN_POINT ( 'NONE',  ( 134.3639308053563752, -3657.457671737659439, 2246.419512734921227 ) ) ;
#15481=EDGE_LOOP ( 'NONE', ( #19142, #22305, #22880, #16866 ) ) ;
#15482=CARTESIAN_POINT ( 'NONE',  ( 104.4447999999999865, -3670.300000000000182, 2239.771999999999935 ) ) ;
#15486=DIRECTION ( 'NONE',  ( -1.000000000000000000, 0.000000000000000000, 0.000000000000000000 ) ) ;
#15488=VERTEX_POINT ( 'NONE', #4407 ) ;
#15490=CARTESIAN_POINT ( 'NONE',  ( 20.52663075323999919, -3544.443975433000105, 2260.595783961000052 ) ) ;
#15497=DIRECTION ( 'NONE',  ( 0.000000000000000000, 0.000000000000000000, -1.000000000000000000 ) ) ;
#15499=CARTESIAN_POINT ( 'NONE',  ( 0.000000000000000000, -3544.570000000000164, 2240.279999999999745 ) ) ;
#15501=DIRECTION ( 'NONE',  ( -1.000000000000000000, 0.000000000000000000, 0.000000000000000000 ) ) ;
#15502=CARTESIAN_POINT ( 'NONE',  ( 141.9552987850744898, -3657.771063528342893, 2248.967151300436399 ) ) ;
#15504=AXIS2_PLACEMENT_3D ( 'NONE', #17284, #19521, #10497 ) ;
#15511=DIRECTION ( 'NONE',  ( 0.000000000000000000, 0.000000000000000000, -1.000000000000000000 ) ) ;
#15512=EDGE_CURVE ( 'NONE', #21090, #6888, #21764, .T. ) ;
#15516=EDGE_CURVE ( 'NONE', #21672, #16839, #3786, .T. ) ;
#15517=DIRECTION ( 'NONE',  ( 0.000000000000000000, -1.000000000000000000, 0.000000000000000000 ) ) ;
#15520=ORIENTED_EDGE ( 'NONE', *, *, #22157, .F. ) ;
#15521=CARTESIAN_POINT ( 'NONE',  ( 136.9568000000001291, -3580.373257047432617, 2255.967039999999997 ) ) ;
#15522=DIRECTION ( 'NONE',  ( 0.000000000000000000, 0.000000000000000000, 1.000000000000000000 ) ) ;
#15524=CIRCLE ( 'NONE', #16692, 0.7619999999999294005 ) ;
#15525=CYLINDRICAL_SURFACE ( 'NONE', #6500, 2.844800000000091700 ) ;
#15527=CARTESIAN_POINT ( 'NONE',  ( 57.14999999999999858, -3568.700000000000273, 2247.392000000000280 ) ) ;
#15530=VECTOR ( 'NONE', #1270, 1000.000000000000000 ) ;
#15532=AXIS2_PLACEMENT_3D ( 'NONE', #16442, #21499, #19741 ) ;
#15533=EDGE_CURVE ( 'NONE', #13997, #5890, #22494, .T. ) ;
#15534=DIRECTION ( 'NONE',  ( 0.000000000000000000, 0.000000000000000000, 1.000000000000000000 ) ) ;
#15535=CARTESIAN_POINT ( 'NONE',  ( 10.38213137239466732, -3581.144250671618011, 2249.087841259171910 ) ) ;
#15540=CIRCLE ( 'NONE', #18899, 1.269999999999882334 ) ;
#15541=CARTESIAN_POINT ( 'NONE',  ( 20.34169023495000062, -3544.202533098000458, 2260.545675974999995 ) ) ;
#15542=CARTESIAN_POINT ( 'NONE',  ( 145.3794022844519702, -3660.142231666386579, 2244.547199809527683 ) ) ;
#15544=DIRECTION ( 'NONE',  ( 0.000000000000000000, 1.000000000000000000, 0.000000000000000000 ) ) ;
#15545=CARTESIAN_POINT ( 'NONE',  ( 11.44214827259342293, -3662.056613363663928, 2249.494299770979069 ) ) ;
#15547=TOROIDAL_SURFACE ( 'NONE', #19250, 3.606799999998999695, 0.7620000000000000107 ) ;
#15571=TOROIDAL_SURFACE ( 'NONE', #15201, 3.606799999999999784, 0.7620000000000000107 ) ;
#15572=DIRECTION ( 'NONE',  ( 1.000000000000000000, 0.000000000000000000, 0.000000000000000000 ) ) ;
#15574=AXIS2_PLACEMENT_3D ( 'NONE', #15243, #22370, #6229 ) ;
#15581=VECTOR ( 'NONE', #16810, 1000.000000000000000 ) ;
#15583=CARTESIAN_POINT ( 'NONE',  ( 147.3230419228115693, -3694.590198012000656, 2260.592443268617444 ) ) ;
#15584=CIRCLE ( 'NONE', #9178, 2.844800000000091700 ) ;
#15588=CARTESIAN_POINT ( 'NONE',  ( 76.20000000000000284, -3670.300000000000182, 2259.837999999999738 ) ) ;
#15589=ORIENTED_EDGE ( 'NONE', *, *, #9526, .T. ) ;
#15592=EDGE_CURVE ( 'NONE', #21188, #14926, #15698, .T. ) ;
#15594=TOROIDAL_SURFACE ( 'NONE', #2129, 4.114799999999999791, 1.270000000000000018 ) ;
#15595=EDGE_CURVE ( 'NONE', #13823, #18734, #437, .T. ) ;
#15596=CARTESIAN_POINT ( 'NONE',  ( 9.652920519510999497, -3695.699999999999818, 2254.503999999999905 ) ) ;
#15598=CARTESIAN_POINT ( 'NONE',  ( 131.7018716228582491, -3695.661851662454410, 2259.652921219497784 ) ) ;
#15600=CARTESIAN_POINT ( 'NONE',  ( 9.956800000000452400, -3578.616742952519417, 2255.967039999999997 ) ) ;
#15603=DIRECTION ( 'NONE',  ( -1.000000000000000000, 0.000000000000000000, 0.000000000000000000 ) ) ;
#15605=DIRECTION ( 'NONE',  ( 0.000000000000000000, 0.000000000000000000, -1.000000000000000000 ) ) ;
#15606=ORIENTED_EDGE ( 'NONE', *, *, #6520, .T. ) ;
#15607=TOROIDAL_SURFACE ( 'NONE', #14103, 3.606799999999999784, 0.7620000000000000107 ) ;
#15608=CARTESIAN_POINT ( 'NONE',  ( 15.56750744765447436, -3695.617810904695034, 2254.953947933142899 ) ) ;
#15612=VERTEX_POINT ( 'NONE', #6400 ) ;
#15613=CARTESIAN_POINT ( 'NONE',  ( 79.80679999999999552, -3568.700000000000273, 2260.600000000000364 ) ) ;
#15614=DIRECTION ( 'NONE',  ( -1.000000000000000000, 0.000000000000000000, 0.000000000000000000 ) ) ;
#15616=ORIENTED_EDGE ( 'NONE', *, *, #20017, .F. ) ;
#15619=AXIS2_PLACEMENT_3D ( 'NONE', #16536, #489, #14211 ) ;
#15620=CARTESIAN_POINT ( 'NONE',  ( 59.89320000000000022, -3644.899999999999636, 2259.837999999999738 ) ) ;
#15623=CARTESIAN_POINT ( 'NONE',  ( 97.99320000000000164, -3568.700000000000273, 2260.600000000000364 ) ) ;
#15626=AXIS2_PLACEMENT_3D ( 'NONE', #12636, #17783, #21315 ) ;
#15628=CARTESIAN_POINT ( 'NONE',  ( 7.020566483207999475, -3660.139755500999854, 2244.547200037999573 ) ) ;
#15629=DIRECTION ( 'NONE',  ( 0.000000000000000000, 0.000000000000000000, -1.000000000000000000 ) ) ;
#15632=CARTESIAN_POINT ( 'NONE',  ( 142.1880353584854220, -3658.125296333661936, 2249.401294179523120 ) ) ;
#15633=ORIENTED_EDGE ( 'NONE', *, *, #15592, .T. ) ;
#15637=AXIS2_PLACEMENT_3D ( 'NONE', #15828, #9996, #19025 ) ;
#15638=CARTESIAN_POINT ( 'NONE',  ( 116.8400000000000034, -3694.430000000000291, 2250.236800000000130 ) ) ;
#15640=ORIENTED_EDGE ( 'NONE', *, *, #1197, .T. ) ;
#15641=CARTESIAN_POINT ( 'NONE',  ( 15.24000000000000021, -3544.570000000000164, 2255.774000000000342 ) ) ;
#15643=CARTESIAN_POINT ( 'NONE',  ( 136.8552000000001669, -3659.956214629431997, 2256.063560000000052 ) ) ;
#15647=LINE ( 'NONE', #15763, #21061 ) ;
#15649=DIRECTION ( 'NONE',  ( -1.000000000000000000, 0.000000000000000000, 0.000000000000000000 ) ) ;
#15652=PRODUCT_DEFINITION ( 'UNKNOWN', '', #10864, #17210 ) ;
#15653=AXIS2_PLACEMENT_3D ( 'NONE', #8456, #22612, #3397 ) ;
#15656=CARTESIAN_POINT ( 'NONE',  ( 63.50000000000000000, -3594.099999999999909, 2239.009999999999764 ) ) ;
#15658=DIRECTION ( 'NONE',  ( -1.000000000000000000, 0.000000000000000000, 0.000000000000000000 ) ) ;
#15659=EDGE_LOOP ( 'NONE', ( #2600, #11804 ) ) ;
#15661=FACE_BOUND ( 'NONE', #5603, .T. ) ;
#15664=CARTESIAN_POINT ( 'NONE',  ( 144.7333290304783304, -3662.211819972148987, 2245.442509231050281 ) ) ;
#15666=DIRECTION ( 'NONE',  ( 0.000000000000000000, 0.000000000000000000, 1.000000000000000000 ) ) ;
#15668=CARTESIAN_POINT ( 'NONE',  ( 147.5076778864620621, -3543.579977980994954, 2260.129759352632391 ) ) ;
#15671=VECTOR ( 'NONE', #13912, 1000.000000000000000 ) ;
#15673=FACE_OUTER_BOUND ( 'NONE', #14187, .T. ) ;
#15677=DIRECTION ( 'NONE',  ( 0.000000000000000000, 0.000000000000000000, -1.000000000000000000 ) ) ;
#15678=ORIENTED_EDGE ( 'NONE', *, *, #6216, .T. ) ;
#15688=CARTESIAN_POINT ( 'NONE',  ( 88.90000000000000568, -3644.899999999999636, 2259.837999999999738 ) ) ;
#15689=ADVANCED_FACE ( 'NONE', ( #22781 ), #6871, .F. ) ;
#15692=ORIENTED_EDGE ( 'NONE', *, *, #8354, .T. ) ;
#15693=CARTESIAN_POINT ( 'NONE',  ( 147.8270794805000037, -3695.699999999999818, 2259.329999999999927 ) ) ;
#15697=CARTESIAN_POINT ( 'NONE',  ( 10.46449438243440433, -3657.744798957563944, 2248.928716950800663 ) ) ;
#15698=B_SPLINE_CURVE_WITH_KNOTS ( 'NONE', 3,
 ( #12973, #6174, #4295, #4175, #873, #9564, #8039, #9457, #16596, #16710, #664, #7691, #13423, #11650, #18807, #17045, #8160, #21874, #5840, #21984, #547 ),
 .UNSPECIFIED., .F., .F.,
 ( 4, 2, 2, 1, 2, 2, 2, 2, 2, 2, 4 ),
 ( 0.000000000000000000, 0.1249999999978197440, 0.1874999999967315034, 0.2187499999964521435, 0.2343749999963124497, 0.2499999999961727837, 0.3749999999969789721, 0.4999999999977851051, 0.7499999999988021804, 0.8749999999994011457, 1.000000000000000000 ),
 .UNSPECIFIED. ) ;
#15701=DIRECTION ( 'NONE',  ( 1.000000000000000000, 0.000000000000000000, 0.000000000000000000 ) ) ;
#15702=ADVANCED_FACE ( 'NONE', ( #5110 ), #9032, .T. ) ;
#15704=DIRECTION ( 'NONE',  ( 0.000000000000000000, -1.000000000000000000, 0.000000000000000000 ) ) ;
#15707=VERTEX_POINT ( 'NONE', #3333 ) ;
#15710=DIRECTION ( 'NONE',  ( -1.224646799147353207E-16, 1.000000000000000000, 0.000000000000000000 ) ) ;
#15711=CARTESIAN_POINT ( 'NONE',  ( 14.52753400248703741, -3581.675156902885647, 2247.803913149289656 ) ) ;
#15712=TOROIDAL_SURFACE ( 'NONE', #16459, 3.606799999999999784, 0.7620000000000000107 ) ;
#15714=CARTESIAN_POINT ( 'NONE',  ( 76.20000000000000284, -3568.700000000000273, 2239.771999999999935 ) ) ;
#15716=CARTESIAN_POINT ( 'NONE',  ( 88.90000000000000568, -3594.099999999999909, 2239.771999999999935 ) ) ;
#15717=ORIENTED_EDGE ( 'NONE', *, *, #23035, .T. ) ;
#15718=DIRECTION ( 'NONE',  ( 1.000000000000000000, 0.000000000000000000, 0.000000000000000000 ) ) ;
#15719=EDGE_CURVE ( 'NONE', #1882, #8573, #3104, .T. ) ;
#15721=FACE_OUTER_BOUND ( 'NONE', #7081, .T. ) ;
#15722=ORIENTED_EDGE ( 'NONE', *, *, #7445, .F. ) ;
#15725=ORIENTED_EDGE ( 'NONE', *, *, #3073, .F. ) ;
#15726=ORIENTED_EDGE ( 'NONE', *, *, #3765, .T. ) ;
#15728=DIRECTION ( 'NONE',  ( -1.073225997510925892E-13, 0.000000000000000000, -1.000000000000000000 ) ) ;
#15729=EDGE_CURVE ( 'NONE', #7197, #18734, #17260, .T. ) ;
#15731=CARTESIAN_POINT ( 'NONE',  ( 0.000000000000000000, -3695.699999999999818, 2239.009999999999764 ) ) ;
#15732=CARTESIAN_POINT ( 'NONE',  ( 15.54478274857000031, -3659.509919104000346, 2250.166342301999521 ) ) ;
#15733=LINE ( 'NONE', #17593, #15837 ) ;
#15740=CARTESIAN_POINT ( 'NONE',  ( 76.20000000000000284, -3568.700000000000273, 2259.837999999999738 ) ) ;
#15741=DIRECTION ( 'NONE',  ( 0.000000000000000000, 0.000000000000000000, 1.000000000000000000 ) ) ;
#15744=CARTESIAN_POINT ( 'NONE',  ( 141.8623322999648337, -3657.656292019905322, 2248.779374755923982 ) ) ;
#15745=ORIENTED_EDGE ( 'NONE', *, *, #8824, .F. ) ;
#15747=EDGE_CURVE ( 'NONE', #16647, #825, #10024, .T. ) ;
#15748=VERTEX_POINT ( 'NONE', #8269 ) ;
#15749=ORIENTED_EDGE ( 'NONE', *, *, #5959, .F. ) ;
#15752=ORIENTED_EDGE ( 'NONE', *, *, #5992, .F. ) ;
#15754=CARTESIAN_POINT ( 'NONE',  ( 145.3795747169000094, -3578.859731361000286, 2244.547525601999951 ) ) ;
#15755=ORIENTED_EDGE ( 'NONE', *, *, #22160, .T. ) ;
#15756=ORIENTED_EDGE ( 'NONE', *, *, #18733, .F. ) ;
#15758=DIRECTION ( 'NONE',  ( 0.000000000000000000, 0.000000000000000000, -1.000000000000000000 ) ) ;
#15760=EDGE_LOOP ( 'NONE', ( #17061, #19326, #4845, #3314 ) ) ;
#15761=CARTESIAN_POINT ( 'NONE',  ( 50.79999999999999716, -3619.500000000000000, 2259.837999999999738 ) ) ;
#15762=DIRECTION ( 'NONE',  ( 0.000000000000000000, 0.000000000000000000, -1.000000000000000000 ) ) ;
#15763=CARTESIAN_POINT ( 'NONE',  ( 25.39999999999999858, -3660.140000000000327, 2244.547199999999975 ) ) ;
#15770=CARTESIAN_POINT ( 'NONE',  ( 10.45683289038945674, -3581.244648887170115, 2248.943261231277575 ) ) ;
#15774=VERTEX_POINT ( 'NONE', #5460 ) ;
#15775=PLANE ( 'NONE',  #3602 ) ;
#15778=CARTESIAN_POINT ( 'NONE',  ( 145.1382046083306534, -3577.698739476651099, 2244.777305218250604 ) ) ;
#15779=DIRECTION ( 'NONE',  ( -1.000000000000000000, 0.000000000000000000, 0.000000000000000000 ) ) ;
#15780=CARTESIAN_POINT ( 'NONE',  ( 10.57261563002993832, -3661.393710553322762, 2249.945659169295141 ) ) ;
#15782=CARTESIAN_POINT ( 'NONE',  ( 147.3681911278365533, -3544.023782195929925, 2260.479223148535311 ) ) ;
#15785=CARTESIAN_POINT ( 'NONE',  ( 76.20000000000000284, -3568.700000000000273, 2239.771999999999935 ) ) ;
#15787=CARTESIAN_POINT ( 'NONE',  ( 95.25000000000000000, -3694.430000000000291, 2247.392000000000280 ) ) ;
#15789=AXIS2_PLACEMENT_3D ( 'NONE', #734, #22065, #20429 ) ;
#15791=VECTOR ( 'NONE', #4679, 1000.000000000000000 ) ;
#15793=B_SPLINE_CURVE_WITH_KNOTS ( 'NONE', 3,
 ( #16441, #2037, #21723, #5677 ),
 .UNSPECIFIED., .F., .F.,
 ( 4, 4 ),
 ( 0.000000000000000000, 1.000000000000000000 ),
 .UNSPECIFIED. ) ;
#15794=VERTEX_POINT ( 'NONE', #14484 ) ;
#15795=CARTESIAN_POINT ( 'NONE',  ( 9.698254030477786003, -3543.300000000000182, 2254.617539516272700 ) ) ;
#15797=CYLINDRICAL_SURFACE ( 'NONE', #21354, 5.715000000000997282 ) ;
#15798=LINE ( 'NONE', #8420, #9573 ) ;
#15799=FACE_OUTER_BOUND ( 'NONE', #11751, .T. ) ;
#15801=AXIS2_PLACEMENT_3D ( 'NONE', #16310, #18408, #267 ) ;
#15802=DIRECTION ( 'NONE',  ( 0.000000000000000000, 0.000000000000000000, 1.000000000000000000 ) ) ;
#15809=FACE_OUTER_BOUND ( 'NONE', #14760, .T. ) ;
#15810=ADVANCED_FACE ( 'NONE', ( #9202 ), #16115, .F. ) ;
#15813=ADVANCED_FACE ( 'NONE', ( #7330 ), #12363, .T. ) ;
#15815=EDGE_LOOP ( 'NONE', ( #7209, #6633 ) ) ;
#15816=VERTEX_POINT ( 'NONE', #9084 ) ;
#15817=EDGE_CURVE ( 'NONE', #14376, #4689, #11285, .T. ) ;
#15822=CARTESIAN_POINT ( 'NONE',  ( 131.8608747668832564, -3695.477144326939651, 2260.051190193429193 ) ) ;
#15824=AXIS2_PLACEMENT_3D ( 'NONE', #5068, #10334, #7067 ) ;
#15825=CARTESIAN_POINT ( 'NONE',  ( 136.6529205195000145, -3695.699999999999818, 2254.503999999999905 ) ) ;
#15826=EDGE_CURVE ( 'NONE', #3143, #7313, #14909, .T. ) ;
#15827=CARTESIAN_POINT ( 'NONE',  ( 15.27563337016521317, -3580.706179722078105, 2249.559177238421853 ) ) ;
#15828=CARTESIAN_POINT ( 'NONE',  ( 12.69999999999999929, -3659.504999999999654, 2272.030000000000200 ) ) ;
#15831=CARTESIAN_POINT ( 'NONE',  ( 116.8400000000000034, -3544.570000000000164, 2247.392000000000280 ) ) ;
#15832=VERTEX_POINT ( 'NONE', #177 ) ;
#15833=AXIS2_PLACEMENT_3D ( 'NONE', #6098, #19926, #8426 ) ;
#15834=CARTESIAN_POINT ( 'NONE',  ( 151.1299999999999955, -3544.570000000000164, 2259.329999999999927 ) ) ;
#15835=FACE_OUTER_BOUND ( 'NONE', #3020, .T. ) ;
#15836=ORIENTED_EDGE ( 'NONE', *, *, #5931, .T. ) ;
#15837=VECTOR ( 'NONE', #4716, 1000.000000000000000 ) ;
#15839=DIRECTION ( 'NONE',  ( 0.000000000000000000, 0.000000000000000000, -1.000000000000000000 ) ) ;
#15841=ORIENTED_EDGE ( 'NONE', *, *, #13275, .F. ) ;
#15844=DIRECTION ( 'NONE',  ( -1.000000000000000000, 0.000000000000000000, 0.000000000000000000 ) ) ;
#15849=CARTESIAN_POINT ( 'NONE',  ( 136.8603346907000002, -3579.284436177999851, 2250.207695148999846 ) ) ;
#15850=AXIS2_PLACEMENT_3D ( 'NONE', #14310, #14076, #20990 ) ;
#15853=ADVANCED_FACE ( 'NONE', ( #6991 ), #21390, .T. ) ;
#15854=CARTESIAN_POINT ( 'NONE',  ( 28.24479999999899604, -3670.300000000000182, 2259.837999999999738 ) ) ;
#15855=CARTESIAN_POINT ( 'NONE',  ( 9.989282597016131859, -3695.380630527866288, 2255.346357850532968 ) ) ;
#15857=AXIS2_PLACEMENT_3D ( 'NONE', #569, #22009, #13108 ) ;
#15859=DIRECTION ( 'NONE',  ( -1.000000000000000000, 0.000000000000000000, 0.000000000000000000 ) ) ;
#15869=ORIENTED_EDGE ( 'NONE', *, *, #16255, .T. ) ;
#15870=FACE_OUTER_BOUND ( 'NONE', #12345, .T. ) ;
#15874=VERTEX_POINT ( 'NONE', #20322 ) ;
#15875=CARTESIAN_POINT ( 'NONE',  ( 137.1599999999999966, -3580.776127254000130, 2255.774000000000342 ) ) ;
#15876=CARTESIAN_POINT ( 'NONE',  ( 57.14999999999999858, -3694.430000000000291, 2247.392000000000280 ) ) ;
#15878=CARTESIAN_POINT ( 'NONE',  ( 127.0000000000000000, -3660.140000000000327, 2247.392000000000280 ) ) ;
#15879=VERTEX_POINT ( 'NONE', #4150 ) ;
#15881=ADVANCED_FACE ( 'NONE', ( #13058 ), #18665, .F. ) ;
#15883=VERTEX_POINT ( 'NONE', #14823 ) ;
#15885=EDGE_CURVE ( 'NONE', #13759, #20359, #4549, .T. ) ;
#15887=CARTESIAN_POINT ( 'NONE',  ( 10.27313954880075109, -3580.979417148001176, 2249.290044219352239 ) ) ;
#15889=FACE_OUTER_BOUND ( 'NONE', #18648, .T. ) ;
#15892=VERTEX_POINT ( 'NONE', #13276 ) ;
#15893=DIRECTION ( 'NONE',  ( 0.000000000000000000, 0.000000000000000000, 1.000000000000000000 ) ) ;
#15895=PLANE ( 'NONE',  #2853 ) ;
#15897=CARTESIAN_POINT ( 'NONE',  ( 11.22865419974734102, -3661.939788859982855, 2249.595128560251851 ) ) ;
#15898=EDGE_CURVE ( 'NONE', #3611, #21098, #19145, .T. ) ;
#15902=AXIS2_PLACEMENT_3D ( 'NONE', #12200, #21456, #10439 ) ;
#15903=DIRECTION ( 'NONE',  ( 0.000000000000000000, 0.000000000000000000, -1.000000000000000000 ) ) ;
#15904=AXIS2_PLACEMENT_3D ( 'NONE', #7058, #4842, #13638 ) ;
#15907=CARTESIAN_POINT ( 'NONE',  ( 14.94580037973010889, -3657.758775493699432, 2248.948511419066108 ) ) ;
#15911=ORIENTED_EDGE ( 'NONE', *, *, #19227, .T. ) ;
#15915=DIRECTION ( 'NONE',  ( 0.000000000000000000, 0.000000000000000000, -1.000000000000000000 ) ) ;
#15917=LINE ( 'NONE', #3485, #14080 ) ;
#15919=CIRCLE ( 'NONE', #21525, 0.7619999999999987894 ) ;
#15920=LINE ( 'NONE', #14169, #18607 ) ;
#15921=VECTOR ( 'NONE', #10061, 1000.000000000000000 ) ;
#15925=EDGE_LOOP ( 'NONE', ( #380, #12782, #1374, #15356, #1618, #6280, #18086, #9413 ) ) ;
#15928=VERTEX_POINT ( 'NONE', #18441 ) ;
#15929=DIRECTION ( 'NONE',  ( 1.000000000000000000, 0.000000000000000000, 0.000000000000000000 ) ) ;
#15930=ORIENTED_EDGE ( 'NONE', *, *, #5407, .T. ) ;
#15931=CARTESIAN_POINT ( 'NONE',  ( 127.0000000000000000, -3578.860000000000127, 2244.547199999999975 ) ) ;
#15932=AXIS2_PLACEMENT_3D ( 'NONE', #6890, #3354, #12382 ) ;
#15942=CARTESIAN_POINT ( 'NONE',  ( 15.35573774336631914, -3580.514832482311249, 2249.705997884422686 ) ) ;
#15943=DIRECTION ( 'NONE',  ( 0.000000000000000000, 1.000000000000000000, 0.000000000000000000 ) ) ;
#15944=CARTESIAN_POINT ( 'NONE',  ( 9.916854418464000176, -3578.905956564000007, 2250.236428761999832 ) ) ;
#15946=ADVANCED_FACE ( 'NONE', ( #20532 ), #18555, .F. ) ;
#15950=CARTESIAN_POINT ( 'NONE',  ( 15.41076828073257055, -3695.380630529619793, 2255.346378162581459 ) ) ;
#15952=VECTOR ( 'NONE', #18018, 1000.000000000000000 ) ;
#15954=ORIENTED_EDGE ( 'NONE', *, *, #2265, .T. ) ;
#15957=CIRCLE ( 'NONE', #2525, 2.844799999999961582 ) ;
#15958=ORIENTED_EDGE ( 'NONE', *, *, #10451, .T. ) ;
#15960=TOROIDAL_SURFACE ( 'NONE', #14848, 3.606799999999999784, 0.7620000000000000107 ) ;
#15965=DIRECTION ( 'NONE',  ( 0.000000000000000000, 1.000000000000000000, 0.000000000000000000 ) ) ;
#15967=AXIS2_PLACEMENT_3D ( 'NONE', #4032, #19622, #11057 ) ;
#15969=CARTESIAN_POINT ( 'NONE',  ( 117.9067999999989951, -3594.099999999999909, 2239.009999999999764 ) ) ;
#15970=TOROIDAL_SURFACE ( 'NONE', #12614, 3.606799999999999784, 0.7620000000000000107 ) ;
#15972=CARTESIAN_POINT ( 'NONE',  ( 137.9080942012932951, -3657.295453499272298, 2247.303175097353687 ) ) ;
#15974=ADVANCED_FACE ( 'NONE', ( #5807 ), #18030, .T. ) ;
#15977=CARTESIAN_POINT ( 'NONE',  ( 137.1196777603386181, -3660.705328851377089, 2250.180928057881374 ) ) ;
#15979=ORIENTED_EDGE ( 'NONE', *, *, #19451, .T. ) ;
#15985=ORIENTED_EDGE ( 'NONE', *, *, #5665, .F. ) ;
#15987=CARTESIAN_POINT ( 'NONE',  ( 151.4000000000000057, -3695.699999999999818, 2239.039032635400417 ) ) ;
#15989=CARTESIAN_POINT ( 'NONE',  ( 101.5999999999999943, -3619.500000000000000, 2261.869999999999891 ) ) ;
#15990=CARTESIAN_POINT ( 'NONE',  ( 127.0000000000000000, -3619.500000000000000, 2239.009999999999764 ) ) ;
#15992=CARTESIAN_POINT ( 'NONE',  ( 97.99320000000000164, -3619.500000000000000, 2260.600000000000364 ) ) ;
#15993=CARTESIAN_POINT ( 'NONE',  ( 57.14999999999999858, -3568.700000000000273, 2247.392000000000280 ) ) ;
#15996=CARTESIAN_POINT ( 'NONE',  ( 114.2999999999999972, -3594.099999999999909, 2239.771999999999935 ) ) ;
#15997=VERTEX_POINT ( 'NONE', #10224 ) ;
#16000=CARTESIAN_POINT ( 'NONE',  ( 131.7408816625886345, -3543.371700234166838, 2259.750712803343049 ) ) ;
#16001=DIRECTION ( 'NONE',  ( 1.000000000000000000, 0.000000000000000000, 0.000000000000000000 ) ) ;
#16002=CIRCLE ( 'NONE', #22713, 4.114799999999974034 ) ;
#16003=DIRECTION ( 'NONE',  ( 0.000000000000000000, 0.000000000000000000, -1.000000000000000000 ) ) ;
#16008=CARTESIAN_POINT ( 'NONE',  ( 144.5184724295484671, -3576.421590092805673, 2245.925647645899062 ) ) ;
#16009=FACE_OUTER_BOUND ( 'NONE', #3594, .T. ) ;
#16011=EDGE_CURVE ( 'NONE', #6769, #16761, #14673, .T. ) ;
#16012=EDGE_CURVE ( 'NONE', #21114, #11744, #7555, .T. ) ;
#16013=FACE_OUTER_BOUND ( 'NONE', #4583, .T. ) ;
#16014=ORIENTED_EDGE ( 'NONE', *, *, #22429, .T. ) ;
#16015=EDGE_CURVE ( 'NONE', #20116, #6254, #449, .T. ) ;
#16019=DIRECTION ( 'NONE',  ( 0.000000000000000000, -1.000000000000000000, 0.000000000000000000 ) ) ;
#16020=CARTESIAN_POINT ( 'NONE',  ( 15.35765731516040056, -3658.489959486714270, 2249.709633093460980 ) ) ;
#16021=CARTESIAN_POINT ( 'NONE',  ( 136.8825577675800105, -3695.562642952237638, 2255.079235783421609 ) ) ;
#16024=CARTESIAN_POINT ( 'NONE',  ( 1.270000000000000018, -3578.860000000000127, 2243.277199999999993 ) ) ;
#16026=VECTOR ( 'NONE', #10551, 1000.000000000000000 ) ;
#16028=CARTESIAN_POINT ( 'NONE',  ( 10.01184914621919653, -3543.672816122378208, 2255.402917874179821 ) ) ;
#16030=EDGE_CURVE ( 'NONE', #18590, #22471, #2722, .T. ) ;
#16033=DIRECTION ( 'NONE',  ( 0.000000000000000000, 0.000000000000000000, -1.000000000000000000 ) ) ;
#16034=CARTESIAN_POINT ( 'NONE',  ( 14.61266695128000137, -3657.399152860999493, 2246.630000000000109 ) ) ;
#16035=LINE ( 'NONE', #17904, #11475 ) ;
#16036=AXIS2_PLACEMENT_3D ( 'NONE', #1436, #19486, #21364 ) ;
#16037=ORIENTED_EDGE ( 'NONE', *, *, #22015, .F. ) ;
#16038=DIRECTION ( 'NONE',  ( -1.073225997510925892E-13, 0.000000000000000000, -1.000000000000000000 ) ) ;
#16041=ADVANCED_FACE ( 'NONE', ( #22866 ), #15276, .F. ) ;
#16045=EDGE_LOOP ( 'NONE', ( #21093, #4981 ) ) ;
#16046=DIRECTION ( 'NONE',  ( 0.000000000000000000, 0.000000000000000000, 1.000000000000000000 ) ) ;
#16047=CYLINDRICAL_SURFACE ( 'NONE', #7558, 2.844799999999999773 ) ;
#16048=VERTEX_POINT ( 'NONE', #6842 ) ;
#16049=ORIENTED_EDGE ( 'NONE', *, *, #17820, .F. ) ;
#16050=CARTESIAN_POINT ( 'NONE',  ( 137.0385493787570965, -3580.499829900386885, 2249.716652619521483 ) ) ;
#16051=ORIENTED_EDGE ( 'NONE', *, *, #2078, .F. ) ;
#16052=VECTOR ( 'NONE', #12876, 1000.000000000000000 ) ;
#16053=CARTESIAN_POINT ( 'NONE',  ( 60.65520000000000067, -3644.899999999999636, 2259.837999999999738 ) ) ;
#16055=DIRECTION ( 'NONE',  ( -0.000000000000000000, -1.000000000000000000, -0.000000000000000000 ) ) ;
#16056=DIRECTION ( 'NONE',  ( 0.000000000000000000, 0.000000000000000000, -1.000000000000000000 ) ) ;
#16058=DIRECTION ( 'NONE',  ( 1.000000000000000000, 0.000000000000000000, 0.000000000000000000 ) ) ;
#16060=ORIENTED_EDGE ( 'NONE', *, *, #3478, .F. ) ;
#16063=VERTEX_POINT ( 'NONE', #13755 ) ;
#16064=CARTESIAN_POINT ( 'NONE',  ( 4.934178814895267884, -3695.321318630448332, 2260.234746714515040 ) ) ;
#16065=AXIS2_PLACEMENT_3D ( 'NONE', #8875, #16019, #7116 ) ;
#16066=DIRECTION ( 'NONE',  ( 0.000000000000000000, 0.000000000000000000, -1.000000000000000000 ) ) ;
#16068=CARTESIAN_POINT ( 'NONE',  ( 20.34169023495000062, -3544.202533098000458, 2260.545675974999995 ) ) ;
#16072=ORIENTED_EDGE ( 'NONE', *, *, #14607, .T. ) ;
#16074=CYLINDRICAL_SURFACE ( 'NONE', #20589, 1.269999999999900320 ) ;
#16080=ORIENTED_EDGE ( 'NONE', *, *, #12108, .F. ) ;
#16083=CARTESIAN_POINT ( 'NONE',  ( 35.56000000000000227, -3695.699999999999818, 2247.392000000000280 ) ) ;
#16088=CARTESIAN_POINT ( 'NONE',  ( 137.0620653827227500, -3658.440016311159980, 2249.673027215405909 ) ) ;
#16089=ORIENTED_EDGE ( 'NONE', *, *, #12746, .T. ) ;
#16091=VERTEX_POINT ( 'NONE', #5075 ) ;
#16096=AXIS2_PLACEMENT_3D ( 'NONE', #6675, #15448, #4785 ) ;
#16099=EDGE_LOOP ( 'NONE', ( #13998, #5558, #11189, #1391 ) ) ;
#16100=EDGE_LOOP ( 'NONE', ( #9406, #19855, #15269, #7674 ) ) ;
#16104=DIRECTION ( 'NONE',  ( -0.9296367896487196525, 0.3684771897032736443, 0.000000000000000000 ) ) ;
#16108=ADVANCED_FACE ( 'NONE', ( #1435 ), #13916, .T. ) ;
#16109=FACE_BOUND ( 'NONE', #3065, .T. ) ;
#16110=CARTESIAN_POINT ( 'NONE',  ( 6.985000002048998624, -3579.713624101183086, 2244.668992692460506 ) ) ;
#16115=CYLINDRICAL_SURFACE ( 'NONE', #21009, 2.844799999999994444 ) ;
#16117=CARTESIAN_POINT ( 'NONE',  ( 25.39999999999999858, -3578.860000000000127, 2247.392000000000280 ) ) ;
#16124=CARTESIAN_POINT ( 'NONE',  ( 47.95519999999999783, -3619.500000000000000, 2239.771999999999935 ) ) ;
#16127=CARTESIAN_POINT ( 'NONE',  ( 18.25163997286968254, -3658.148427273620200, 2245.360569998716983 ) ) ;
#16130=B_SPLINE_CURVE_WITH_KNOTS ( 'NONE', 3,
 ( #3921, #7446, #3803, #183, #16231, #16348, #5584, #18330, #10957, #16571, #2398, #4042, #12944, #18102, #5813, #4152, #20103, #11188, #16455 ),
 .UNSPECIFIED., .F., .F.,
 ( 4, 2, 2, 1, 2, 2, 2, 2, 2, 4 ),
 ( 0.000000000000000000, 0.1249999999982433219, 0.1874999999975868747, 0.2187499999972586651, 0.2343749999970945463, 0.2499999999969304554, 0.3749999999975224818, 0.4999999999981145082, 0.7499999999990571986, 1.000000000000000000 ),
 .UNSPECIFIED. ) ;
#16134=CARTESIAN_POINT ( 'NONE',  ( 0.000000000000000000, -3578.860000000000127, 2251.506800000000112 ) ) ;
#16139=ORIENTED_EDGE ( 'NONE', *, *, #6085, .T. ) ;
#16141=DIRECTION ( 'NONE',  ( -1.000000000000000000, 0.000000000000000000, 0.000000000000000000 ) ) ;
#16142=DIRECTION ( 'NONE',  ( -1.000000000000000000, 0.000000000000000000, 0.000000000000000000 ) ) ;
#16143=TOROIDAL_SURFACE ( 'NONE', #10159, 4.114799999999999791, 1.270000000000000018 ) ;
#16145=ADVANCED_FACE ( 'NONE', ( #10458 ), #9046, .T. ) ;
#16146=CIRCLE ( 'NONE', #4520, 0.7619999999999987894 ) ;
#16147=DIRECTION ( 'NONE',  ( -1.000000000000000000, 0.000000000000000000, 0.000000000000000000 ) ) ;
#16148=EDGE_CURVE ( 'NONE', #17874, #22306, #3725, .T. ) ;
#16153=CARTESIAN_POINT ( 'NONE',  ( 25.39999999999999858, -3568.700000000000273, 2239.009999999999764 ) ) ;
#16154=ORIENTED_EDGE ( 'NONE', *, *, #2411, .F. ) ;
#16155=PLANE ( 'NONE',  #13693 ) ;
#16156=FACE_OUTER_BOUND ( 'NONE', #9018, .T. ) ;
#16157=ORIENTED_EDGE ( 'NONE', *, *, #5073, .F. ) ;
#16159=AXIS2_PLACEMENT_3D ( 'NONE', #1312, #13863, #15741 ) ;
#16161=VECTOR ( 'NONE', #6714, 1000.000000000000000 ) ;
#16166=CARTESIAN_POINT ( 'NONE',  ( 137.9071795004996943, -3581.703785729057017, 2247.306121288057057 ) ) ;
#16167=VERTEX_POINT ( 'NONE', #3657 ) ;
#16169=EDGE_CURVE ( 'NONE', #15892, #6818, #797, .T. ) ;
#16170=CARTESIAN_POINT ( 'NONE',  ( 142.2400000000000091, -3544.570000000000164, 2254.503999999999905 ) ) ;
#16171=DIRECTION ( 'NONE',  ( 1.000000000000000000, 0.000000000000000000, 0.000000000000000000 ) ) ;
#16172=B_SPLINE_CURVE_WITH_KNOTS ( 'NONE', 3,
 ( #6700, #6351, #15600, #2816 ),
 .UNSPECIFIED., .F., .F.,
 ( 4, 4 ),
 ( 0.000000000000000000, 1.000000000000000000 ),
 .UNSPECIFIED. ) ;
#16173=CIRCLE ( 'NONE', #6076, 2.844799999999009010 ) ;
#16175=CARTESIAN_POINT ( 'NONE',  ( 101.5999999999999943, -3619.500000000000000, 2259.837999999999738 ) ) ;
#16176=AXIS2_PLACEMENT_3D ( 'NONE', #18144, #19678, #112 ) ;
#16177=CARTESIAN_POINT ( 'NONE',  ( 142.1753987576898055, -3578.092974057908123, 2250.131498804146304 ) ) ;
#16178=ORIENTED_EDGE ( 'NONE', *, *, #5208, .T. ) ;
#16179=CARTESIAN_POINT ( 'NONE',  ( 134.2649038272905386, -3577.728047718949256, 2244.781081195526895 ) ) ;
#16182=ORIENTED_EDGE ( 'NONE', *, *, #4797, .F. ) ;
#16186=ADVANCED_FACE ( 'NONE', ( #23102 ), #7416, .T. ) ;
#16187=VERTEX_POINT ( 'NONE', #14566 ) ;
#16191=TOROIDAL_SURFACE ( 'NONE', #4944, 3.606799999999999784, 0.7620000000000000107 ) ;
#16193=AXIS2_PLACEMENT_3D ( 'NONE', #11229, #2329, #18488 ) ;
#16196=LINE ( 'NONE', #147, #21792 ) ;
#16200=DIRECTION ( 'NONE',  ( 0.000000000000000000, 1.000000000000000000, 0.000000000000000000 ) ) ;
#16201=VERTEX_POINT ( 'NONE', #21706 ) ;
#16204=CARTESIAN_POINT ( 'NONE',  ( 22.55520000000100111, -3568.700000000000273, 2259.837999999999738 ) ) ;
#16205=ORIENTED_EDGE ( 'NONE', *, *, #17026, .F. ) ;
#16207=CARTESIAN_POINT ( 'NONE',  ( 137.6831814252260813, -3661.513472532589276, 2249.884315932574737 ) ) ;
#16209=ORIENTED_EDGE ( 'NONE', *, *, #18822, .T. ) ;
#16210=ORIENTED_EDGE ( 'NONE', *, *, #11519, .T. ) ;
#16212=VERTEX_POINT ( 'NONE', #10692 ) ;
#16214=FACE_OUTER_BOUND ( 'NONE', #1157, .T. ) ;
#16217=CIRCLE ( 'NONE', #12837, 2.844799999999994444 ) ;
#16221=CARTESIAN_POINT ( 'NONE',  ( 57.14999999999999858, -3543.299999999999727, 2247.392000000000280 ) ) ;
#16222=CARTESIAN_POINT ( 'NONE',  ( 7.086979097592000620, -3580.606330658807565, 2245.129232553048496 ) ) ;
#16227=CARTESIAN_POINT ( 'NONE',  ( 131.9328299862054905, -3543.675011529194762, 2260.231706197272615 ) ) ;
#16231=CARTESIAN_POINT ( 'NONE',  ( 7.939941740107332002, -3662.668415385413937, 2246.085609779290280 ) ) ;
#16232=ORIENTED_EDGE ( 'NONE', *, *, #17520, .F. ) ;
#16233=VECTOR ( 'NONE', #3488, 1000.000000000000000 ) ;
#16236=EDGE_CURVE ( 'NONE', #12668, #6472, #6830, .T. ) ;
#16241=CARTESIAN_POINT ( 'NONE',  ( 18.11755229430770697, -3657.685221718821140, 2245.954260265993980 ) ) ;
#16247=EDGE_CURVE ( 'NONE', #14745, #4174, #22526, .T. ) ;
#16248=CARTESIAN_POINT ( 'NONE',  ( 136.9313810085959062, -3695.492037868740226, 2255.201647171010791 ) ) ;
#16249=ORIENTED_EDGE ( 'NONE', *, *, #20451, .F. ) ;
#16252=CIRCLE ( 'NONE', #1268, 2.844800000000001550 ) ;
#16254=ORIENTED_EDGE ( 'NONE', *, *, #5511, .T. ) ;
#16255=EDGE_CURVE ( 'NONE', #17585, #6642, #12945, .T. ) ;
#16258=CYLINDRICAL_SURFACE ( 'NONE', #17288, 1.269999999999882334 ) ;
#16259=DIRECTION ( 'NONE',  ( -1.224646799147353207E-16, 1.000000000000000000, 0.000000000000000000 ) ) ;
#16260=DIRECTION ( 'NONE',  ( 1.000000000000000000, -0.000000000000000000, 1.224646799147353207E-16 ) ) ;
#16261=CARTESIAN_POINT ( 'NONE',  ( 101.5999999999999943, -3568.700000000000273, 2261.869999999999891 ) ) ;
#16265=ORIENTED_EDGE ( 'NONE', *, *, #11943, .T. ) ;
#16267=EDGE_CURVE ( 'NONE', #16307, #1882, #2254, .T. ) ;
#16270=ADVANCED_FACE ( 'NONE', ( #18415 ), #16191, .T. ) ;
#16274=CARTESIAN_POINT ( 'NONE',  ( 25.39999999999999858, -3660.140000000000327, 2247.392000000000280 ) ) ;
#16276=CARTESIAN_POINT ( 'NONE',  ( 142.2429993025672275, -3694.590198013145255, 2255.766426251082976 ) ) ;
#16279=CARTESIAN_POINT ( 'NONE',  ( 137.8421157351343709, -3581.650442338845551, 2246.808394885380039 ) ) ;
#16281=VERTEX_POINT ( 'NONE', #5660 ) ;
#16284=AXIS2_PLACEMENT_3D ( 'NONE', #8780, #3612, #15929 ) ;
#16285=AXIS2_PLACEMENT_3D ( 'NONE', #20764, #3300, #15844 ) ;
#16286=DIRECTION ( 'NONE',  ( 0.000000000000000000, 1.000000000000000000, 0.000000000000000000 ) ) ;
#16289=CARTESIAN_POINT ( 'NONE',  ( 105.2067999999999870, -3670.300000000000182, 2259.837999999999738 ) ) ;
#16290=CARTESIAN_POINT ( 'NONE',  ( 138.0864475737284067, -3577.151256281058068, 2249.666874368690515 ) ) ;
#16291=EDGE_LOOP ( 'NONE', ( #16080, #4224, #11411, #19799 ) ) ;
#16292=CARTESIAN_POINT ( 'NONE',  ( 134.0205977155505650, -3578.857768333618878, 2244.547199809527683 ) ) ;
#16299=EDGE_CURVE ( 'NONE', #11298, #10072, #14325, .T. ) ;
#16301=CIRCLE ( 'NONE', #1720, 0.7619999999999987894 ) ;
#16302=ORIENTED_EDGE ( 'NONE', *, *, #17127, .T. ) ;
#16305=CARTESIAN_POINT ( 'NONE',  ( 95.25000000000000000, -3670.300000000000182, 2247.392000000000280 ) ) ;
#16306=CIRCLE ( 'NONE', #1320, 2.844800000000001550 ) ;
#16307=VERTEX_POINT ( 'NONE', #20296 ) ;
#16308=CARTESIAN_POINT ( 'NONE',  ( 151.1299999999999955, -3695.699999999999818, 2259.329999999999927 ) ) ;
#16310=CARTESIAN_POINT ( 'NONE',  ( 57.14999999999999858, -3568.700000000000273, 2247.392000000000280 ) ) ;
#16311=ADVANCED_FACE ( 'NONE', ( #9510 ), #8302, .F. ) ;
#16314=CARTESIAN_POINT ( 'NONE',  ( 9.971147940439486490, -3695.419680868843443, 2255.300839618168538 ) ) ;
#16316=CARTESIAN_POINT ( 'NONE',  ( 18.14575475405891680, -3581.228764778724781, 2245.816281745348988 ) ) ;
#16317=AXIS2_PLACEMENT_3D ( 'NONE', #15785, #19185, #20941 ) ;
#16319=ADVANCED_FACE ( 'NONE', ( #18841 ), #16652, .F. ) ;
#16322=CIRCLE ( 'NONE', #22658, 1.269999999999882334 ) ;
#16323=EDGE_CURVE ( 'NONE', #17137, #16091, #10192, .T. ) ;
#16324=VERTEX_POINT ( 'NONE', #7523 ) ;
#16325=ORIENTED_EDGE ( 'NONE', *, *, #1967, .F. ) ;
#16327=CARTESIAN_POINT ( 'NONE',  ( 140.6722870908654386, -3662.179796010951577, 2249.375424445521730 ) ) ;
#16328=AXIS2_PLACEMENT_3D ( 'NONE', #1400, #13831, #17329 ) ;
#16329=AXIS2_PLACEMENT_3D ( 'NONE', #5349, #3579, #17881 ) ;
#16330=EDGE_LOOP ( 'NONE', ( #2139, #2212, #7498, #2485, #6545, #6025, #10001, #477, #5671 ) ) ;
#16332=CARTESIAN_POINT ( 'NONE',  ( 41.70680000000000121, -3644.899999999999636, 2259.837999999999738 ) ) ;
#16333=ORIENTED_EDGE ( 'NONE', *, *, #18850, .F. ) ;
#16335=CARTESIAN_POINT ( 'NONE',  ( 0.000000000000000000, -3694.430000000000291, 2259.329999999999927 ) ) ;
#16338=CIRCLE ( 'NONE', #6243, 3.606799999998994366 ) ;
#16339=CARTESIAN_POINT ( 'NONE',  ( 79.80679999999999552, -3670.300000000000182, 2239.009999999999764 ) ) ;
#16342=DIRECTION ( 'NONE',  ( 0.000000000000000000, 0.000000000000000000, -1.000000000000000000 ) ) ;
#16344=AXIS2_PLACEMENT_3D ( 'NONE', #7000, #3462, #10263 ) ;
#16345=CARTESIAN_POINT ( 'NONE',  ( 131.9608861896474252, -3543.750038107418732, 2260.302253161996305 ) ) ;
#16346=VERTEX_POINT ( 'NONE', #10048 ) ;
#16347=DIRECTION ( 'NONE',  ( 0.000000000000000000, 0.000000000000000000, -1.000000000000000000 ) ) ;
#16348=CARTESIAN_POINT ( 'NONE',  ( 7.901418343680338019, -3662.609162415918490, 2245.978569001930282 ) ) ;
#16352=DIRECTION ( 'NONE',  ( 0.000000000000000000, -1.000000000000000000, 0.000000000000000000 ) ) ;
#16353=VECTOR ( 'NONE', #16747, 1000.000000000000000 ) ;
#16354=CARTESIAN_POINT ( 'NONE',  ( 47.19319999999999737, -3670.300000000000182, 2239.771999999999935 ) ) ;
#16357=CARTESIAN_POINT ( 'NONE',  ( 18.03944995089040049, -3657.466237342172008, 2246.412073519087699 ) ) ;
#16358=AXIS2_PLACEMENT_3D ( 'NONE', #307, #7451, #14604 ) ;
#16360=CARTESIAN_POINT ( 'NONE',  ( 147.6747367346642932, -3695.644174308748461, 2259.712265308950464 ) ) ;
#16364=CARTESIAN_POINT ( 'NONE',  ( 4.572920519510999426, -3695.699999999999818, 2259.329999999999927 ) ) ;
#16365=CARTESIAN_POINT ( 'NONE',  ( 136.9721883683046997, -3695.420022019528915, 2255.303812753265902 ) ) ;
#16366=CARTESIAN_POINT ( 'NONE',  ( 7.834124089763437659, -3576.497611619219697, 2245.807063631086294 ) ) ;
#16367=ORIENTED_EDGE ( 'NONE', *, *, #15390, .F. ) ;
#16370=ADVANCED_FACE ( 'NONE', ( #17194 ), #18186, .F. ) ;
#16374=ADVANCED_FACE ( 'NONE', ( #19954 ), #18300, .F. ) ;
#16375=AXIS2_PLACEMENT_3D ( 'NONE', #1741, #1610, #6903 ) ;
#16379=DIRECTION ( 'NONE',  ( 0.000000000000000000, 0.000000000000000000, 1.000000000000000000 ) ) ;
#16380=VERTEX_POINT ( 'NONE', #20073 ) ;
#16383=CARTESIAN_POINT ( 'NONE',  ( 18.01287425286000143, -3581.600847139000052, 2246.630000000000109 ) ) ;
#16385=CARTESIAN_POINT ( 'NONE',  ( 12.31593207299000170, -3694.430000000000291, 2251.974139024000124 ) ) ;
#16386=ORIENTED_EDGE ( 'NONE', *, *, #8593, .T. ) ;
#16387=CYLINDRICAL_SURFACE ( 'NONE', #21546, 2.844800000000091700 ) ;
#16389=CARTESIAN_POINT ( 'NONE',  ( 142.4276778852931784, -3695.420022016050098, 2255.303759356630508 ) ) ;
#16391=ORIENTED_EDGE ( 'NONE', *, *, #17954, .F. ) ;
#16393=CARTESIAN_POINT ( 'NONE',  ( 137.7588963307679251, -3581.574831038090906, 2248.242363506559286 ) ) ;
#16398=ADVANCED_FACE ( 'NONE', ( #12285 ), #103, .T. ) ;
#16400=DIRECTION ( 'NONE',  ( 0.000000000000000000, 0.000000000000000000, -1.000000000000000000 ) ) ;
#16402=CARTESIAN_POINT ( 'NONE',  ( 131.8084957954999936, -3544.527728344000025, 2260.600000000000364 ) ) ;
#16404=CARTESIAN_POINT ( 'NONE',  ( 140.5570903332553030, -3576.782304280421613, 2249.335231873303655 ) ) ;
#16405=ORIENTED_EDGE ( 'NONE', *, *, #9831, .F. ) ;
#16406=CARTESIAN_POINT ( 'NONE',  ( 105.2067999999999870, -3619.500000000000000, 2239.009999999999764 ) ) ;
#16407=DIRECTION ( 'NONE',  ( 1.000000000000000000, 0.000000000000000000, 0.000000000000000000 ) ) ;
#16408=ORIENTED_EDGE ( 'NONE', *, *, #14891, .T. ) ;
#16422=CARTESIAN_POINT ( 'NONE',  ( 21.79320000000099711, -3568.700000000000273, 2239.009999999999764 ) ) ;
#16425=PLANE ( 'NONE',  #19746 ) ;
#16426=DIRECTION ( 'NONE',  ( 0.000000000000000000, 0.000000000000000000, -1.000000000000000000 ) ) ;
#16427=ORIENTED_EDGE ( 'NONE', *, *, #956, .T. ) ;
#16428=CARTESIAN_POINT ( 'NONE',  ( 18.01287425286000143, -3581.600847139000052, 2246.630000000000109 ) ) ;
#16430=DIRECTION ( 'NONE',  ( 0.000000000000000000, -1.000000000000000000, 0.000000000000000000 ) ) ;
#16431=ADVANCED_FACE ( 'NONE', ( #12162 ), #3483, .F. ) ;
#16433=CIRCLE ( 'NONE', #7839, 6.477000000000000313 ) ;
#16434=CARTESIAN_POINT ( 'NONE',  ( 138.8069558488828932, -3662.206088545077819, 2249.347568272374701 ) ) ;
#16435=VERTEX_POINT ( 'NONE', #21310 ) ;
#16437=EDGE_LOOP ( 'NONE', ( #22745, #17739 ) ) ;
#16438=DIRECTION ( 'NONE',  ( 0.000000000000000000, 0.000000000000000000, -1.000000000000000000 ) ) ;
#16439=ORIENTED_EDGE ( 'NONE', *, *, #5272, .F. ) ;
#16440=ORIENTED_EDGE ( 'NONE', *, *, #19258, .T. ) ;
#16441=CARTESIAN_POINT ( 'NONE',  ( 15.24000000000000021, -3658.223872745999870, 2255.774000000000342 ) ) ;
#16442=CARTESIAN_POINT ( 'NONE',  ( 101.5999999999999943, -3619.500000000000000, 2239.771999999999935 ) ) ;
#16443=EDGE_CURVE ( 'NONE', #14575, #4022, #20837, .T. ) ;
#16444=EDGE_LOOP ( 'NONE', ( #2830, #21607, #8600, #9250 ) ) ;
#16447=CARTESIAN_POINT ( 'NONE',  ( 7.306649500355966609, -3581.385628413785980, 2246.082317946663352 ) ) ;
#16448=CARTESIAN_POINT ( 'NONE',  ( 95.25000000000000000, -3694.430000000000291, 2247.392000000000280 ) ) ;
#16452=DIRECTION ( 'NONE',  ( 1.000000000000000000, 0.000000000000000000, 0.000000000000000000 ) ) ;
#16454=EDGE_LOOP ( 'NONE', ( #6915, #19578, #5037, #22475 ) ) ;
#16455=CARTESIAN_POINT ( 'NONE',  ( 7.020566483207999475, -3660.139755500999854, 2244.547200037999573 ) ) ;
#16459=AXIS2_PLACEMENT_3D ( 'NONE', #18269, #20267, #18154 ) ;
#16461=CARTESIAN_POINT ( 'NONE',  ( 63.50000000000000000, -3644.899999999999636, 2239.771999999999935 ) ) ;
#16465=ORIENTED_EDGE ( 'NONE', *, *, #9713, .T. ) ;
#16466=CARTESIAN_POINT ( 'NONE',  ( 18.16341182905199503, -3657.827357193916214, 2245.734039593747639 ) ) ;
#16467=ORIENTED_EDGE ( 'NONE', *, *, #5955, .F. ) ;
#16470=CARTESIAN_POINT ( 'NONE',  ( 29.00679999999900005, -3670.300000000000182, 2260.600000000000364 ) ) ;
#16472=CARTESIAN_POINT ( 'NONE',  ( 127.0000000000000000, -3578.860000000000127, 2247.392000000000280 ) ) ;
#16473=DIRECTION ( 'NONE',  ( 0.000000000000000000, 0.000000000000000000, 1.000000000000000000 ) ) ;
#16475=CARTESIAN_POINT ( 'NONE',  ( 7.579779957786826117, -3576.956500483505806, 2245.277209879519887 ) ) ;
#16476=EDGE_LOOP ( 'NONE', ( #17414, #11215 ) ) ;
#16478=TOROIDAL_SURFACE ( 'NONE', #12364, 3.606799999998999695, 0.7620000000000000107 ) ;
#16484=CARTESIAN_POINT ( 'NONE',  ( 41.70680000000000121, -3594.099999999999909, 2239.771999999999935 ) ) ;
#16487=CARTESIAN_POINT ( 'NONE',  ( 134.9639022863356388, -3662.704503798480346, 2246.158276165796451 ) ) ;
#16489=ORIENTED_EDGE ( 'NONE', *, *, #4200, .F. ) ;
#16491=ORIENTED_EDGE ( 'NONE', *, *, #23005, .F. ) ;
#16496=DIRECTION ( 'NONE',  ( 0.000000000000000000, 0.000000000000000000, -1.000000000000000000 ) ) ;
#16498=CARTESIAN_POINT ( 'NONE',  ( 1.270000000000000018, -3544.570000000000164, 2259.329999999999927 ) ) ;
#16501=CARTESIAN_POINT ( 'NONE',  ( 1.270000000000000018, -3578.860000000000127, 2251.506800000000112 ) ) ;
#16503=AXIS2_PLACEMENT_3D ( 'NONE', #6506, #6281, #20663 ) ;
#16504=UNCERTAINTY_MEASURE_WITH_UNIT (LENGTH_MEASURE( 1.000000000000000082E-05 ), #20317, 'distance_accuracy_value', 'NONE');
#16506=CARTESIAN_POINT ( 'NONE',  ( 145.2441493676143409, -3580.882459096562343, 2245.390311603773625 ) ) ;
#16508=CARTESIAN_POINT ( 'NONE',  ( 57.14999999999999858, -3568.700000000000273, 2244.547199999999975 ) ) ;
#16509=DIRECTION ( 'NONE',  ( 0.000000000000000000, 1.000000000000000000, 0.000000000000000000 ) ) ;
#16510=DIRECTION ( 'NONE',  ( 0.000000000000000000, -1.000000000000000000, 0.000000000000000000 ) ) ;
#16512=DIRECTION ( 'NONE',  ( 1.000000000000000000, 0.000000000000000000, 0.000000000000000000 ) ) ;
#16513=CARTESIAN_POINT ( 'NONE',  ( 138.9527035083802105, -3576.750047203152462, 2249.300150270811173 ) ) ;
#16517=ADVANCED_FACE ( 'NONE', ( #8542 ), #3255, .F. ) ;
#16518=VERTEX_POINT ( 'NONE', #11928 ) ;
#16519=CARTESIAN_POINT ( 'NONE',  ( 145.0128742528999908, -3581.600847139000052, 2246.630000000000109 ) ) ;
#16522=CARTESIAN_POINT ( 'NONE',  ( 142.2400000000000091, -3695.699999999999818, 2255.774000000000342 ) ) ;
#16523=CARTESIAN_POINT ( 'NONE',  ( 15.55234650392334927, -3543.397347667163558, 2254.991636092748649 ) ) ;
#16524=EDGE_CURVE ( 'NONE', #1541, #21716, #17295, .T. ) ;
#16525=ORIENTED_EDGE ( 'NONE', *, *, #15898, .F. ) ;
#16528=EDGE_LOOP ( 'NONE', ( #20337, #18149 ) ) ;
#16530=CARTESIAN_POINT ( 'NONE',  ( 15.15611746081473399, -3578.059478917778051, 2250.121899032252259 ) ) ;
#16533=DIRECTION ( 'NONE',  ( 1.000000000000000000, 0.000000000000000000, 0.000000000000000000 ) ) ;
#16534=VERTEX_POINT ( 'NONE', #13923 ) ;
#16535=AXIS2_PLACEMENT_3D ( 'NONE', #21508, #5338, #2174 ) ;
#16536=CARTESIAN_POINT ( 'NONE',  ( 92.50679999999999836, -3594.099999999999909, 2259.837999999999738 ) ) ;
#16538=AXIS2_PLACEMENT_3D ( 'NONE', #22141, #924, #22027 ) ;
#16539=DIRECTION ( 'NONE',  ( 0.000000000000000000, 0.000000000000000000, 1.000000000000000000 ) ) ;
#16542=CARTESIAN_POINT ( 'NONE',  ( 18.24414936330329340, -3580.882459114104677, 2245.390311621496039 ) ) ;
#16543=ADVANCED_FACE ( 'NONE', ( #21073 ), #6900, .F. ) ;
#16545=ORIENTED_EDGE ( 'NONE', *, *, #6952, .F. ) ;
#16546=VERTEX_POINT ( 'NONE', #10756 ) ;
#16548=AXIS2_PLACEMENT_3D ( 'NONE', #19757, #14594, #7216 ) ;
#16549=CARTESIAN_POINT ( 'NONE',  ( 137.4648769445816754, -3661.265785465956469, 2250.004993578675567 ) ) ;
#16550=ORIENTED_EDGE ( 'NONE', *, *, #21561, .F. ) ;
#16555=CARTESIAN_POINT ( 'NONE',  ( 50.79999999999999716, -3670.300000000000182, 2260.600000000000364 ) ) ;
#16556=VERTEX_POINT ( 'NONE', #9347 ) ;
#16559=EDGE_CURVE ( 'NONE', #8087, #18027, #13933, .T. ) ;
#16561=EDGE_CURVE ( 'NONE', #7890, #22920, #16173, .T. ) ;
#16562=CARTESIAN_POINT ( 'NONE',  ( 7.038650801644599220, -3658.717805898987535, 2244.925821907141199 ) ) ;
#16563=DIRECTION ( 'NONE',  ( -1.000000000000000000, 0.000000000000000000, 0.000000000000000000 ) ) ;
#16564=FACE_OUTER_BOUND ( 'NONE', #19942, .T. ) ;
#16570=CARTESIAN_POINT ( 'NONE',  ( 142.4905652536138234, -3658.950617808927291, 2249.976257908279877 ) ) ;
#16571=CARTESIAN_POINT ( 'NONE',  ( 7.837774371996756528, -3662.508315729218339, 2245.815813615873139 ) ) ;
#16576=CIRCLE ( 'NONE', #10220, 1.269999999999882334 ) ;
#16577=FACE_OUTER_BOUND ( 'NONE', #20413, .T. ) ;
#16578=CARTESIAN_POINT ( 'NONE',  ( 147.6177065956714785, -3543.413280444305656, 2259.854323493447282 ) ) ;
#16583=CIRCLE ( 'NONE', #18459, 1.269999999999882334 ) ;
#16585=ADVANCED_FACE ( 'NONE', ( #21422 ), #93, .T. ) ;
#16586=EDGE_CURVE ( 'NONE', #15612, #287, #15435, .T. ) ;
#16589=DIRECTION ( 'NONE',  ( 0.000000000000000000, 0.000000000000000000, 1.000000000000000000 ) ) ;
#16591=CARTESIAN_POINT ( 'NONE',  ( 95.25000000000000000, -3568.700000000000273, 2250.236800000000130 ) ) ;
#16594=ORIENTED_EDGE ( 'NONE', *, *, #4085, .T. ) ;
#16596=CARTESIAN_POINT ( 'NONE',  ( 145.1168285562762890, -3657.683068618205198, 2245.957879822228278 ) ) ;
#16598=CIRCLE ( 'NONE', #18104, 2.844800000000091700 ) ;
#16599=DIRECTION ( 'NONE',  ( 0.000000000000000000, 0.000000000000000000, 1.000000000000000000 ) ) ;
#16608=DIRECTION ( 'NONE',  ( 0.000000000000000000, 1.000000000000000000, 0.000000000000000000 ) ) ;
#16609=EDGE_LOOP ( 'NONE', ( #18160, #14828 ) ) ;
#16619=CARTESIAN_POINT ( 'NONE',  ( 145.3787162833025377, -3580.137931053215198, 2244.850299910533977 ) ) ;
#16621=CARTESIAN_POINT ( 'NONE',  ( 17.83565360962044721, -3662.011901429552381, 2245.249457087976225 ) ) ;
#16623=FACE_OUTER_BOUND ( 'NONE', #5015, .T. ) ;
#16627=CARTESIAN_POINT ( 'NONE',  ( 142.4730239663999782, -3578.859999866000180, 2250.236800057000437 ) ) ;
#16629=ORIENTED_EDGE ( 'NONE', *, *, #6674, .T. ) ;
#16633=CARTESIAN_POINT ( 'NONE',  ( 142.5447999999993272, -3659.053785370568221, 2256.063560000000962 ) ) ;
#16634=VERTEX_POINT ( 'NONE', #7362 ) ;
#16635=LINE ( 'NONE', #11482, #12426 ) ;
#16642=DIRECTION ( 'NONE',  ( 0.000000000000000000, 0.000000000000000000, -1.000000000000000000 ) ) ;
#16643=CARTESIAN_POINT ( 'NONE',  ( 14.51593956253670825, -3577.305016495025484, 2249.774268863664020 ) ) ;
#16645=AXIS2_PLACEMENT_3D ( 'NONE', #4370, #2500, #11284 ) ;
#16646=DIRECTION ( 'NONE',  ( 0.000000000000000000, 0.000000000000000000, 1.000000000000000000 ) ) ;
#16647=VERTEX_POINT ( 'NONE', #18355 ) ;
#16648=LINE ( 'NONE', #14910, #2895 ) ;
#16651=DIRECTION ( 'NONE',  ( -1.000000000000000000, 0.000000000000000000, 0.000000000000000000 ) ) ;
#16652=CYLINDRICAL_SURFACE ( 'NONE', #8697, 2.844799999998995244 ) ;
#16653=EDGE_LOOP ( 'NONE', ( #1627, #881, #1730, #5707, #16408, #18700, #16427, #21328, #18123, #22139 ) ) ;
#16656=ADVANCED_FACE ( 'NONE', ( #19784 ), #16258, .T. ) ;
#16658=AXIS2_PLACEMENT_3D ( 'NONE', #13152, #11280, #4470 ) ;
#16660=CARTESIAN_POINT ( 'NONE',  ( 140.3462183034946520, -3662.275628691427301, 2249.271390612719188 ) ) ;
#16661=AXIS2_PLACEMENT_3D ( 'NONE', #8582, #13743, #15728 ) ;
#16665=DIRECTION ( 'NONE',  ( -1.000000000000000000, 0.000000000000000000, 0.000000000000000000 ) ) ;
#16671=DIRECTION ( 'NONE',  ( 0.000000000000000000, 0.000000000000000000, -1.000000000000000000 ) ) ;
#16681=EDGE_CURVE ( 'NONE', #16201, #20008, #9796, .T. ) ;
#16683=CARTESIAN_POINT ( 'NONE',  ( 142.3444509448549979, -3658.456267385442970, 2249.685054683717681 ) ) ;
#16686=CIRCLE ( 'NONE', #11071, 0.7619999999999294005 ) ;
#16687=EDGE_LOOP ( 'NONE', ( #22722, #7077, #22628, #7502 ) ) ;
#16688=DIRECTION ( 'NONE',  ( 0.000000000000000000, 0.000000000000000000, -1.000000000000000000 ) ) ;
#16691=VERTEX_POINT ( 'NONE', #22431 ) ;
#16692=AXIS2_PLACEMENT_3D ( 'NONE', #16332, #21493, #9186 ) ;
#16696=CARTESIAN_POINT ( 'NONE',  ( 18.26004394573143941, -3658.183240515012130, 2245.327057614696514 ) ) ;
#16698=ORIENTED_EDGE ( 'NONE', *, *, #11861, .T. ) ;
#16699=CARTESIAN_POINT ( 'NONE',  ( 147.4602137133928466, -3695.306816721560153, 2260.248793245645629 ) ) ;
#16703=DIRECTION ( 'NONE',  ( 0.000000000000000000, 0.000000000000000000, -1.000000000000000000 ) ) ;
#16705=DIRECTION ( 'NONE',  ( 0.000000000000000000, 0.000000000000000000, -1.000000000000000000 ) ) ;
#16706=CARTESIAN_POINT ( 'NONE',  ( 7.643488289160662141, -3576.831741762340243, 2245.397138245397400 ) ) ;
#16709=EDGE_CURVE ( 'NONE', #14725, #21716, #14686, .T. ) ;
#16710=CARTESIAN_POINT ( 'NONE',  ( 145.1202614246111580, -3657.693328148723140, 2245.940466390600250 ) ) ;
#16711=FACE_OUTER_BOUND ( 'NONE', #14567, .T. ) ;
#16712=AXIS2_PLACEMENT_3D ( 'NONE', #13860, #21010, #12097 ) ;
#16713=CYLINDRICAL_SURFACE ( 'NONE', #11598, 2.844800000000001550 ) ;
#16714=AXIS2_PLACEMENT_3D ( 'NONE', #1384, #17314, #1259 ) ;
#16717=CARTESIAN_POINT ( 'NONE',  ( 134.1072540231934624, -3660.723001229534020, 2244.591060091476265 ) ) ;
#16721=DIRECTION ( 'NONE',  ( 1.000000000000000000, 0.000000000000000000, 0.000000000000000000 ) ) ;
#16723=B_SPLINE_CURVE_WITH_KNOTS ( 'NONE', 3,
 ( #13180, #16808, #20447, #2629, #9885, #18914 ),
 .UNSPECIFIED., .F., .F.,
 ( 4, 1, 1, 4 ),
 ( 0.000000000000000000, 0.3333333333333000081, 0.6666666666667000474, 1.000000000000000000 ),
 .UNSPECIFIED. ) ;
#16724=CARTESIAN_POINT ( 'NONE',  ( 13.44550029692929272, -3662.251450944823318, 2249.298748438002804 ) ) ;
#16725=CARTESIAN_POINT ( 'NONE',  ( 15.54479951278000094, -3579.494996001999880, 2250.165024905999871 ) ) ;
#16727=EDGE_CURVE ( 'NONE', #3620, #2616, #1196, .T. ) ;
#16729=AXIS2_PLACEMENT_3D ( 'NONE', #10780, #9263, #2228 ) ;
#16733=DIRECTION ( 'NONE',  ( 0.000000000000000000, 0.000000000000000000, 1.000000000000000000 ) ) ;
#16734=CARTESIAN_POINT ( 'NONE',  ( 38.10000000000000142, -3644.899999999999636, 2260.600000000000364 ) ) ;
#16737=AXIS2_PLACEMENT_3D ( 'NONE', #9571, #18130, #14743 ) ;
#16740=FACE_OUTER_BOUND ( 'NONE', #17894, .T. ) ;
#16741=UNCERTAINTY_MEASURE_WITH_UNIT (LENGTH_MEASURE( 1.000000000000000082E-05 ), #21126, 'distance_accuracy_value', 'NONE');
#16745=DIRECTION ( 'NONE',  ( -1.000000000000000000, 0.000000000000000000, 0.000000000000000000 ) ) ;
#16746=DIRECTION ( 'NONE',  ( 0.000000000000000000, 0.000000000000000000, -1.000000000000000000 ) ) ;
#16747=DIRECTION ( 'NONE',  ( 0.000000000000000000, -1.000000000000000000, 0.000000000000000000 ) ) ;
#16748=CARTESIAN_POINT ( 'NONE',  ( 145.3796772601000100, -3660.139769217999856, 2244.548186305999934 ) ) ;
#16749=AXIS2_PLACEMENT_3D ( 'NONE', #1253, #22809, #12159 ) ;
#16750=ADVANCED_FACE ( 'NONE', ( #14961 ), #875, .F. ) ;
#16752=VERTEX_POINT ( 'NONE', #7692 ) ;
#16754=VECTOR ( 'NONE', #8135, 1000.000000000000000 ) ;
#16759=CARTESIAN_POINT ( 'NONE',  ( 15.39362723101645969, -3543.659322603280998, 2255.389249077201384 ) ) ;
#16761=VERTEX_POINT ( 'NONE', #764 ) ;
#16762=DIRECTION ( 'NONE',  ( -1.000000000000000000, 0.000000000000000000, 0.000000000000000000 ) ) ;
#16764=CIRCLE ( 'NONE', #16036, 0.7619999999999987894 ) ;
#16766=CARTESIAN_POINT ( 'NONE',  ( 14.06012086060861854, -3576.995964396000545, 2249.541211835891318 ) ) ;
#16767=CARTESIAN_POINT ( 'NONE',  ( 142.1404520028303011, -3580.959877191935448, 2249.315266803219856 ) ) ;
#16769=CARTESIAN_POINT ( 'NONE',  ( 35.56000000000000227, -3544.570000000000164, 2244.547199999999975 ) ) ;
#16773=CARTESIAN_POINT ( 'NONE',  ( 136.8551930557000276, -3659.505009668000184, 2250.165028799000083 ) ) ;
#16778=FACE_OUTER_BOUND ( 'NONE', #12356, .T. ) ;
#16780=ADVANCED_FACE ( 'NONE', ( #16711 ), #14856, .F. ) ;
#16782=DIRECTION ( 'NONE',  ( 1.000000000000000000, 0.000000000000000000, 0.000000000000000000 ) ) ;
#16783=PLANE ( 'NONE',  #3176 ) ;
#16785=CARTESIAN_POINT ( 'NONE',  ( 7.273601599882602464, -3657.711793654752910, 2245.909852404346566 ) ) ;
#16787=DIRECTION ( 'NONE',  ( 0.000000000000000000, 0.000000000000000000, 1.000000000000000000 ) ) ;
#16791=EDGE_LOOP ( 'NONE', ( #13872, #5565, #7143, #22765 ) ) ;
#16794=CARTESIAN_POINT ( 'NONE',  ( 142.5038613777062437, -3659.021559187911862, 2250.007933345488709 ) ) ;
#16795=DIRECTION ( 'NONE',  ( 0.000000000000000000, 0.000000000000000000, -1.000000000000000000 ) ) ;
#16796=ORIENTED_EDGE ( 'NONE', *, *, #3137, .F. ) ;
#16801=DIRECTION ( 'NONE',  ( 0.000000000000000000, 0.000000000000000000, -1.000000000000000000 ) ) ;
#16804=ORIENTED_EDGE ( 'NONE', *, *, #8644, .F. ) ;
#16807=EDGE_CURVE ( 'NONE', #7313, #8026, #18499, .T. ) ;
#16808=CARTESIAN_POINT ( 'NONE',  ( 20.31206600734000034, -3694.758336080999925, 2260.533847755999886 ) ) ;
#16810=DIRECTION ( 'NONE',  ( 0.000000000000000000, 0.000000000000000000, -1.000000000000000000 ) ) ;
#16811=EDGE_CURVE ( 'NONE', #11524, #5223, #2335, .T. ) ;
#16814=CARTESIAN_POINT ( 'NONE',  ( 8.037678690397633829, -3576.188730137088442, 2246.379736642491480 ) ) ;
#16815=ORIENTED_EDGE ( 'NONE', *, *, #17665, .T. ) ;
#16817=CARTESIAN_POINT ( 'NONE',  ( 105.2067999999999870, -3670.300000000000182, 2239.771999999999935 ) ) ;
#16819=CARTESIAN_POINT ( 'NONE',  ( 9.926995637850000165, -3660.140002548000211, 2250.236801297000056 ) ) ;
#16821=EDGE_CURVE ( 'NONE', #20008, #16201, #18057, .T. ) ;
#16822=CIRCLE ( 'NONE', #8976, 6.477000000000000313 ) ;
#16824=CARTESIAN_POINT ( 'NONE',  ( 134.0525542150678291, -3660.427269758552029, 2244.547227117760031 ) ) ;
#16825=DIRECTION ( 'NONE',  ( 1.000000000000000000, 0.000000000000000000, 0.000000000000000000 ) ) ;
#16826=CARTESIAN_POINT ( 'NONE',  ( 134.5329181263396094, -3577.053440065938503, 2245.194077375531833 ) ) ;
#16827=ORIENTED_EDGE ( 'NONE', *, *, #15747, .F. ) ;
#16829=FACE_OUTER_BOUND ( 'NONE', #13654, .T. ) ;
#16830=CARTESIAN_POINT ( 'NONE',  ( 95.25000000000000000, -3543.300000000000182, 2251.506800000000112 ) ) ;
#16834=AXIS2_PLACEMENT_3D ( 'NONE', #17079, #4660, #4897 ) ;
#16837=DIRECTION ( 'NONE',  ( -1.000000000000000000, 0.000000000000000000, 0.000000000000000000 ) ) ;
#16839=VERTEX_POINT ( 'NONE', #21046 ) ;
#16840=EDGE_CURVE ( 'NONE', #16546, #19496, #22155, .T. ) ;
#16842=CIRCLE ( 'NONE', #6762, 2.844799999998897988 ) ;
#16845=CARTESIAN_POINT ( 'NONE',  ( 145.3744937373275832, -3580.174051493410389, 2244.868862703849118 ) ) ;
#16847=CARTESIAN_POINT ( 'NONE',  ( 145.3976541156836788, -3579.044846244369637, 2244.552343491880492 ) ) ;
#16848=CARTESIAN_POINT ( 'NONE',  ( 17.56682579340610673, -3662.500841285317165, 2245.804760078034178 ) ) ;
#16849=CIRCLE ( 'NONE', #760, 0.7619999999999987894 ) ;
#16850=DIRECTION ( 'NONE',  ( 0.000000000000000000, 1.000000000000000000, 0.000000000000000000 ) ) ;
#16851=CARTESIAN_POINT ( 'NONE',  ( 151.1299999999999955, -3544.570000000000164, 2240.279999999999745 ) ) ;
#16853=CARTESIAN_POINT ( 'NONE',  ( 116.8400000000000034, -3544.570000000000164, 2247.392000000000280 ) ) ;
#16857=DIRECTION ( 'NONE',  ( 0.000000000000000000, 0.000000000000000000, -1.000000000000000000 ) ) ;
#16860=ORIENTED_EDGE ( 'NONE', *, *, #5980, .T. ) ;
#16864=AXIS2_PLACEMENT_3D ( 'NONE', #16917, #862, #8028 ) ;
#16866=ORIENTED_EDGE ( 'NONE', *, *, #22160, .F. ) ;
#16869=DIRECTION ( 'NONE',  ( -1.000000000000000000, 0.000000000000000000, 0.000000000000000000 ) ) ;
#16870=EDGE_CURVE ( 'NONE', #22886, #18714, #20303, .T. ) ;
#16871=CARTESIAN_POINT ( 'NONE',  ( 11.90373727042107355, -3576.763824424820086, 2249.315280365585750 ) ) ;
#16873=CARTESIAN_POINT ( 'NONE',  ( 142.4777174751457380, -3580.110796106637736, 2249.947098715658285 ) ) ;
#16874=ORIENTED_EDGE ( 'NONE', *, *, #18110, .T. ) ;
#16881=PRODUCT ( 'Base Plate', 'Base Plate', '', ( #7841 ) ) ;
#16882=FACE_OUTER_BOUND ( 'NONE', #4652, .T. ) ;
#16883=CIRCLE ( 'NONE', #17262, 3.606799999999993567 ) ;
#16885=EDGE_CURVE ( 'NONE', #9004, #4163, #2688, .T. ) ;
#16887=EDGE_CURVE ( 'NONE', #20367, #5163, #12433, .T. ) ;
#16893=DIRECTION ( 'NONE',  ( 0.000000000000000000, 0.000000000000000000, -1.000000000000000000 ) ) ;
#16894=AXIS2_PLACEMENT_3D ( 'NONE', #16902, #9756, #11622 ) ;
#16898=SHAPE_REPRESENTATION_RELATIONSHIP ( 'NONE' , 'NONE' ,  #7730, #21380 ) ;
#16902=CARTESIAN_POINT ( 'NONE',  ( 76.20000000000000284, -3568.700000000000273, 2261.869999999999891 ) ) ;
#16909=EDGE_LOOP ( 'NONE', ( #1754, #11099, #20732, #13093 ) ) ;
#16914=DIRECTION ( 'NONE',  ( -1.224646799147353207E-16, 1.000000000000000000, 0.000000000000000000 ) ) ;
#16915=ORIENTED_EDGE ( 'NONE', *, *, #10850, .F. ) ;
#16917=CARTESIAN_POINT ( 'NONE',  ( 136.2852881834000129, -3544.570000000000164, 2254.853250718999789 ) ) ;
#16919=AXIS2_PLACEMENT_3D ( 'NONE', #16289, #10433, #14543 ) ;
#16921=DIRECTION ( 'NONE',  ( 1.000000000000000000, 0.000000000000000000, 0.000000000000000000 ) ) ;
#16922=CARTESIAN_POINT ( 'NONE',  ( 142.4431999999993366, -3578.616742952568075, 2255.967040000000907 ) ) ;
#16924=CARTESIAN_POINT ( 'NONE',  ( 20.53015091878355491, -3695.459526430383903, 2260.073662062739913 ) ) ;
#16925=ORIENTED_EDGE ( 'NONE', *, *, #8673, .F. ) ;
#16928=AXIS2_PLACEMENT_3D ( 'NONE', #12329, #8817, #10215 ) ;
#16935=ORIENTED_EDGE ( 'NONE', *, *, #6674, .F. ) ;
#16937=CARTESIAN_POINT ( 'NONE',  ( 25.39999999999999858, -3568.700000000000273, 2239.009999999999764 ) ) ;
#16938=EDGE_CURVE ( 'NONE', #16647, #10320, #7937, .T. ) ;
#16940=CARTESIAN_POINT ( 'NONE',  ( 134.1465012860365675, -3578.137695944618372, 2244.636253112222221 ) ) ;
#16942=AXIS2_PLACEMENT_3D ( 'NONE', #19249, #6951, #3184 ) ;
#16943=CARTESIAN_POINT ( 'NONE',  ( 79.80679999999999552, -3670.300000000000182, 2260.600000000000364 ) ) ;
#16945=AXIS2_PLACEMENT_3D ( 'NONE', #11855, #2947, #6822 ) ;
#16947=ORIENTED_EDGE ( 'NONE', *, *, #11771, .F. ) ;
#16948=EDGE_CURVE ( 'NONE', #15032, #7066, #14365, .T. ) ;
#16949=CARTESIAN_POINT ( 'NONE',  ( 1.270000000000000018, -3544.570000000000164, 2259.329999999999927 ) ) ;
#16952=DIRECTION ( 'NONE',  ( -1.000000000000000000, 0.000000000000000000, 0.000000000000000000 ) ) ;
#16953=CARTESIAN_POINT ( 'NONE',  ( 76.20000000000000284, -3568.700000000000273, 2260.600000000000364 ) ) ;
#16955=ORIENTED_EDGE ( 'NONE', *, *, #7098, .T. ) ;
#16956=CIRCLE ( 'NONE', #6876, 3.606800000000000228 ) ;
#16957=ORIENTED_EDGE ( 'NONE', *, *, #15817, .F. ) ;
#16964=CARTESIAN_POINT ( 'NONE',  ( 17.93858170739038371, -3661.789460736868023, 2245.074020119504439 ) ) ;
#16966=ADVANCED_FACE ( 'NONE', ( #12484 ), #11661, .T. ) ;
#16967=CARTESIAN_POINT ( 'NONE',  ( 137.1599999999999966, -3660.786127253999894, 2255.774000000000342 ) ) ;
#16970=CARTESIAN_POINT ( 'NONE',  ( 136.9932263412491693, -3578.570683720540728, 2250.236800207163924 ) ) ;
#16971=ORIENTED_EDGE ( 'NONE', *, *, #13966, .T. ) ;
#16972=AXIS2_PLACEMENT_3D ( 'NONE', #15716, #19577, #5177 ) ;
#16976=LINE ( 'NONE', #6447, #15530 ) ;
#16978=VERTEX_POINT ( 'NONE', #12606 ) ;
#16980=ORIENTED_EDGE ( 'NONE', *, *, #12705, .T. ) ;
#16982=ORIENTED_EDGE ( 'NONE', *, *, #21318, .T. ) ;
#16984=CARTESIAN_POINT ( 'NONE',  ( 11.61431908031736171, -3576.865156646217201, 2249.420288324090507 ) ) ;
#16985=CARTESIAN_POINT ( 'NONE',  ( 141.8090081642606322, -3581.404182753561145, 2248.664805393861116 ) ) ;
#16987=DIRECTION ( 'NONE',  ( -1.000000000000000000, 0.000000000000000000, 0.000000000000000000 ) ) ;
#16993=CARTESIAN_POINT ( 'NONE',  ( 134.2595036476987502, -3657.754874278681200, 2245.841254873516846 ) ) ;
#16996=EDGE_CURVE ( 'NONE', #20246, #10320, #8708, .T. ) ;
#16997=EDGE_CURVE ( 'NONE', #8573, #7121, #19513, .T. ) ;
#17000=B_SPLINE_CURVE_WITH_KNOTS ( 'NONE', 3,
 ( #14153, #12032, #19414, #19303 ),
 .UNSPECIFIED., .F., .F.,
 ( 4, 4 ),
 ( 0.000000000000000000, 1.000000000000000000 ),
 .UNSPECIFIED. ) ;
#17003=AXIS2_PLACEMENT_3D ( 'NONE', #11528, #745, #9545 ) ;
#17009=DIRECTION ( 'NONE',  ( 1.000000000000000000, 0.000000000000000000, 0.000000000000000000 ) ) ;
#17011=ORIENTED_EDGE ( 'NONE', *, *, #12458, .T. ) ;
#17012=CARTESIAN_POINT ( 'NONE',  ( 7.172952441013247693, -3658.051458389673371, 2245.460178138798256 ) ) ;
#17015=DIRECTION ( 'NONE',  ( 1.000000000000000000, 0.000000000000000000, 0.000000000000000000 ) ) ;
#17016=EDGE_CURVE ( 'NONE', #17151, #7277, #9461, .T. ) ;
#17022=DIRECTION ( 'NONE',  ( 0.000000000000000000, 0.000000000000000000, 1.000000000000000000 ) ) ;
#17025=DIRECTION ( 'NONE',  ( 0.000000000000000000, 0.000000000000000000, 1.000000000000000000 ) ) ;
#17026=EDGE_CURVE ( 'NONE', #13045, #14116, #20320, .T. ) ;
#17028=EDGE_LOOP ( 'NONE', ( #16982, #14922, #11044, #2539, #18429 ) ) ;
#17030=CARTESIAN_POINT ( 'NONE',  ( 18.30933195705248195, -3658.407053146634553, 2245.132319941641526 ) ) ;
#17034=CARTESIAN_POINT ( 'NONE',  ( 18.40320150486666506, -3579.070516913197025, 2244.547180105589632 ) ) ;
#17035=AXIS2_PLACEMENT_3D ( 'NONE', #19439, #12408, #21209 ) ;
#17037=DIRECTION ( 'NONE',  ( -1.000000000000000000, 0.000000000000000000, 0.000000000000000000 ) ) ;
#17045=CARTESIAN_POINT ( 'NONE',  ( 145.3463507443650258, -3658.589118495387083, 2244.993626476412828 ) ) ;
#17047=CARTESIAN_POINT ( 'NONE',  ( 57.14999999999999858, -3543.299999999999727, 2247.392000000000280 ) ) ;
#17049=ORIENTED_EDGE ( 'NONE', *, *, #10437, .F. ) ;
#17050=VECTOR ( 'NONE', #21520, 1000.000000000000000 ) ;
#17051=CIRCLE ( 'NONE', #5863, 3.606799999999001027 ) ;
#17053=CARTESIAN_POINT ( 'NONE',  ( 144.5560466049839192, -3662.518293485689810, 2245.831027411331434 ) ) ;
#17056=AXIS2_PLACEMENT_3D ( 'NONE', #11190, #18105, #19992 ) ;
#17057=CARTESIAN_POINT ( 'NONE',  ( 14.29440584201453568, -3661.861461941862672, 2249.657208667620580 ) ) ;
#17060=CIRCLE ( 'NONE', #6232, 5.715000000000999947 ) ;
#17061=ORIENTED_EDGE ( 'NONE', *, *, #18385, .F. ) ;
#17062=CARTESIAN_POINT ( 'NONE',  ( 142.7460459831000037, -3581.600847922473804, 2246.630002817673358 ) ) ;
#17067=CYLINDRICAL_SURFACE ( 'NONE', #9088, 2.844799999998998796 ) ;
#17068=ORIENTED_EDGE ( 'NONE', *, *, #11128, .F. ) ;
#17069=VERTEX_POINT ( 'NONE', #8017 ) ;
#17073=VERTEX_POINT ( 'NONE', #2284 ) ;
#17075=VECTOR ( 'NONE', #5086, 1000.000000000000000 ) ;
#17077=CARTESIAN_POINT ( 'NONE',  ( 9.926985991717000246, -3578.860012824000023, 2250.236835079999764 ) ) ;
#17079=CARTESIAN_POINT ( 'NONE',  ( 25.39999999999999858, -3578.860000000000127, 2247.392000000000280 ) ) ;
#17080=CARTESIAN_POINT ( 'NONE',  ( 18.22723190021353545, -3660.957995005359862, 2244.667224069949043 ) ) ;
#17082=DIRECTION ( 'NONE',  ( 0.000000000000000000, 0.000000000000000000, 1.000000000000000000 ) ) ;
#17084=ORIENTED_EDGE ( 'NONE', *, *, #9392, .F. ) ;
#17085=CIRCLE ( 'NONE', #20105, 4.114799999999974034 ) ;
#17086=CARTESIAN_POINT ( 'NONE',  ( 7.276271050567447496, -3657.703743155135726, 2245.923136281652205 ) ) ;
#17090=VERTEX_POINT ( 'NONE', #13401 ) ;
#17093=VERTEX_POINT ( 'NONE', #7898 ) ;
#17095=EDGE_CURVE ( 'NONE', #1923, #9353, #4487, .T. ) ;
#17101=ORIENTED_EDGE ( 'NONE', *, *, #5643, .T. ) ;
#17104=CARTESIAN_POINT ( 'NONE',  ( 127.0000000000000000, -3619.500000000000000, 2239.771999999999935 ) ) ;
#17106=CARTESIAN_POINT ( 'NONE',  ( 142.0458560721536116, -3581.104231592735687, 2249.140446724335561 ) ) ;
#17108=FACE_OUTER_BOUND ( 'NONE', #110, .T. ) ;
#17113=AXIS2_PLACEMENT_3D ( 'NONE', #5145, #98, #23052 ) ;
#17114=CARTESIAN_POINT ( 'NONE',  ( 134.1174645519585908, -3658.281435122416497, 2245.237728517810865 ) ) ;
#17116=EDGE_CURVE ( 'NONE', #12626, #8199, #21805, .T. ) ;
#17117=ORIENTED_EDGE ( 'NONE', *, *, #11212, .T. ) ;
#17118=CARTESIAN_POINT ( 'NONE',  ( 142.0222535324996898, -3661.148760393995417, 2250.052190083144069 ) ) ;
#17119=ORIENTED_EDGE ( 'NONE', *, *, #5212, .F. ) ;
#17127=EDGE_CURVE ( 'NONE', #3088, #18712, #10582, .T. ) ;
#17128=CARTESIAN_POINT ( 'NONE',  ( 12.69999999999999929, -3579.494999999999891, 2246.630000000000109 ) ) ;
#17131=DIRECTION ( 'NONE',  ( 0.000000000000000000, 0.000000000000000000, -1.000000000000000000 ) ) ;
#17133=EDGE_CURVE ( 'NONE', #17093, #10895, #9584, .T. ) ;
#17134=ADVANCED_FACE ( 'NONE', ( #17605 ), #18903, .T. ) ;
#17137=VERTEX_POINT ( 'NONE', #2850 ) ;
#17139=DIRECTION ( 'NONE',  ( 0.000000000000000000, -1.000000000000000000, 0.000000000000000000 ) ) ;
#17140=AXIS2_PLACEMENT_3D ( 'NONE', #1313, #14217, #12104 ) ;
#17142=EDGE_CURVE ( 'NONE', #7229, #13759, #2964, .T. ) ;
#17144=CARTESIAN_POINT ( 'NONE',  ( 137.1599999999999966, -3580.776127254000130, 2255.774000000000342 ) ) ;
#17148=CARTESIAN_POINT ( 'NONE',  ( 4.931849146582301557, -3695.327183876642721, 2260.228917875151637 ) ) ;
#17149=DIRECTION ( 'NONE',  ( 1.000000000000000000, 0.000000000000000000, 0.000000000000000000 ) ) ;
#17151=VERTEX_POINT ( 'NONE', #17254 ) ;
#17152=DIRECTION ( 'NONE',  ( 0.000000000000000000, 0.000000000000000000, 1.000000000000000000 ) ) ;
#17155=ORIENTED_EDGE ( 'NONE', *, *, #17665, .F. ) ;
#17158=CARTESIAN_POINT ( 'NONE',  ( 18.29277998665192939, -3578.277056357326273, 2244.591048105684877 ) ) ;
#17161=EDGE_LOOP ( 'NONE', ( #10376, #2571, #14958, #18757 ) ) ;
#17165=CARTESIAN_POINT ( 'NONE',  ( 151.1299999999999955, -3543.299999999999727, 2240.279999999999745 ) ) ;
#17166=CARTESIAN_POINT ( 'NONE',  ( 10.75008131230051411, -3581.566695960163543, 2248.268778118700538 ) ) ;
#17167=CARTESIAN_POINT ( 'NONE',  ( 101.5999999999999943, -3619.500000000000000, 2239.771999999999935 ) ) ;
#17170=DIRECTION ( 'NONE',  ( 0.000000000000000000, -1.000000000000000000, 0.000000000000000000 ) ) ;
#17171=CARTESIAN_POINT ( 'NONE',  ( 145.2092688553343578, -3661.024727042168252, 2244.688205607526015 ) ) ;
#17172=VERTEX_POINT ( 'NONE', #278 ) ;
#17175=ADVANCED_FACE ( 'NONE', ( #21604 ), #14569, .F. ) ;
#17176=CARTESIAN_POINT ( 'NONE',  ( 13.55331166973191159, -3662.218869883657135, 2249.333995280556792 ) ) ;
#17180=DIRECTION ( 'NONE',  ( -1.000000000000000000, 0.000000000000000000, 0.000000000000000000 ) ) ;
#17181=DIRECTION ( 'NONE',  ( 0.000000000000000000, 0.000000000000000000, -1.000000000000000000 ) ) ;
#17183=DIRECTION ( 'NONE',  ( -1.000000000000000000, 0.000000000000000000, 0.000000000000000000 ) ) ;
#17184=ORIENTED_EDGE ( 'NONE', *, *, #13682, .T. ) ;
#17185=VERTEX_POINT ( 'NONE', #16204 ) ;
#17186=CIRCLE ( 'NONE', #8215, 2.844800000000091700 ) ;
#17190=B_SPLINE_CURVE_WITH_KNOTS ( 'NONE', 3,
 ( #4095, #16402, #7844, #2459, #13115, #20047 ),
 .UNSPECIFIED., .F., .F.,
 ( 4, 1, 1, 4 ),
 ( 0.000000000000000000, 0.3333333333333000081, 0.6666666666667000474, 1.000000000000000000 ),
 .UNSPECIFIED. ) ;
#17194=FACE_OUTER_BOUND ( 'NONE', #10532, .T. ) ;
#17197=DIRECTION ( 'NONE',  ( -5.197384013923999056E-14, 1.000000000000000000, 0.000000000000000000 ) ) ;
#17198=DIRECTION ( 'NONE',  ( 0.000000000000000000, 0.000000000000000000, -1.000000000000000000 ) ) ;
#17199=CARTESIAN_POINT ( 'NONE',  ( 137.3069051741637736, -3577.956663428028151, 2250.089631299345911 ) ) ;
#17200=ORIENTED_EDGE ( 'NONE', *, *, #22684, .T. ) ;
#17201=AXIS2_PLACEMENT_3D ( 'NONE', #3284, #16055, #9142 ) ;
#17202=FACE_OUTER_BOUND ( 'NONE', #20407, .T. ) ;
#17203=ORIENTED_EDGE ( 'NONE', *, *, #133, .F. ) ;
#17206=CARTESIAN_POINT ( 'NONE',  ( 10.57571262906792420, -3657.612833920940830, 2248.698263331576527 ) ) ;
#17208=ORIENTED_EDGE ( 'NONE', *, *, #18278, .T. ) ;
#17209=CARTESIAN_POINT ( 'NONE',  ( 134.1971129226658377, -3581.033299165523658, 2245.555178679493565 ) ) ;
#17210=PRODUCT_DEFINITION_CONTEXT ( 'detailed design', #4108, 'design' ) ;
#17213=DIRECTION ( 'NONE',  ( 0.000000000000000000, 0.000000000000000000, 1.000000000000000000 ) ) ;
#17214=CARTESIAN_POINT ( 'NONE',  ( 95.25000000000000000, -3568.700000000000273, 2247.392000000000280 ) ) ;
#17215=CARTESIAN_POINT ( 'NONE',  ( 142.3245498262872388, -3580.592634219400679, 2249.648323945948505 ) ) ;
#17216=EDGE_LOOP ( 'NONE', ( #4974, #17155, #3103, #533 ) ) ;
#17220=DIRECTION ( 'NONE',  ( 0.000000000000000000, -1.000000000000000000, 0.000000000000000000 ) ) ;
#17222=CARTESIAN_POINT ( 'NONE',  ( 14.61878770176556053, -3581.595291073398130, 2248.174049405876758 ) ) ;
#17224=CARTESIAN_POINT ( 'NONE',  ( 134.0114081857246617, -3658.956231532004949, 2244.804996324768126 ) ) ;
#17226=EDGE_CURVE ( 'NONE', #22243, #12173, #3982, .T. ) ;
#17227=VERTEX_POINT ( 'NONE', #2592 ) ;
#17232=DIRECTION ( 'NONE',  ( -1.000000000000000000, 0.000000000000000000, 0.000000000000000000 ) ) ;
#17235=ORIENTED_EDGE ( 'NONE', *, *, #18673, .T. ) ;
#17236=EDGE_CURVE ( 'NONE', #16534, #21188, #20666, .T. ) ;
#17237=ORIENTED_EDGE ( 'NONE', *, *, #693, .T. ) ;
#17239=CARTESIAN_POINT ( 'NONE',  ( 20.62424768829000143, -3544.570000000000164, 2260.600000000000364 ) ) ;
#17242=VERTEX_POINT ( 'NONE', #13143 ) ;
#17251=DIRECTION ( 'NONE',  ( 0.000000000000000000, -1.000000000000000000, 0.000000000000000000 ) ) ;
#17253=CARTESIAN_POINT ( 'NONE',  ( 142.2400000000000091, -3695.699999999999818, 2255.774000000000342 ) ) ;
#17254=CARTESIAN_POINT ( 'NONE',  ( 151.4000000000000057, -3578.860000000000127, 2244.518167364599321 ) ) ;
#17255=ORIENTED_EDGE ( 'NONE', *, *, #19982, .F. ) ;
#17256=EDGE_LOOP ( 'NONE', ( #19054, #6228, #5835, #21304 ) ) ;
#17257=CARTESIAN_POINT ( 'NONE',  ( 137.0971312009782253, -3543.951823054724173, 2255.616383244340341 ) ) ;
#17258=ADVANCED_FACE ( 'NONE', ( #16882 ), #7638, .T. ) ;
#17259=ORIENTED_EDGE ( 'NONE', *, *, #5959, .T. ) ;
#17260=CIRCLE ( 'NONE', #17635, 2.844800000000001550 ) ;
#17261=CARTESIAN_POINT ( 'NONE',  ( 4.918032642227820439, -3695.360820973939099, 2260.194368632764053 ) ) ;
#17262=AXIS2_PLACEMENT_3D ( 'NONE', #13154, #22506, #22274 ) ;
#17264=EDGE_LOOP ( 'NONE', ( #6821, #13062, #19264, #10160 ) ) ;
#17265=ORIENTED_EDGE ( 'NONE', *, *, #20109, .T. ) ;
#17269=ORIENTED_EDGE ( 'NONE', *, *, #5637, .F. ) ;
#17274=DIRECTION ( 'NONE',  ( 3.547420834900000257E-14, -1.000000000000000000, 0.000000000000000000 ) ) ;
#17277=ORIENTED_EDGE ( 'NONE', *, *, #22247, .F. ) ;
#17280=CARTESIAN_POINT ( 'NONE',  ( 101.5999999999999943, -3568.700000000000273, 2239.771999999999935 ) ) ;
#17284=CARTESIAN_POINT ( 'NONE',  ( 79.80679999999999552, -3670.300000000000182, 2259.837999999999738 ) ) ;
#17285=CARTESIAN_POINT ( 'NONE',  ( 144.8670818688862596, -3661.946559944367436, 2245.194077383999684 ) ) ;
#17287=CARTESIAN_POINT ( 'NONE',  ( 35.56000000000000227, -3568.700000000000273, 2247.392000000000280 ) ) ;
#17288=AXIS2_PLACEMENT_3D ( 'NONE', #17900, #19658, #3599 ) ;
#17289=CARTESIAN_POINT ( 'NONE',  ( 12.57171830751316399, -3662.347666198358638, 2249.186210068741730 ) ) ;
#17294=DIRECTION ( 'NONE',  ( 0.000000000000000000, 0.000000000000000000, -1.000000000000000000 ) ) ;
#17295=CIRCLE ( 'NONE', #820, 1.269999999999882334 ) ;
#17297=AXIS2_PLACEMENT_3D ( 'NONE', #11799, #1369, #17183 ) ;
#17298=CARTESIAN_POINT ( 'NONE',  ( 8.520495716475997128, -3581.600846411636667, 2246.629997383320188 ) ) ;
#17300=CARTESIAN_POINT ( 'NONE',  ( 136.9269649396999853, -3660.140004248000423, 2250.236800000000130 ) ) ;
#17302=FACE_OUTER_BOUND ( 'NONE', #12569, .T. ) ;
#17304=CARTESIAN_POINT ( 'NONE',  ( 9.958091716253592907, -3543.555041880599219, 2255.268543560162470 ) ) ;
#17311=DIRECTION ( 'NONE',  ( 0.000000000000000000, 0.000000000000000000, -1.000000000000000000 ) ) ;
#17313=AXIS2_PLACEMENT_3D ( 'NONE', #9224, #201, #7350 ) ;
#17314=DIRECTION ( 'NONE',  ( 0.000000000000000000, 0.000000000000000000, -1.000000000000000000 ) ) ;
#17315=CARTESIAN_POINT ( 'NONE',  ( 101.5999999999999943, -3670.300000000000182, 2239.009999999999764 ) ) ;
#17318=VERTEX_POINT ( 'NONE', #4463 ) ;
#17320=DIRECTION ( 'NONE',  ( -1.000000000000000000, 0.000000000000000000, 0.000000000000000000 ) ) ;
#17322=CARTESIAN_POINT ( 'NONE',  ( 57.14999999999999858, -3694.430000000000291, 2251.506800000000112 ) ) ;
#17323=CARTESIAN_POINT ( 'NONE',  ( 10.40077585279555450, -3657.828902820233452, 2249.052517041838655 ) ) ;
#17329=DIRECTION ( 'NONE',  ( 0.000000000000000000, 0.000000000000000000, -1.000000000000000000 ) ) ;
#17336=CARTESIAN_POINT ( 'NONE',  ( 15.12912523891256278, -3580.975774486991668, 2249.293871663121990 ) ) ;
#17338=CARTESIAN_POINT ( 'NONE',  ( 134.1931015038649662, -3657.976686104013879, 2245.544188612589551 ) ) ;
#17340=CARTESIAN_POINT ( 'NONE',  ( 15.24000000000000021, -3694.430000000000291, 2255.774000000000342 ) ) ;
#17342=ORIENTED_EDGE ( 'NONE', *, *, #79, .T. ) ;
#17343=FACE_OUTER_BOUND ( 'NONE', #17801, .T. ) ;
#17347=CARTESIAN_POINT ( 'NONE',  ( 135.0886139726999886, -3576.119152860999748, 2246.630000000000109 ) ) ;
#17349=AXIS2_PLACEMENT_3D ( 'NONE', #15831, #2231, #2119 ) ;
#17351=CARTESIAN_POINT ( 'NONE',  ( 15.50959416859028117, -3659.956910932261053, 2250.231754334763082 ) ) ;
#17352=EDGE_CURVE ( 'NONE', #1856, #6511, #15446, .T. ) ;
#17353=CARTESIAN_POINT ( 'NONE',  ( 142.2400000000000091, -3544.570000000000164, 2255.774000000000342 ) ) ;
#17354=AXIS2_PLACEMENT_3D ( 'NONE', #13296, #15291, #4501 ) ;
#17358=EDGE_CURVE ( 'NONE', #20273, #22341, #6469, .T. ) ;
#17362=CARTESIAN_POINT ( 'NONE',  ( 141.8518928781941213, -3657.644192185515294, 2248.757418371342283 ) ) ;
#17363=ORIENTED_EDGE ( 'NONE', *, *, #6651, .T. ) ;
#17367=AXIS2_PLACEMENT_3D ( 'NONE', #7317, #5326, #19853 ) ;
#17369=DIRECTION ( 'NONE',  ( -1.000000000000000000, 0.000000000000000000, 0.000000000000000000 ) ) ;
#17370=ORIENTED_EDGE ( 'NONE', *, *, #969, .T. ) ;
#17371=VERTEX_POINT ( 'NONE', #6702 ) ;
#17372=CARTESIAN_POINT ( 'NONE',  ( 50.79999999999999716, -3670.300000000000182, 2239.009999999999764 ) ) ;
#17375=CARTESIAN_POINT ( 'NONE',  ( 63.50000000000000000, -3644.899999999999636, 2239.009999999999764 ) ) ;
#17376=ADVANCED_FACE ( 'NONE', ( #20627 ), #7225, .T. ) ;
#17378=DIRECTION ( 'NONE',  ( -1.000000000000000000, 0.000000000000000000, 0.000000000000000000 ) ) ;
#17380=CARTESIAN_POINT ( 'NONE',  ( 40.94480000000000075, -3594.099999999999909, 2239.771999999999935 ) ) ;
#17383=EDGE_CURVE ( 'NONE', #5385, #4126, #10202, .T. ) ;
#17386=AXIS2_PLACEMENT_3D ( 'NONE', #15344, #4795, #4553 ) ;
#17387=EDGE_CURVE ( 'NONE', #17090, #16534, #573, .T. ) ;
#17388=ORIENTED_EDGE ( 'NONE', *, *, #7827, .F. ) ;
#17392=CARTESIAN_POINT ( 'NONE',  ( 10.45150839067501813, -3581.237797149968173, 2248.953753074173619 ) ) ;
#17396=EDGE_CURVE ( 'NONE', #19707, #11877, #1985, .T. ) ;
#17397=CIRCLE ( 'NONE', #19661, 3.606800000000000228 ) ;
#17398=CARTESIAN_POINT ( 'NONE',  ( 41.70680000000000121, -3594.099999999999909, 2260.600000000000364 ) ) ;
#17399=CARTESIAN_POINT ( 'NONE',  ( 144.4566314728151895, -3662.673839737894014, 2246.096241040939276 ) ) ;
#17400=CARTESIAN_POINT ( 'NONE',  ( 57.14999999999999858, -3544.570000000000164, 2247.392000000000280 ) ) ;
#17409=CARTESIAN_POINT ( 'NONE',  ( 117.9067999999989951, -3644.899999999999636, 2239.771999999999935 ) ) ;
#17410=DIRECTION ( 'NONE',  ( 0.000000000000000000, 1.000000000000000000, 0.000000000000000000 ) ) ;
#17412=DIRECTION ( 'NONE',  ( -1.000000000000000000, 0.000000000000000000, 0.000000000000000000 ) ) ;
#17414=ORIENTED_EDGE ( 'NONE', *, *, #1529, .T. ) ;
#17415=ADVANCED_FACE ( 'NONE', ( #19000 ), #2940, .T. ) ;
#17418=ORIENTED_EDGE ( 'NONE', *, *, #8578, .T. ) ;
#17420=AXIS2_PLACEMENT_3D ( 'NONE', #11447, #18703, #9798 ) ;
#17422=EDGE_CURVE ( 'NONE', #17069, #17829, #10948, .T. ) ;
#17424=AXIS2_PLACEMENT_3D ( 'NONE', #17375, #12244, #19040 ) ;
#17425=EDGE_CURVE ( 'NONE', #21589, #22478, #13944, .T. ) ;
#17431=CARTESIAN_POINT ( 'NONE',  ( 15.24000000000000021, -3660.786127253999894, 2255.774000000000342 ) ) ;
#17435=EDGE_CURVE ( 'NONE', #18295, #22481, #6844, .T. ) ;
#17436=ORIENTED_EDGE ( 'NONE', *, *, #13438, .F. ) ;
#17440=VECTOR ( 'NONE', #2978, 1000.000000000000000 ) ;
#17442=CARTESIAN_POINT ( 'NONE',  ( 10.85008925745106723, -3657.343667564798579, 2247.916674758225781 ) ) ;
#17446=ORIENTED_EDGE ( 'NONE', *, *, #1635, .T. ) ;
#17450=DIRECTION ( 'NONE',  ( 0.000000000000000000, 0.000000000000000000, -1.000000000000000000 ) ) ;
#17452=CIRCLE ( 'NONE', #16344, 2.844800000000091700 ) ;
#17454=B_SPLINE_CURVE_WITH_KNOTS ( 'NONE', 3,
 ( #3506, #5750, #20038, #17684, #11461, #13005, #688, #16619, #20593, #16845, #458, #9370, #14879, #22011, #20154, #15104, #2559, #6089, #9703, #4433, #18613, #14761, #4091, #16506, #2223, #4203, #22228, #900, #18266, #14988, #8068, #7604, #22347, #7954, #5976, #21901, #13451, #2667, #22122, #15217, #6199 ),
 .UNSPECIFIED., .F., .F.,
 ( 4, 2, 2, 1, 1, 2, 2, 2, 2, 1, 1, 1, 2, 2, 2, 2, 2, 2, 2, 1, 1, 2, 2, 4 ),
 ( 0.000000000000000000, 0.1250000000073855644, 0.1875000000110783605, 0.2187500000129247446, 0.2343750000138479228, 0.2421875000143108858, 0.2500000000147738488, 0.3750000000221110352, 0.4375000000258316701, 0.4687500000276899614, 0.4843750000284952617, 0.4921875000288853941, 0.4960937500290684699, 0.5000000000292516011, 0.5625000000271654921, 0.5937500000262729838, 0.6250000000253805865, 0.6875000000235473863, 0.7187500000224613661, 0.7343750000221259677, 0.7421875000219583240, 0.7460937500217790230, 0.7500000000215996110, 1.000000000000000000 ),
 .UNSPECIFIED. ) ;
#17458=EDGE_CURVE ( 'NONE', #12839, #4608, #16217, .T. ) ;
#17460=CARTESIAN_POINT ( 'NONE',  ( 134.0265221272451015, -3658.817503259591831, 2244.873283007213558 ) ) ;
#17462=CARTESIAN_POINT ( 'NONE',  ( 1.270000000000000018, -3660.140000000000327, 2247.392000000000280 ) ) ;
#17466=CARTESIAN_POINT ( 'NONE',  ( 15.44190828346374467, -3695.444958118781869, 2255.268543560987382 ) ) ;
#17467=CARTESIAN_POINT ( 'NONE',  ( 127.0000000000000000, -3670.300000000000182, 2259.837999999999738 ) ) ;
#17470=CARTESIAN_POINT ( 'NONE',  ( 25.39999999999999858, -3660.140000000000327, 2247.392000000000280 ) ) ;
#17475=CARTESIAN_POINT ( 'NONE',  ( 133.9968099895132525, -3659.875514725911216, 2244.559017653038609 ) ) ;
#17476=EDGE_LOOP ( 'NONE', ( #3330, #18571, #9129, #6933 ) ) ;
#17477=VECTOR ( 'NONE', #3624, 1000.000000000000000 ) ;
#17478=CARTESIAN_POINT ( 'NONE',  ( 151.4000000000000057, -3695.670967364599164, 2239.009999999999764 ) ) ;
#17481=CARTESIAN_POINT ( 'NONE',  ( 38.10000000000000142, -3594.099999999999909, 2239.771999999999935 ) ) ;
#17482=CARTESIAN_POINT ( 'NONE',  ( 139.6999999999999886, -3659.504999999999654, 2246.630000000000109 ) ) ;
#17485=CIRCLE ( 'NONE', #7397, 0.7619999999999987894 ) ;
#17486=DIRECTION ( 'NONE',  ( 0.000000000000000000, 0.000000000000000000, -1.000000000000000000 ) ) ;
#17489=CARTESIAN_POINT ( 'NONE',  ( 18.40091559669128785, -3579.898563401232423, 2244.742832167099550 ) ) ;
#17492=CARTESIAN_POINT ( 'NONE',  ( 141.4948555334656533, -3657.297722024060022, 2247.260386800592642 ) ) ;
#17497=VERTEX_POINT ( 'NONE', #10666 ) ;
#17500=VERTEX_POINT ( 'NONE', #23076 ) ;
#17501=CARTESIAN_POINT ( 'NONE',  ( 4.891147941723409609, -3543.580319133069679, 2260.126839620043938 ) ) ;
#17503=LINE ( 'NONE', #3090, #10273 ) ;
#17508=DIRECTION ( 'NONE',  ( 0.000000000000000000, 0.000000000000000000, 1.000000000000000000 ) ) ;
#17509=DIRECTION ( 'NONE',  ( 0.000000000000000000, 0.000000000000000000, -1.000000000000000000 ) ) ;
#17512=ORIENTED_EDGE ( 'NONE', *, *, #12089, .F. ) ;
#17513=CARTESIAN_POINT ( 'NONE',  ( 88.90000000000000568, -3644.899999999999636, 2261.869999999999891 ) ) ;
#17515=CARTESIAN_POINT ( 'NONE',  ( 10.39560465552007429, -3581.163134149680900, 2249.062244971506061 ) ) ;
#17518=FACE_BOUND ( 'NONE', #2433, .T. ) ;
#17519=EDGE_CURVE ( 'NONE', #2160, #7862, #249, .T. ) ;
#17520=EDGE_CURVE ( 'NONE', #1856, #2862, #22923, .T. ) ;
#17522=CARTESIAN_POINT ( 'NONE',  ( 144.4360977138962312, -3576.295496202077629, 2246.158276164633662 ) ) ;
#17523=DIRECTION ( 'NONE',  ( 0.000000000000000000, 0.000000000000000000, -1.000000000000000000 ) ) ;
#17524=CARTESIAN_POINT ( 'NONE',  ( 10.34485765540272162, -3661.108525532338717, 2250.070618451575683 ) ) ;
#17526=CARTESIAN_POINT ( 'NONE',  ( 147.3450752001671447, -3544.173420539331801, 2260.537168198814925 ) ) ;
#17527=ORIENTED_EDGE ( 'NONE', *, *, #13406, .T. ) ;
#17528=B_SPLINE_CURVE_WITH_KNOTS ( 'NONE', 3,
 ( #1995, #17570, #122, #19343 ),
 .UNSPECIFIED., .F., .F.,
 ( 4, 4 ),
 ( 0.000000000000000000, 1.000000000000000000 ),
 .UNSPECIFIED. ) ;
#17529=AXIS2_PLACEMENT_3D ( 'NONE', #3728, #18033, #19561 ) ;
#17530=FACE_OUTER_BOUND ( 'NONE', #551, .T. ) ;
#17532=CARTESIAN_POINT ( 'NONE',  ( 14.76142536199160560, -3657.543251715168935, 2248.559521133435737 ) ) ;
#17535=ORIENTED_EDGE ( 'NONE', *, *, #16811, .T. ) ;
#17537=ORIENTED_EDGE ( 'NONE', *, *, #10557, .F. ) ;
#17540=EDGE_LOOP ( 'NONE', ( #16182, #157, #5316, #1654 ) ) ;
#17541=CARTESIAN_POINT ( 'NONE',  ( 9.832492551972105588, -3543.382189094968908, 2254.953947932267056 ) ) ;
#17542=CARTESIAN_POINT ( 'NONE',  ( 57.14999999999999858, -3544.570000000000164, 2251.506800000000112 ) ) ;
#17544=LINE ( 'NONE', #5022, #15196 ) ;
#17545=VECTOR ( 'NONE', #1952, 1000.000000000000000 ) ;
#17550=DIRECTION ( 'NONE',  ( 0.000000000000000000, 0.000000000000000000, 1.000000000000000000 ) ) ;
#17551=EDGE_CURVE ( 'NONE', #11149, #8967, #1764, .T. ) ;
#17554=CARTESIAN_POINT ( 'NONE',  ( 6.985000000000000320, -3659.504999999999654, 2246.630000000000109 ) ) ;
#17555=CARTESIAN_POINT ( 'NONE',  ( 130.6067999999989979, -3670.300000000000182, 2260.600000000000364 ) ) ;
#17556=EDGE_CURVE ( 'NONE', #1252, #13105, #2720, .T. ) ;
#17558=ORIENTED_EDGE ( 'NONE', *, *, #17658, .F. ) ;
#17559=CARTESIAN_POINT ( 'NONE',  ( 134.3871257470999865, -3581.600847139000052, 2246.630000000000109 ) ) ;
#17560=CIRCLE ( 'NONE', #10846, 6.477000000001009283 ) ;
#17562=EDGE_LOOP ( 'NONE', ( #13938, #5788, #13227, #14504 ) ) ;
#17567=CARTESIAN_POINT ( 'NONE',  ( 131.8393559128971049, -3695.512751957134697, 2259.997167822851679 ) ) ;
#17570=CARTESIAN_POINT ( 'NONE',  ( 6.985000002048997736, -3579.284482508065139, 2244.570813839142829 ) ) ;
#17571=CARTESIAN_POINT ( 'NONE',  ( 15.47643293920226526, -3580.121238382759202, 2249.943944374062085 ) ) ;
#17573=AXIS2_PLACEMENT_3D ( 'NONE', #12192, #10548, #21223 ) ;
#17574=CARTESIAN_POINT ( 'NONE',  ( 146.1770000000009873, -3579.494999999999891, 2239.009999999999764 ) ) ;
#17578=CARTESIAN_POINT ( 'NONE',  ( 116.8400000000000034, -3568.700000000000273, 2247.392000000000280 ) ) ;
#17581=ORIENTED_EDGE ( 'NONE', *, *, #14655, .F. ) ;
#17585=VERTEX_POINT ( 'NONE', #15944 ) ;
#17587=DIRECTION ( 'NONE',  ( 0.000000000000000000, 0.000000000000000000, 1.000000000000000000 ) ) ;
#17588=CARTESIAN_POINT ( 'NONE',  ( 134.0107419914343154, -3660.047848187909040, 2244.548477525994713 ) ) ;
#17589=CIRCLE ( 'NONE', #11240, 3.606799999999001027 ) ;
#17592=CARTESIAN_POINT ( 'NONE',  ( 124.1552000000010025, -3670.300000000000182, 2259.837999999999738 ) ) ;
#17593=CARTESIAN_POINT ( 'NONE',  ( 60.65520000000000067, -3594.099999999999909, 2261.869999999999891 ) ) ;
#17597=DIRECTION ( 'NONE',  ( 0.000000000000000000, 0.000000000000000000, 1.000000000000000000 ) ) ;
#17601=CARTESIAN_POINT ( 'NONE',  ( 9.698254031360443506, -3695.699999999987995, 2254.617539518482772 ) ) ;
#17602=CARTESIAN_POINT ( 'NONE',  ( 18.34588546172644996, -3580.386202656615751, 2244.987819353370014 ) ) ;
#17604=EDGE_CURVE ( 'NONE', #10320, #6015, #2460, .T. ) ;
#17605=FACE_OUTER_BOUND ( 'NONE', #5854, .T. ) ;
#17606=EDGE_CURVE ( 'NONE', #13352, #6776, #20333, .T. ) ;
#17607=ORIENTED_EDGE ( 'NONE', *, *, #9071, .T. ) ;
#17611=CARTESIAN_POINT ( 'NONE',  ( 116.8400000000000034, -3694.430000000000291, 2243.277199999999993 ) ) ;
#17617=CARTESIAN_POINT ( 'NONE',  ( 4.918047856626605707, -3543.639179025994054, 2260.194362557658224 ) ) ;
#17619=FACE_OUTER_BOUND ( 'NONE', #3148, .T. ) ;
#17620=DIRECTION ( 'NONE',  ( 1.000000000000000000, 0.000000000000000000, 0.000000000000000000 ) ) ;
#17623=PLANE ( 'NONE',  #14457 ) ;
#17624=FACE_BOUND ( 'NONE', #19063, .T. ) ;
#17625=DIRECTION ( 'NONE',  ( 1.000000000000000000, 0.000000000000000000, 0.000000000000000000 ) ) ;
#17626=DIRECTION ( 'NONE',  ( 0.000000000000000000, 0.000000000000000000, 1.000000000000000000 ) ) ;
#17631=CARTESIAN_POINT ( 'NONE',  ( 10.32891780134183612, -3581.066905197333199, 2249.187322304957434 ) ) ;
#17632=DIRECTION ( 'NONE',  ( 0.000000000000000000, 1.000000000000000000, -1.224646799147353207E-16 ) ) ;
#17634=B_SPLINE_CURVE_WITH_KNOTS ( 'NONE', 3,
 ( #3884, #11033, #601, #18181, #7517, #14671, #21815, #9621, #816, #13133, #20620, #4688, #13475, #1053, #4570, #22373, #1161, #2812, #20288, #713, #13366, #15016, #11714, #13244, #20740, #16985, #15128, #7867, #6459, #18638, #4348, #6346, #4233, #9958, #22487, #6234, #18866, #11594, #22257, #17106, #2584, #13600, #934, #20398, #18523, #22035, #7983, #16767, #11839, #5998, #2934, #8208, #9731, #2480, #17215, #18990, #2693, #10071, #15355, #14907, #11372, #16873, #22145, #18746, #6118, #20508, #11487 ),
 .UNSPECIFIED., .F., .F.,
 ( 4, 2, 2, 2, 2, 2, 1, 1, 2, 2, 2, 2, 1, 1, 1, 2, 2, 2, 2, 1, 2, 2, 2, 2, 1, 1, 2, 2, 2, 2, 1, 2, 2, 2, 1, 1, 2, 2, 4 ),
 ( 0.000000000000000000, 0.06250000000155657431, 0.09375000000233692232, 0.1250000000031172565, 0.2500000000069327877, 0.3125000000086731733, 0.3437500000095414232, 0.3593750000100068842, 0.3671875000102372555, 0.3750000000104676823, 0.4375000000137948541, 0.4687500000154145030, 0.4843750000161757274, 0.4921875000165590319, 0.4960937500167533765, 0.4980468750169005920, 0.5000000000170478076, 0.5312500000163082881, 0.5468750000158427715, 0.5546875000155574442, 0.5585937500154427582, 0.5625000000153280721, 0.5937500000142669210, 0.6093750000137334588, 0.6171875000135523814, 0.6210937500136807232, 0.6230468750136081146, 0.6250000000135353950, 0.6875000000106663567, 0.7187500000092291730, 0.7343750000084173779, 0.7421875000081177287, 0.7500000000078179685, 0.8125000000061641803, 0.8437500000053371751, 0.8593750000049256155, 0.8671875000047818416, 0.8750000000046379567, 1.000000000000000000 ),
 .UNSPECIFIED. ) ;
#17635=AXIS2_PLACEMENT_3D ( 'NONE', #4985, #15534, #1581 ) ;
#17639=CARTESIAN_POINT ( 'NONE',  ( 145.0383630478528403, -3577.416324816570523, 2244.919872096889776 ) ) ;
#17641=CARTESIAN_POINT ( 'NONE',  ( 11.81573155947770992, -3662.209820030859191, 2249.343846417981240 ) ) ;
#17642=CARTESIAN_POINT ( 'NONE',  ( 12.69999999999999929, -3659.504999999999654, 2239.771999999999935 ) ) ;
#17643=ORIENTED_EDGE ( 'NONE', *, *, #8936, .F. ) ;
#17644=CARTESIAN_POINT ( 'NONE',  ( 63.50000000000000000, -3644.899999999999636, 2259.837999999999738 ) ) ;
#17645=FACE_OUTER_BOUND ( 'NONE', #9725, .T. ) ;
#17648=CARTESIAN_POINT ( 'NONE',  ( 14.61004568054142005, -3657.396752578035830, 2248.145630951006297 ) ) ;
#17649=CARTESIAN_POINT ( 'NONE',  ( 22.55520000000100111, -3619.500000000000000, 2261.869999999999891 ) ) ;
#17652=AXIS2_PLACEMENT_3D ( 'NONE', #9616, #20283, #16762 ) ;
#17658=EDGE_CURVE ( 'NONE', #14926, #14558, #8422, .T. ) ;
#17660=CARTESIAN_POINT ( 'NONE',  ( 25.39999999999999858, -3568.700000000000273, 2260.600000000000364 ) ) ;
#17662=AXIS2_PLACEMENT_3D ( 'NONE', #5692, #7332, #16452 ) ;
#17663=CARTESIAN_POINT ( 'NONE',  ( 127.0000000000000000, -3670.300000000000182, 2260.600000000000364 ) ) ;
#17665=EDGE_CURVE ( 'NONE', #14593, #16647, #16576, .T. ) ;
#17666=VECTOR ( 'NONE', #7755, 1000.000000000000000 ) ;
#17667=CARTESIAN_POINT ( 'NONE',  ( 139.6999999999999886, -3659.504999999999654, 2246.630000000000109 ) ) ;
#17668=EDGE_LOOP ( 'NONE', ( #6084, #8602, #11953, #11194 ) ) ;
#17673=ADVANCED_FACE ( 'NONE', ( #14769 ), #6487, .T. ) ;
#17674=DIRECTION ( 'NONE',  ( 1.000000000000000000, 0.000000000000000000, 0.000000000000000000 ) ) ;
#17676=CARTESIAN_POINT ( 'NONE',  ( 114.2999999999999972, -3644.899999999999636, 2239.009999999999764 ) ) ;
#17677=VECTOR ( 'NONE', #15050, 1000.000000000000000 ) ;
#17678=ORIENTED_EDGE ( 'NONE', *, *, #12718, .T. ) ;
#17683=TOROIDAL_SURFACE ( 'NONE', #19202, 3.606799999998999695, 0.7620000000000000107 ) ;
#17684=CARTESIAN_POINT ( 'NONE',  ( 145.4009155966692788, -3579.898563401719002, 2244.742832167291454 ) ) ;
#17685=EDGE_CURVE ( 'NONE', #21948, #13787, #19213, .T. ) ;
#17689=DIRECTION ( 'NONE',  ( 0.000000000000000000, 0.000000000000000000, 1.000000000000000000 ) ) ;
#17692=CARTESIAN_POINT ( 'NONE',  ( 95.25000000000000000, -3568.700000000000273, 2244.547199999999975 ) ) ;
#17693=DIRECTION ( 'NONE',  ( 0.000000000000000000, 0.000000000000000000, -1.000000000000000000 ) ) ;
#17694=LINE ( 'NONE', #22844, #19243 ) ;
#17695=EDGE_LOOP ( 'NONE', ( #11305, #4303, #19089, #16467 ) ) ;
#17696=AXIS2_PLACEMENT_3D ( 'NONE', #2912, #10170, #15223 ) ;
#17697=CARTESIAN_POINT ( 'NONE',  ( 15.54902373130514981, -3695.599092773423763, 2255.000110291663077 ) ) ;
#17698=CARTESIAN_POINT ( 'NONE',  ( 28.24479999999899604, -3568.700000000000273, 2261.869999999999891 ) ) ;
#17700=CARTESIAN_POINT ( 'NONE',  ( 4.909231720582250880, -3695.380630526287405, 2260.172378166327235 ) ) ;
#17705=DIRECTION ( 'NONE',  ( 0.000000000000000000, 0.000000000000000000, -1.000000000000000000 ) ) ;
#17706=CARTESIAN_POINT ( 'NONE',  ( 95.25000000000000000, -3694.430000000000291, 2250.236800000000130 ) ) ;
#17707=ORIENTED_EDGE ( 'NONE', *, *, #19387, .F. ) ;
#17708=CYLINDRICAL_SURFACE ( 'NONE', #3470, 2.844799999998998796 ) ;
#17709=FACE_OUTER_BOUND ( 'NONE', #16291, .T. ) ;
#17711=CARTESIAN_POINT ( 'NONE',  ( 136.8551999999999964, -3579.425093798000034, 2250.181036214999949 ) ) ;
#17712=AXIS2_PLACEMENT_3D ( 'NONE', #13651, #10246, #3531 ) ;
#17715=DIRECTION ( 'NONE',  ( 1.000000000000000000, 0.000000000000000000, 0.000000000000000000 ) ) ;
#17717=DIRECTION ( 'NONE',  ( 0.000000000000000000, -1.000000000000000000, 0.000000000000000000 ) ) ;
#17718=EDGE_CURVE ( 'NONE', #724, #14116, #1605, .T. ) ;
#17719=AXIS2_PLACEMENT_3D ( 'NONE', #8316, #1039, #8664 ) ;
#17720=CARTESIAN_POINT ( 'NONE',  ( 137.1914968215908459, -3658.160756285533807, 2249.438291734014911 ) ) ;
#17721=EDGE_CURVE ( 'NONE', #21259, #6861, #2001, .T. ) ;
#17722=EDGE_CURVE ( 'NONE', #2712, #2680, #10983, .T. ) ;
#17724=CARTESIAN_POINT ( 'NONE',  ( 136.9601134096845385, -3660.284759461715112, 2250.236799783840979 ) ) ;
#17725=VERTEX_POINT ( 'NONE', #22585 ) ;
#17734=DIRECTION ( 'NONE',  ( 1.000000000000000000, 0.000000000000000000, 0.000000000000000000 ) ) ;
#17736=DIRECTION ( 'NONE',  ( 0.000000000000000000, 0.000000000000000000, -1.000000000000000000 ) ) ;
#17737=FACE_OUTER_BOUND ( 'NONE', #22724, .T. ) ;
#17739=ORIENTED_EDGE ( 'NONE', *, *, #6312, .T. ) ;
#17742=DIRECTION ( 'NONE',  ( 1.000000000000000000, 0.000000000000000000, 0.000000000000000000 ) ) ;
#17744=CARTESIAN_POINT ( 'NONE',  ( 50.79999999999999716, -3619.500000000000000, 2239.771999999999935 ) ) ;
#17747=ORIENTED_EDGE ( 'NONE', *, *, #9579, .T. ) ;
#17751=DIRECTION ( 'NONE',  ( 0.000000000000000000, 0.000000000000000000, 1.000000000000000000 ) ) ;
#17753=ORIENTED_EDGE ( 'NONE', *, *, #6507, .F. ) ;
#17754=FACE_OUTER_BOUND ( 'NONE', #8294, .T. ) ;
#17755=CIRCLE ( 'NONE', #1660, 2.844800000000091700 ) ;
#17759=CARTESIAN_POINT ( 'NONE',  ( 95.25000000000000000, -3670.300000000000182, 2250.236800000000130 ) ) ;
#17760=FACE_OUTER_BOUND ( 'NONE', #23020, .T. ) ;
#17761=CARTESIAN_POINT ( 'NONE',  ( 22.55520000000100111, -3619.500000000000000, 2259.837999999999738 ) ) ;
#17768=LINE ( 'NONE', #8758, #17545 ) ;
#17769=TOROIDAL_SURFACE ( 'NONE', #17367, 3.606799999999999784, 0.7620000000000000107 ) ;
#17770=CARTESIAN_POINT ( 'NONE',  ( 15.33227593808441469, -3658.426079296531043, 2249.662570456160665 ) ) ;
#17771=CARTESIAN_POINT ( 'NONE',  ( 136.8326572973758744, -3695.618941226884999, 2254.954211613487587 ) ) ;
#17773=CARTESIAN_POINT ( 'NONE',  ( 10.45084209371125183, -3577.751058544115040, 2250.012766604421813 ) ) ;
#17774=ORIENTED_EDGE ( 'NONE', *, *, #9968, .F. ) ;
#17779=DIRECTION ( 'NONE',  ( -1.000000000000000000, 0.000000000000000000, 0.000000000000000000 ) ) ;
#17783=DIRECTION ( 'NONE',  ( 1.000000000000000000, -0.000000000000000000, -0.000000000000000000 ) ) ;
#17786=AXIS2_PLACEMENT_3D ( 'NONE', #726, #15038, #624 ) ;
#17790=DIRECTION ( 'NONE',  ( -1.000000000000000000, 0.000000000000000000, 0.000000000000000000 ) ) ;
#17791=ADVANCED_FACE ( 'NONE', ( #8075 ), #1260, .F. ) ;
#17794=LINE ( 'NONE', #8898, #6558 ) ;
#17795=EDGE_CURVE ( 'NONE', #8900, #13472, #22557, .T. ) ;
#17797=FACE_OUTER_BOUND ( 'NONE', #20606, .T. ) ;
#17799=CIRCLE ( 'NONE', #2819, 1.270000000000000018 ) ;
#17800=AXIS2_PLACEMENT_3D ( 'NONE', #18254, #21664, #21997 ) ;
#17801=EDGE_LOOP ( 'NONE', ( #12851, #3497 ) ) ;
#17802=ORIENTED_EDGE ( 'NONE', *, *, #2364, .T. ) ;
#17803=AXIS2_PLACEMENT_3D ( 'NONE', #7958, #16746, #4325 ) ;
#17804=CARTESIAN_POINT ( 'NONE',  ( 136.9377862181021897, -3580.181062415173074, 2249.913373991909793 ) ) ;
#17806=CARTESIAN_POINT ( 'NONE',  ( 116.8400000000000034, -3695.699999999999818, 2247.392000000000280 ) ) ;
#17809=DIRECTION ( 'NONE',  ( 0.000000000000000000, 0.000000000000000000, 1.000000000000000000 ) ) ;
#17810=LINE ( 'NONE', #17692, #16026 ) ;
#17813=B_SPLINE_CURVE_WITH_KNOTS ( 'NONE', 3,
 ( #19469, #1777, #3411, #14204, #21350, #16068 ),
 .UNSPECIFIED., .F., .F.,
 ( 4, 1, 1, 4 ),
 ( 0.000000000000000000, 0.3333333333333000081, 0.6666666666667000474, 1.000000000000000000 ),
 .UNSPECIFIED. ) ;
#17814=CIRCLE ( 'NONE', #7719, 3.606799999998994366 ) ;
#17816=ORIENTED_EDGE ( 'NONE', *, *, #3765, .F. ) ;
#17818=DIRECTION ( 'NONE',  ( 1.000000000000000000, 0.000000000000000000, 0.000000000000000000 ) ) ;
#17820=EDGE_CURVE ( 'NONE', #7575, #16167, #8728, .T. ) ;
#17822=ORIENTED_EDGE ( 'NONE', *, *, #18398, .T. ) ;
#17823=DIRECTION ( 'NONE',  ( 1.000000000000000000, 0.000000000000000000, 0.000000000000000000 ) ) ;
#17826=ADVANCED_FACE ( 'NONE', ( #3024 ), #1143, .F. ) ;
#17828=CIRCLE ( 'NONE', #1361, 0.7619999999999294005 ) ;
#17829=VERTEX_POINT ( 'NONE', #6680 ) ;
#17833=CARTESIAN_POINT ( 'NONE',  ( 47.95519999999999783, -3619.500000000000000, 2259.837999999999738 ) ) ;
#17836=EDGE_CURVE ( 'NONE', #13352, #21090, #2375, .T. ) ;
#17838=CARTESIAN_POINT ( 'NONE',  ( 25.39999999999999858, -3578.860000000000127, 2247.392000000000280 ) ) ;
#17840=CIRCLE ( 'NONE', #16712, 3.606800000000000228 ) ;
#17844=CYLINDRICAL_SURFACE ( 'NONE', #13402, 2.844799999998998796 ) ;
#17846=AXIS2_PLACEMENT_3D ( 'NONE', #18501, #16850, #18271 ) ;
#17847=CARTESIAN_POINT ( 'NONE',  ( 137.2921315476570499, -3657.990157942962924, 2249.255081503176370 ) ) ;
#17850=ORIENTED_EDGE ( 'NONE', *, *, #3359, .T. ) ;
#17851=VERTEX_POINT ( 'NONE', #22353 ) ;
#17853=CARTESIAN_POINT ( 'NONE',  ( 145.4149999999999920, -3659.504999999999654, 2246.630000000000109 ) ) ;
#17855=ORIENTED_EDGE ( 'NONE', *, *, #8889, .T. ) ;
#17856=CARTESIAN_POINT ( 'NONE',  ( 5.080000000000000071, -3544.570000000000164, 2260.600000000000364 ) ) ;
#17858=FACE_OUTER_BOUND ( 'NONE', #12158, .T. ) ;
#17859=CARTESIAN_POINT ( 'NONE',  ( 9.855200000000998273, -3659.504999999999654, 2256.063560000000052 ) ) ;
#17861=ORIENTED_EDGE ( 'NONE', *, *, #22098, .T. ) ;
#17862=AXIS2_PLACEMENT_3D ( 'NONE', #11216, #16379, #7473 ) ;
#17863=EDGE_CURVE ( 'NONE', #16691, #3271, #149, .T. ) ;
#17864=CARTESIAN_POINT ( 'NONE',  ( 57.14999999999969305, -3670.300000000000182, 2244.547199999999975 ) ) ;
#17865=VERTEX_POINT ( 'NONE', #8190 ) ;
#17866=CIRCLE ( 'NONE', #1395, 1.269999999999882334 ) ;
#17871=CARTESIAN_POINT ( 'NONE',  ( 131.8392664897742179, -3543.487248044008538, 2259.997203529242142 ) ) ;
#17874=VERTEX_POINT ( 'NONE', #15336 ) ;
#17875=CYLINDRICAL_SURFACE ( 'NONE', #9699, 2.844800000000091700 ) ;
#17876=ORIENTED_EDGE ( 'NONE', *, *, #23160, .T. ) ;
#17878=FACE_BOUND ( 'NONE', #12804, .T. ) ;
#17879=AXIS2_PLACEMENT_3D ( 'NONE', #10781, #12770, #9 ) ;
#17881=DIRECTION ( 'NONE',  ( 1.000000000000000000, 0.000000000000000000, 0.000000000000000000 ) ) ;
#17883=DIRECTION ( 'NONE',  ( 0.000000000000000000, 0.000000000000000000, -1.000000000000000000 ) ) ;
#17885=CARTESIAN_POINT ( 'NONE',  ( 18.23925622610050823, -3658.098689426352394, 2245.410334305951437 ) ) ;
#17889=AXIS2_PLACEMENT_3D ( 'NONE', #11517, #965, #2723 ) ;
#17890=EDGE_CURVE ( 'NONE', #10620, #5839, #12402, .T. ) ;
#17892=CARTESIAN_POINT ( 'NONE',  ( 14.63011727138534646, -3657.415010725946104, 2248.209217256212014 ) ) ;
#17893=LINE ( 'NONE', #17649, #18427 ) ;
#17894=EDGE_LOOP ( 'NONE', ( #22406, #738, #3554, #21888 ) ) ;
#17895=DIRECTION ( 'NONE',  ( -1.000000000000000000, 0.000000000000000000, 0.000000000000000000 ) ) ;
#17896=ORIENTED_EDGE ( 'NONE', *, *, #11212, .F. ) ;
#17897=DIRECTION ( 'NONE',  ( 1.000000000000000000, 0.000000000000000000, 0.000000000000000000 ) ) ;
#17900=CARTESIAN_POINT ( 'NONE',  ( 0.000000000000000000, -3694.430000000000291, 2259.329999999999927 ) ) ;
#17901=DIRECTION ( 'NONE',  ( -1.224646799147353207E-16, 1.000000000000000000, 0.000000000000000000 ) ) ;
#17902=DIRECTION ( 'NONE',  ( 1.224646799147353207E-16, 1.000000000000000000, -0.000000000000000000 ) ) ;
#17904=CARTESIAN_POINT ( 'NONE',  ( 15.74707948048999917, -3543.299999999999727, 2254.503999999999905 ) ) ;
#17907=ORIENTED_EDGE ( 'NONE', *, *, #21537, .T. ) ;
#17910=EDGE_LOOP ( 'NONE', ( #6856, #11635, #1480, #15030 ) ) ;
#17911=CYLINDRICAL_SURFACE ( 'NONE', #22252, 2.844799999998998796 ) ;
#17913=DIRECTION ( 'NONE',  ( 0.000000000000000000, 0.000000000000000000, -1.000000000000000000 ) ) ;
#17916=CARTESIAN_POINT ( 'NONE',  ( 137.0191252110892322, -3580.447152269891376, 2249.753138802207559 ) ) ;
#17918=DIRECTION ( 'NONE',  ( 0.000000000000000000, 0.000000000000000000, -1.000000000000000000 ) ) ;
#17920=CARTESIAN_POINT ( 'NONE',  ( 117.1447999999989946, -3594.099999999999909, 2261.869999999999891 ) ) ;
#17922=CARTESIAN_POINT ( 'NONE',  ( 10.16000000000000014, -3580.776127254000130, 2255.774000000000342 ) ) ;
#17924=CARTESIAN_POINT ( 'NONE',  ( 140.7110437557817590, -3576.835571923886619, 2249.390760484202474 ) ) ;
#17925=EDGE_LOOP ( 'NONE', ( #7031, #14691, #17527, #161 ) ) ;
#17926=CARTESIAN_POINT ( 'NONE',  ( 5.080000000000000071, -3544.570000000000164, 2260.600000000000364 ) ) ;
#17927=AXIS2_PLACEMENT_3D ( 'NONE', #7102, #6993, #8970 ) ;
#17928=ORIENTED_EDGE ( 'NONE', *, *, #18110, .F. ) ;
#17930=EDGE_LOOP ( 'NONE', ( #12603, #16935, #23004, #6134 ) ) ;
#17931=CARTESIAN_POINT ( 'NONE',  ( 4.771243568379631483, -3695.598810868119926, 2259.826779105117112 ) ) ;
#17932=AXIS2_PLACEMENT_3D ( 'NONE', #16472, #428, #16703 ) ;
#17933=LINE ( 'NONE', #14435, #21848 ) ;
#17935=ORIENTED_EDGE ( 'NONE', *, *, #14142, .F. ) ;
#17938=ORIENTED_EDGE ( 'NONE', *, *, #21642, .F. ) ;
#17944=CYLINDRICAL_SURFACE ( 'NONE', #19735, 2.844800000000001550 ) ;
#17947=TOROIDAL_SURFACE ( 'NONE', #10487, 3.606799999999999784, 0.7620000000000000107 ) ;
#17953=CARTESIAN_POINT ( 'NONE',  ( 18.27191195451976569, -3580.765843483243316, 2245.279837209925972 ) ) ;
#17954=EDGE_CURVE ( 'NONE', #23086, #20690, #10234, .T. ) ;
#17955=CIRCLE ( 'NONE', #20205, 3.606799999999001027 ) ;
#17959=VERTEX_POINT ( 'NONE', #23053 ) ;
#17960=CARTESIAN_POINT ( 'NONE',  ( 137.1966912320340271, -3660.857380486106194, 2250.145240675303285 ) ) ;
#17961=ORIENTED_EDGE ( 'NONE', *, *, #1621, .F. ) ;
#17962=VERTEX_POINT ( 'NONE', #304 ) ;
#17965=ORIENTED_EDGE ( 'NONE', *, *, #22284, .F. ) ;
#17968=ORIENTED_EDGE ( 'NONE', *, *, #15592, .F. ) ;
#17970=CARTESIAN_POINT ( 'NONE',  ( 6.222999999999998977, -3579.494999999999891, 2239.009999999999764 ) ) ;
#17973=FACE_OUTER_BOUND ( 'NONE', #17540, .T. ) ;
#17974=DIRECTION ( 'NONE',  ( 0.000000000000000000, 0.000000000000000000, -1.000000000000000000 ) ) ;
#17981=CARTESIAN_POINT ( 'NONE',  ( 131.9776566397356703, -3543.802992058954260, 2260.344391216158328 ) ) ;
#17984=CIRCLE ( 'NONE', #3754, 0.7619999999999987894 ) ;
#17990=ORIENTED_EDGE ( 'NONE', *, *, #1197, .F. ) ;
#17993=CARTESIAN_POINT ( 'NONE',  ( 144.6787468485286752, -3576.681201580200195, 2245.535362107170840 ) ) ;
#17994=DIRECTION ( 'NONE',  ( 1.000000000000000000, 0.000000000000000000, 0.000000000000000000 ) ) ;
#17999=ORIENTED_EDGE ( 'NONE', *, *, #11984, .T. ) ;
#18000=PLANE ( 'NONE',  #19877 ) ;
#18001=CARTESIAN_POINT ( 'NONE',  ( 76.20000000000000284, -3568.700000000000273, 2259.837999999999738 ) ) ;
#18004=FACE_OUTER_BOUND ( 'NONE', #2281, .T. ) ;
#18005=CARTESIAN_POINT ( 'NONE',  ( 142.5377471795426345, -3543.413280444186512, 2255.028339697483716 ) ) ;
#18010=CARTESIAN_POINT ( 'NONE',  ( 7.808657878250968132, -3576.539255533550659, 2245.746599050030454 ) ) ;
#18011=ORIENTED_EDGE ( 'NONE', *, *, #13275, .T. ) ;
#18018=DIRECTION ( 'NONE',  ( -1.000000000000000000, 0.000000000000000000, -1.344534956949000041E-13 ) ) ;
#18021=EDGE_CURVE ( 'NONE', #17242, #22049, #20689, .T. ) ;
#18027=VERTEX_POINT ( 'NONE', #17380 ) ;
#18028=EDGE_CURVE ( 'NONE', #8967, #16380, #21841, .T. ) ;
#18029=FACE_OUTER_BOUND ( 'NONE', #16330, .T. ) ;
#18030=TOROIDAL_SURFACE ( 'NONE', #21415, 3.606799999998999695, 0.7620000000000000107 ) ;
#18031=CIRCLE ( 'NONE', #17652, 2.844800000000001550 ) ;
#18033=DIRECTION ( 'NONE',  ( 0.000000000000000000, 0.000000000000000000, 1.000000000000000000 ) ) ;
#18035=ADVANCED_FACE ( 'NONE', ( #992 ), #22663, .T. ) ;
#18036=EDGE_LOOP ( 'NONE', ( #9835, #9732, #6248, #18058 ) ) ;
#18038=CARTESIAN_POINT ( 'NONE',  ( 137.3036342121837379, -3581.028288794486343, 2249.234011237613686 ) ) ;
#18039=ORIENTED_EDGE ( 'NONE', *, *, #15512, .T. ) ;
#18042=DIRECTION ( 'NONE',  ( 1.000000000000000000, 0.000000000000000000, 0.000000000000000000 ) ) ;
#18049=CARTESIAN_POINT ( 'NONE',  ( 138.4607614358540388, -3576.933900292242924, 2249.485745238374875 ) ) ;
#18051=CARTESIAN_POINT ( 'NONE',  ( 134.5203320287740496, -3577.080245332521827, 2245.172503490672170 ) ) ;
#18052=DIRECTION ( 'NONE',  ( 0.000000000000000000, 0.000000000000000000, -1.000000000000000000 ) ) ;
#18055=CARTESIAN_POINT ( 'NONE',  ( 0.000000000000000000, -3694.430000000000291, 2259.329999999999927 ) ) ;
#18057=CIRCLE ( 'NONE', #1576, 2.844799999999994444 ) ;
#18058=ORIENTED_EDGE ( 'NONE', *, *, #12964, .T. ) ;
#18062=ORIENTED_EDGE ( 'NONE', *, *, #5347, .T. ) ;
#18063=CIRCLE ( 'NONE', #7964, 0.7619999999999987894 ) ;
#18064=DIRECTION ( 'NONE',  ( -1.000000000000000000, 0.000000000000000000, 0.000000000000000000 ) ) ;
#18067=CARTESIAN_POINT ( 'NONE',  ( 9.652920519510999497, -3543.299999999999727, 2254.503999999999905 ) ) ;
#18071=CARTESIAN_POINT ( 'NONE',  ( 9.802881971985723197, -3695.643849726979624, 2254.879006055995887 ) ) ;
#18075=CARTESIAN_POINT ( 'NONE',  ( 137.8181448509824918, -3657.371504566497606, 2248.046850338492732 ) ) ;
#18076=ORIENTED_EDGE ( 'NONE', *, *, #10302, .F. ) ;
#18079=CARTESIAN_POINT ( 'NONE',  ( 141.4070264929715393, -3661.780831764733193, 2249.715973214696533 ) ) ;
#18081=VERTEX_POINT ( 'NONE', #7177 ) ;
#18083=DIRECTION ( 'NONE',  ( 0.000000000000000000, -1.000000000000000000, 0.000000000000000000 ) ) ;
#18086=ORIENTED_EDGE ( 'NONE', *, *, #14939, .T. ) ;
#18090=EDGE_CURVE ( 'NONE', #10469, #17185, #9131, .T. ) ;
#18091=ORIENTED_EDGE ( 'NONE', *, *, #15138, .T. ) ;
#18093=LINE ( 'NONE', #19394, #7855 ) ;
#18095=VECTOR ( 'NONE', #13948, 1000.000000000000114 ) ;
#18096=DIRECTION ( 'NONE',  ( 0.000000000000000000, 0.000000000000000000, 1.000000000000000000 ) ) ;
#18099=CARTESIAN_POINT ( 'NONE',  ( 131.7715554716681936, -3543.401400258583635, 2259.827586953830632 ) ) ;
#18100=ORIENTED_EDGE ( 'NONE', *, *, #1892, .F. ) ;
#18102=CARTESIAN_POINT ( 'NONE',  ( 7.545491619780686499, -3661.969978295142482, 2245.207967436793297 ) ) ;
#18103=EDGE_LOOP ( 'NONE', ( #22390, #22952, #15002, #5559 ) ) ;
#18104=AXIS2_PLACEMENT_3D ( 'NONE', #3289, #8798, #21229 ) ;
#18105=DIRECTION ( 'NONE',  ( -0.6887494619146010688, 0.000000000000000000, -0.7249994335945012525 ) ) ;
#18107=DIRECTION ( 'NONE',  ( -1.000000000000000000, -0.000000000000000000, -0.000000000000000000 ) ) ;
#18109=FACE_OUTER_BOUND ( 'NONE', #684, .T. ) ;
#18110=EDGE_CURVE ( 'NONE', #11279, #22077, #15413, .T. ) ;
#18111=VERTEX_POINT ( 'NONE', #22775 ) ;
#18114=DIRECTION ( 'NONE',  ( 0.000000000000000000, 0.000000000000000000, -1.000000000000000000 ) ) ;
#18116=CARTESIAN_POINT ( 'NONE',  ( 88.90000000000000568, -3594.099999999999909, 2259.837999999999738 ) ) ;
#18119=CARTESIAN_POINT ( 'NONE',  ( 142.2400000000000091, -3544.570000000000164, 2255.774000000000342 ) ) ;
#18121=AXIS2_PLACEMENT_3D ( 'NONE', #17667, #5026, #23055 ) ;
#18122=CARTESIAN_POINT ( 'NONE',  ( 7.457719349988209068, -3577.219030987115730, 2245.067999188746398 ) ) ;
#18123=ORIENTED_EDGE ( 'NONE', *, *, #9373, .T. ) ;
#18126=DIRECTION ( 'NONE',  ( 0.000000000000000000, 0.000000000000000000, -1.000000000000000000 ) ) ;
#18129=DIRECTION ( 'NONE',  ( 0.000000000000000000, 0.000000000000000000, -1.000000000000000000 ) ) ;
#18130=DIRECTION ( 'NONE',  ( 0.000000000000000000, 1.000000000000000000, 0.000000000000000000 ) ) ;
#18136=VECTOR ( 'NONE', #7452, 1000.000000000000000 ) ;
#18138=VECTOR ( 'NONE', #14001, 1000.000000000000000 ) ;
#18141=ADVANCED_FACE ( 'NONE', ( #2873 ), #15525, .F. ) ;
#18143=CARTESIAN_POINT ( 'NONE',  ( 142.2400000000000091, -3694.430000000000291, 2255.774000000000342 ) ) ;
#18144=CARTESIAN_POINT ( 'NONE',  ( 50.79999999999999716, -3568.700000000000273, 2239.771999999999935 ) ) ;
#18147=EDGE_CURVE ( 'NONE', #8337, #13988, #1620, .T. ) ;
#18148=CARTESIAN_POINT ( 'NONE',  ( 137.5529558738440983, -3581.361364689894344, 2248.747063143178821 ) ) ;
#18149=ORIENTED_EDGE ( 'NONE', *, *, #13090, .T. ) ;
#18151=TOROIDAL_SURFACE ( 'NONE', #15902, 3.606799999998999695, 0.7620000000000000107 ) ;
#18154=DIRECTION ( 'NONE',  ( -1.000000000000000000, 0.000000000000000000, 0.000000000000000000 ) ) ;
#18159=CARTESIAN_POINT ( 'NONE',  ( 141.7805098429321333, -3577.552631540255788, 2249.919755263941170 ) ) ;
#18160=ORIENTED_EDGE ( 'NONE', *, *, #21305, .T. ) ;
#18161=CARTESIAN_POINT ( 'NONE',  ( 134.6795851643913693, -3576.764266229913119, 2245.468189507787883 ) ) ;
#18162=EDGE_CURVE ( 'NONE', #3671, #16761, #2733, .T. ) ;
#18163=EDGE_CURVE ( 'NONE', #11209, #3129, #7612, .T. ) ;
#18164=CARTESIAN_POINT ( 'NONE',  ( 133.2229999999999848, -3659.504999999999654, 2239.009999999999764 ) ) ;
#18171=VECTOR ( 'NONE', #9466, 1000.000000000000114 ) ;
#18174=DIRECTION ( 'NONE',  ( -1.073225997510925892E-13, 0.000000000000000000, -1.000000000000000000 ) ) ;
#18177=CYLINDRICAL_SURFACE ( 'NONE', #7766, 1.269999999999882334 ) ;
#18180=AXIS2_PLACEMENT_3D ( 'NONE', #8239, #6489, #21015 ) ;
#18181=CARTESIAN_POINT ( 'NONE',  ( 141.5378770596536526, -3581.666564005086911, 2246.925237844513958 ) ) ;
#18182=EDGE_LOOP ( 'NONE', ( #10184, #10043, #18366, #14862 ) ) ;
#18186=CYLINDRICAL_SURFACE ( 'NONE', #10932, 2.844800000000091700 ) ;
#18191=CARTESIAN_POINT ( 'NONE',  ( 137.5756652831487656, -3657.612887080431847, 2248.698366170355257 ) ) ;
#18193=EDGE_LOOP ( 'NONE', ( #617, #7399 ) ) ;
#18194=CARTESIAN_POINT ( 'NONE',  ( 141.0596176031389746, -3662.005499788756879, 2249.540428743966004 ) ) ;
#18195=EDGE_CURVE ( 'NONE', #10683, #7794, #5013, .T. ) ;
#18198=ORIENTED_EDGE ( 'NONE', *, *, #18311, .T. ) ;
#18204=LINE ( 'NONE', #14470, #2438 ) ;
#18208=FACE_OUTER_BOUND ( 'NONE', #6946, .T. ) ;
#18209=CARTESIAN_POINT ( 'NONE',  ( 1.270000000000000018, -3694.430000000000291, 2259.329999999999927 ) ) ;
#18216=DIRECTION ( 'NONE',  ( -1.000000000000000000, 0.000000000000000000, 0.000000000000000000 ) ) ;
#18217=DIRECTION ( 'NONE',  ( -1.224646799147353207E-16, 1.000000000000000000, 0.000000000000000000 ) ) ;
#18218=CARTESIAN_POINT ( 'NONE',  ( 12.69999999999999929, -3579.494999999999891, 2255.774000000000342 ) ) ;
#18219=ORIENTED_EDGE ( 'NONE', *, *, #6233, .T. ) ;
#18220=AXIS2_PLACEMENT_3D ( 'NONE', #23103, #21017, #19256 ) ;
#18221=DIRECTION ( 'NONE',  ( 0.000000000000000000, 0.000000000000000000, -1.000000000000000000 ) ) ;
#18228=ORIENTED_EDGE ( 'NONE', *, *, #1417, .F. ) ;
#18229=DIRECTION ( 'NONE',  ( 0.000000000000000000, 0.000000000000000000, 1.000000000000000000 ) ) ;
#18231=CARTESIAN_POINT ( 'NONE',  ( 57.14999999999999858, -3544.570000000000164, 2250.236800000000130 ) ) ;
#18234=FACE_OUTER_BOUND ( 'NONE', #21829, .T. ) ;
#18238=VECTOR ( 'NONE', #18296, 1000.000000000000000 ) ;
#18242=AXIS2_PLACEMENT_3D ( 'NONE', #12401, #8890, #10873 ) ;
#18244=EDGE_CURVE ( 'NONE', #1840, #12928, #16598, .T. ) ;
#18245=DIRECTION ( 'NONE',  ( -1.000000000000000000, 0.000000000000000000, 0.000000000000000000 ) ) ;
#18246=ADVANCED_FACE ( 'NONE', ( #4930 ), #3887, .T. ) ;
#18252=FACE_OUTER_BOUND ( 'NONE', #12648, .T. ) ;
#18253=VECTOR ( 'NONE', #7126, 999.9999999999998863 ) ;
#18254=CARTESIAN_POINT ( 'NONE',  ( 101.5999999999999943, -3619.500000000000000, 2261.869999999999891 ) ) ;
#18256=ADVANCED_FACE ( 'NONE', ( #12427 ), #10611, .T. ) ;
#18258=CIRCLE ( 'NONE', #22001, 2.844800000000091700 ) ;
#18260=CARTESIAN_POINT ( 'NONE',  ( 142.5315320345694090, -3695.579670240429095, 2255.043779575609278 ) ) ;
#18266=CARTESIAN_POINT ( 'NONE',  ( 145.1763627461602653, -3581.130155333931725, 2245.675470994407078 ) ) ;
#18269=CARTESIAN_POINT ( 'NONE',  ( 76.20000000000000284, -3568.700000000000273, 2239.771999999999935 ) ) ;
#18271=DIRECTION ( 'NONE',  ( 1.073225997510925892E-13, 0.000000000000000000, 1.000000000000000000 ) ) ;
#18272=EDGE_CURVE ( 'NONE', #22006, #10186, #16956, .T. ) ;
#18274=CARTESIAN_POINT ( 'NONE',  ( 142.3112457684844685, -3578.363551668762284, 2250.194032828429954 ) ) ;
#18275=B_SPLINE_CURVE_WITH_KNOTS ( 'NONE', 3,
 ( #10111, #13633, #19028, #855, #11878, #8139, #2967, #20541, #17257, #7903, #6622, #20435, #15283, #13514, #9999, #18672, #13405, #8021, #6384, #18785, #20654, #15168, #13760, #4384, #20904, #4839, #11990, #19143, #6271, #3082, #4491 ),
 .UNSPECIFIED., .F., .F.,
 ( 4, 2, 2, 2, 2, 2, 1, 2, 2, 2, 2, 1, 1, 2, 2, 2, 4 ),
 ( 0.000000000000000000, 0.1249999999979858889, 0.1874999999967077724, 0.2499999999954296559, 0.3749999999932559502, 0.4374999999922616900, 0.4687499999917597027, 0.4843749999919371718, 0.4999999999921146410, 0.6249999999960471619, 0.6874999999979408694, 0.7187499999991345812, 0.7343749999999843459, 0.7421875000001566525, 0.7500000000003289591, 0.8750000000001644240, 1.000000000000000000 ),
 .UNSPECIFIED. ) ;
#18277=CARTESIAN_POINT ( 'NONE',  ( 134.2879922902995418, -3577.658673733719752, 2244.812092252487219 ) ) ;
#18278=EDGE_CURVE ( 'NONE', #11706, #14933, #2388, .T. ) ;
#18279=EDGE_CURVE ( 'NONE', #10484, #21098, #17694, .T. ) ;
#18281=CARTESIAN_POINT ( 'NONE',  ( 101.5999999999999943, -3619.500000000000000, 2259.837999999999738 ) ) ;
#18289=ADVANCED_FACE ( 'NONE', ( #10434 ), #12129, .T. ) ;
#18293=CARTESIAN_POINT ( 'NONE',  ( 15.09345051701841456, -3577.955111082732856, 2250.090084402730099 ) ) ;
#18294=PLANE ( 'NONE',  #7942 ) ;
#18295=VERTEX_POINT ( 'NONE', #3866 ) ;
#18296=DIRECTION ( 'NONE',  ( 0.000000000000000000, 1.000000000000000000, 0.000000000000000000 ) ) ;
#18297=EDGE_CURVE ( 'NONE', #7984, #17318, #22346, .T. ) ;
#18299=DIRECTION ( 'NONE',  ( 0.000000000000000000, 0.000000000000000000, -1.000000000000000000 ) ) ;
#18300=CYLINDRICAL_SURFACE ( 'NONE', #9451, 2.844800000000091700 ) ;
#18301=ORIENTED_EDGE ( 'NONE', *, *, #18278, .F. ) ;
#18304=ORIENTED_EDGE ( 'NONE', *, *, #17890, .F. ) ;
#18305=ORIENTED_EDGE ( 'NONE', *, *, #8808, .T. ) ;
#18306=CIRCLE ( 'NONE', #8203, 0.7619999999999294005 ) ;
#18307=CARTESIAN_POINT ( 'NONE',  ( 140.7875140777326237, -3662.134083993774311, 2249.421034100285851 ) ) ;
#18309=ADVANCED_FACE ( 'NONE', ( #22586 ), #5028, .T. ) ;
#18310=ORIENTED_EDGE ( 'NONE', *, *, #1401, .T. ) ;
#18311=EDGE_CURVE ( 'NONE', #13681, #21672, #696, .T. ) ;
#18312=ORIENTED_EDGE ( 'NONE', *, *, #19626, .T. ) ;
#18318=AXIS2_PLACEMENT_3D ( 'NONE', #8041, #20682, #18931 ) ;
#18327=DIRECTION ( 'NONE',  ( 0.000000000000000000, 0.000000000000000000, -1.000000000000000000 ) ) ;
#18330=CARTESIAN_POINT ( 'NONE',  ( 7.860134522445388683, -3662.544182877184085, 2245.871063940706790 ) ) ;
#18335=DIRECTION ( 'NONE',  ( 1.224646799147353207E-16, 1.000000000000000000, -0.000000000000000000 ) ) ;
#18337=CARTESIAN_POINT ( 'NONE',  ( 59.89320000000000022, -3594.099999999999909, 2239.771999999999935 ) ) ;
#18339=CARTESIAN_POINT ( 'NONE',  ( 147.7412001510571997, -3543.315277321059966, 2259.544298694426743 ) ) ;
#18342=CARTESIAN_POINT ( 'NONE',  ( 142.2400000000000091, -3694.430000000000291, 2255.774000000000342 ) ) ;
#18343=B_SPLINE_CURVE_WITH_KNOTS ( 'NONE', 3,
 ( #6891, #11797, #20700, #3243 ),
 .UNSPECIFIED., .F., .F.,
 ( 4, 4 ),
 ( 0.000000000000000000, 1.000000000000000000 ),
 .UNSPECIFIED. ) ;
#18347=DIRECTION ( 'NONE',  ( 0.000000000000000000, 0.000000000000000000, 1.000000000000000000 ) ) ;
#18348=ORIENTED_EDGE ( 'NONE', *, *, #8429, .T. ) ;
#18351=ORIENTED_EDGE ( 'NONE', *, *, #8733, .T. ) ;
#18355=CARTESIAN_POINT ( 'NONE',  ( 151.1299999999999955, -3543.299999999999727, 2240.279999999999745 ) ) ;
#18356=DIRECTION ( 'NONE',  ( 0.000000000000000000, 0.000000000000000000, -1.000000000000000000 ) ) ;
#18357=EDGE_LOOP ( 'NONE', ( #21495, #3337 ) ) ;
#18362=DIRECTION ( 'NONE',  ( 0.000000000000000000, 0.000000000000000000, -1.000000000000000000 ) ) ;
#18366=ORIENTED_EDGE ( 'NONE', *, *, #3222, .T. ) ;
#18370=CYLINDRICAL_SURFACE ( 'NONE', #18549, 1.269999999999882334 ) ;
#18373=CARTESIAN_POINT ( 'NONE',  ( 73.35520000000001062, -3568.700000000000273, 2239.771999999999935 ) ) ;
#18375=EDGE_CURVE ( 'NONE', #15488, #20927, #20721, .T. ) ;
#18385=EDGE_CURVE ( 'NONE', #13823, #15748, #2032, .T. ) ;
#18387=CARTESIAN_POINT ( 'NONE',  ( 17.96576512614983301, -3661.726329895977869, 2245.029840763826087 ) ) ;
#18390=CARTESIAN_POINT ( 'NONE',  ( 139.9692956761142000, -3576.650356814839597, 2249.183748893157372 ) ) ;
#18391=EDGE_LOOP ( 'NONE', ( #20960, #4678, #16072, #6449 ) ) ;
#18394=CARTESIAN_POINT ( 'NONE',  ( 116.8400000000000034, -3695.699999999999818, 2247.392000000000280 ) ) ;
#18395=EDGE_LOOP ( 'NONE', ( #21437, #2208 ) ) ;
#18397=CARTESIAN_POINT ( 'NONE',  ( 15.38817332932362802, -3543.672816122930726, 2255.402926848485095 ) ) ;
#18398=EDGE_CURVE ( 'NONE', #2146, #20703, #3512, .T. ) ;
#18401=EDGE_CURVE ( 'NONE', #9781, #18611, #19613, .T. ) ;
#18403=ADVANCED_FACE ( 'NONE', ( #6790 ), #13618, .T. ) ;
#18404=ORIENTED_EDGE ( 'NONE', *, *, #8012, .F. ) ;
#18407=CARTESIAN_POINT ( 'NONE',  ( 14.61823970408851459, -3577.393621464491389, 2249.830013958978725 ) ) ;
#18408=DIRECTION ( 'NONE',  ( 0.000000000000000000, 1.000000000000000000, 0.000000000000000000 ) ) ;
#18409=ORIENTED_EDGE ( 'NONE', *, *, #23119, .F. ) ;
#18410=AXIS2_PLACEMENT_3D ( 'NONE', #11743, #15629, #13982 ) ;
#18415=FACE_OUTER_BOUND ( 'NONE', #16444, .T. ) ;
#18416=ORIENTED_EDGE ( 'NONE', *, *, #17435, .T. ) ;
#18417=CARTESIAN_POINT ( 'NONE',  ( 20.52303563691415889, -3543.553571235837353, 2260.091479989294839 ) ) ;
#18420=ORIENTED_EDGE ( 'NONE', *, *, #14655, .T. ) ;
#18422=CARTESIAN_POINT ( 'NONE',  ( 140.4994326884994678, -3662.235235933393142, 2249.316303956256888 ) ) ;
#18425=EDGE_LOOP ( 'NONE', ( #2322, #9440, #17363, #13564, #16957 ) ) ;
#18426=AXIS2_PLACEMENT_3D ( 'NONE', #18966, #4239, #15332 ) ;
#18427=VECTOR ( 'NONE', #202, 1000.000000000000000 ) ;
#18428=CARTESIAN_POINT ( 'NONE',  ( 88.90000000000000568, -3644.899999999999636, 2260.600000000000364 ) ) ;
#18429=ORIENTED_EDGE ( 'NONE', *, *, #371, .T. ) ;
#18430=DIRECTION ( 'NONE',  ( 0.000000000000000000, 0.000000000000000000, 1.000000000000000000 ) ) ;
#18433=CARTESIAN_POINT ( 'NONE',  ( 7.117165288956338820, -3658.282806376657391, 2245.236545222771838 ) ) ;
#18434=DIRECTION ( 'NONE',  ( 0.000000000000000000, -1.000000000000000000, 0.000000000000000000 ) ) ;
#18435=CARTESIAN_POINT ( 'NONE',  ( 139.6999999999999886, -3659.504999999999654, 2239.771999999999935 ) ) ;
#18440=EDGE_CURVE ( 'NONE', #12110, #15239, #4270, .T. ) ;
#18441=CARTESIAN_POINT ( 'NONE',  ( 132.3005794017000198, -3694.430000000000291, 2260.390449568000349 ) ) ;
#18442=TOROIDAL_SURFACE ( 'NONE', #7959, 3.606799999999999784, 0.7620000000000000107 ) ;
#18445=CARTESIAN_POINT ( 'NONE',  ( 15.24000000000000021, -3658.223872745999870, 2255.774000000000342 ) ) ;
#18447=ORIENTED_EDGE ( 'NONE', *, *, #8843, .F. ) ;
#18450=EDGE_LOOP ( 'NONE', ( #6895, #18305, #5644, #1913, #13593, #20134, #14808, #16439 ) ) ;
#18451=AXIS2_PLACEMENT_3D ( 'NONE', #17315, #12048, #8307 ) ;
#18452=EDGE_CURVE ( 'NONE', #11171, #18027, #14384, .T. ) ;
#18454=EDGE_CURVE ( 'NONE', #20632, #10769, #5778, .T. ) ;
#18455=CARTESIAN_POINT ( 'NONE',  ( 18.36780534667559550, -3658.772087440082032, 2244.897599096027079 ) ) ;
#18457=DIRECTION ( 'NONE',  ( 0.000000000000000000, 0.000000000000000000, -1.000000000000000000 ) ) ;
#18458=CYLINDRICAL_SURFACE ( 'NONE', #7292, 5.715000000000997282 ) ;
#18459=AXIS2_PLACEMENT_3D ( 'NONE', #18209, #12933, #3914 ) ;
#18462=DIRECTION ( 'NONE',  ( 0.000000000000000000, 0.000000000000000000, 1.000000000000000000 ) ) ;
#18463=CARTESIAN_POINT ( 'NONE',  ( 142.5174422324677153, -3543.437357047561363, 2255.079235783017793 ) ) ;
#18464=LINE ( 'NONE', #16591, #11689 ) ;
#18465=CARTESIAN_POINT ( 'NONE',  ( 7.497499966924064729, -3577.129409902275256, 2245.133902264068638 ) ) ;
#18471=CARTESIAN_POINT ( 'NONE',  ( 9.855390812759999619, -3579.528596999999991, 2250.157115725000040 ) ) ;
#18473=EDGE_LOOP ( 'NONE', ( #9162, #13088 ) ) ;
#18474=CARTESIAN_POINT ( 'NONE',  ( 134.2617953917601028, -3661.301260524150166, 2244.777305218606216 ) ) ;
#18477=DIRECTION ( 'NONE',  ( 1.000000000000000000, 0.000000000000000000, 0.000000000000000000 ) ) ;
#18478=ORIENTED_EDGE ( 'NONE', *, *, #16948, .F. ) ;
#18479=CARTESIAN_POINT ( 'NONE',  ( 15.44120561128188562, -3660.278885126651858, 2250.236802488000194 ) ) ;
#18482=SPHERICAL_SURFACE ( 'NONE', #3147, 1.270000000000000018 ) ;
#18484=DIRECTION ( 'NONE',  ( 0.000000000000000000, 0.000000000000000000, 1.000000000000000000 ) ) ;
#18488=DIRECTION ( 'NONE',  ( -1.000000000000000000, 0.000000000000000000, 0.000000000000000000 ) ) ;
#18491=EDGE_LOOP ( 'NONE', ( #11217, #727, #18825, #21260 ) ) ;
#18498=CARTESIAN_POINT ( 'NONE',  ( 17.60812544259881562, -3662.432924330847982, 2245.707771157191928 ) ) ;
#18499=B_SPLINE_CURVE_WITH_KNOTS ( 'NONE', 3,
 ( #18471, #2425, #8040, #13542, #21987, #2754, #13425, #666, #22094, #4631, #18930, #9458, #549, #1462, #12256, #8621, #10373, #12366, #14015, #1110, #11903, #22671, #15887, #21283, #23018, #8741, #4989, #3106, #19052, #17631, #6645, #15535, #17515, #8272, #21165, #10488, #17392, #15770, #22782, #10254, #5112, #1348, #1583, #12130, #1229, #6524, #10026, #12018, #20806, #6992, #17166, #14135, #22899, #13784, #13660, #5227, #2881, #19287, #20926, #15421, #22554, #3227, #4754, #3336, #6755, #2991 ),
 .UNSPECIFIED., .F., .F.,
 ( 4, 2, 1, 1, 2, 2, 2, 1, 1, 2, 2, 2, 2, 1, 1, 1, 1, 2, 2, 2, 2, 1, 2, 2, 2, 2, 1, 2, 2, 2, 2, 2, 2, 2, 2, 2, 2, 4 ),
 ( 0.000000000000000000, 0.06250000001292387031, 0.09375000001938579852, 0.1093750000227409619, 0.1171875000244185505, 0.1250000000260961253, 0.1875000000388516719, 0.2187500000451599591, 0.2343750000483139639, 0.2421875000498185937, 0.2500000000513232234, 0.3125000000629582497, 0.3437500000687803703, 0.3593750000717660931, 0.3671875000732587879, 0.3710937500739424078, 0.3730468750743454742, 0.3740234375744863615, 0.3750000000746271933, 0.4062500000718055060, 0.4218750000703743175, 0.4296875000695432045, 0.4335937500691276481, 0.4375000000687120916, 0.4687500000660348998, 0.4843750000646543930, 0.4921875000640169029, 0.4960937500635165254, 0.5000000000630161479, 0.5625000000558735280, 0.5937500000522591970, 0.6093750000502783370, 0.6250000000482974771, 0.6875000000403100886, 0.7500000000323225890, 0.8125000000243352005, 0.8750000000163478120, 1.000000000000000000 ),
 .UNSPECIFIED. ) ;
#18500=AXIS2_PLACEMENT_3D ( 'NONE', #22560, #10146, #11908 ) ;
#18501=CARTESIAN_POINT ( 'NONE',  ( 95.25000000000000000, -3568.700000000000273, 2247.392000000000280 ) ) ;
#18502=DIRECTION ( 'NONE',  ( -0.000000000000000000, -0.000000000000000000, 1.000000000000000000 ) ) ;
#18507=DIRECTION ( 'NONE',  ( 0.000000000000000000, 0.000000000000000000, -1.000000000000000000 ) ) ;
#18509=CARTESIAN_POINT ( 'NONE',  ( 136.8551999999999964, -3579.494999999999891, 2256.063560000000052 ) ) ;
#18512=CARTESIAN_POINT ( 'NONE',  ( 15.74707948048999917, -3543.299999999999727, 2254.503999999999905 ) ) ;
#18513=ORIENTED_EDGE ( 'NONE', *, *, #4140, .F. ) ;
#18521=CARTESIAN_POINT ( 'NONE',  ( 14.46426801451776356, -3577.263211980953201, 2249.746456749269782 ) ) ;
#18522=TOROIDAL_SURFACE ( 'NONE', #16645, 6.477000000000000313, 0.7620000000000000107 ) ;
#18523=CARTESIAN_POINT ( 'NONE',  ( 142.0852733101186516, -3581.045180569711192, 2249.213504086232206 ) ) ;
#18525=DIRECTION ( 'NONE',  ( 0.000000000000000000, -1.000000000000000000, 0.000000000000000000 ) ) ;
#18528=CARTESIAN_POINT ( 'NONE',  ( 20.53015567188813861, -3543.540473573110376, 2260.073663966102231 ) ) ;
#18530=ADVANCED_FACE ( 'NONE', ( #19206 ), #19552, .F. ) ;
#18532=TOROIDAL_SURFACE ( 'NONE', #215, 6.477000000000000313, 0.7620000000000000107 ) ;
#18535=CARTESIAN_POINT ( 'NONE',  ( 101.5999999999999943, -3670.300000000000182, 2239.771999999999935 ) ) ;
#18542=CARTESIAN_POINT ( 'NONE',  ( 114.2999999999999972, -3594.099999999999909, 2239.009999999999764 ) ) ;
#18545=CARTESIAN_POINT ( 'NONE',  ( 7.200432652932446054, -3657.950405511532608, 2245.575309129941616 ) ) ;
#18546=PLANE ( 'NONE',  #7471 ) ;
#18549=AXIS2_PLACEMENT_3D ( 'NONE', #1649, #22000, #18484 ) ;
#18554=CIRCLE ( 'NONE', #14822, 2.844800000000001550 ) ;
#18555=CYLINDRICAL_SURFACE ( 'NONE', #16894, 2.844799999999994444 ) ;
#18556=AXIS2_PLACEMENT_3D ( 'NONE', #8862, #15893, #12371 ) ;
#18557=CARTESIAN_POINT ( 'NONE',  ( 127.0000000000000000, -3619.500000000000000, 2239.771999999999935 ) ) ;
#18559=AXIS2_PLACEMENT_3D ( 'NONE', #6116, #13242, #10420 ) ;
#18560=ORIENTED_EDGE ( 'NONE', *, *, #11946, .F. ) ;
#18561=DIRECTION ( 'NONE',  ( 0.000000000000000000, -1.000000000000000000, 0.000000000000000000 ) ) ;
#18563=CIRCLE ( 'NONE', #13334, 2.844799999999994444 ) ;
#18565=ORIENTED_EDGE ( 'NONE', *, *, #19464, .F. ) ;
#18566=DIRECTION ( 'NONE',  ( 1.000000000000000000, 0.000000000000000000, 0.000000000000000000 ) ) ;
#18567=EDGE_CURVE ( 'NONE', #5595, #650, #3144, .T. ) ;
#18568=AXIS2_PLACEMENT_3D ( 'NONE', #22590, #4332, #8194 ) ;
#18569=ADVANCED_FACE ( 'NONE', ( #20021 ), #21428, .T. ) ;
#18570=DIRECTION ( 'NONE',  ( -1.000000000000000000, 0.000000000000000000, 0.000000000000000000 ) ) ;
#18571=ORIENTED_EDGE ( 'NONE', *, *, #1034, .F. ) ;
#18572=ORIENTED_EDGE ( 'NONE', *, *, #1531, .F. ) ;
#18574=CARTESIAN_POINT ( 'NONE',  ( 95.24999999999970157, -3670.300000000000182, 2244.547199999999975 ) ) ;
#18577=TOROIDAL_SURFACE ( 'NONE', #3239, 3.606799999998999695, 0.7620000000000000107 ) ;
#18579=CARTESIAN_POINT ( 'NONE',  ( 142.5447999999993272, -3579.043785370568457, 2256.063560000000962 ) ) ;
#18581=CARTESIAN_POINT ( 'NONE',  ( 20.70551549691483828, -3695.663357297210496, 2259.634152369406365 ) ) ;
#18588=VECTOR ( 'NONE', #3305, 1000.000000000000000 ) ;
#18590=VERTEX_POINT ( 'NONE', #12868 ) ;
#18591=CARTESIAN_POINT ( 'NONE',  ( 134.7212531515910996, -3662.318798419799805, 2245.535362107170840 ) ) ;
#18592=CIRCLE ( 'NONE', #9989, 0.7619999999999294005 ) ;
#18596=CARTESIAN_POINT ( 'NONE',  ( 13.16106602307787732, -3662.312985057125843, 2249.228091833082544 ) ) ;
#18600=DIRECTION ( 'NONE',  ( 1.000000000000000000, 0.000000000000000000, 0.000000000000000000 ) ) ;
#18601=CARTESIAN_POINT ( 'NONE',  ( 38.10000000000000142, -3644.899999999999636, 2259.837999999999738 ) ) ;
#18602=VECTOR ( 'NONE', #15020, 1000.000000000000000 ) ;
#18605=ORIENTED_EDGE ( 'NONE', *, *, #693, .F. ) ;
#18607=VECTOR ( 'NONE', #14517, 1000.000000000000000 ) ;
#18610=CIRCLE ( 'NONE', #14085, 3.606799999999993567 ) ;
#18611=VERTEX_POINT ( 'NONE', #2095 ) ;
#18612=ADVANCED_FACE ( 'NONE', ( #4072 ), #14753, .T. ) ;
#18613=CARTESIAN_POINT ( 'NONE',  ( 145.2625040556375211, -3580.806353043091349, 2245.317242612459722 ) ) ;
#18617=CARTESIAN_POINT ( 'NONE',  ( 18.36256270591483286, -3660.286495684446891, 2244.547215521768521 ) ) ;
#18621=DIRECTION ( 'NONE',  ( 0.000000000000000000, 0.000000000000000000, 1.000000000000000000 ) ) ;
#18625=CARTESIAN_POINT ( 'NONE',  ( 0.000000000000000000, -3660.140000000000327, 2247.392000000000280 ) ) ;
#18630=ORIENTED_EDGE ( 'NONE', *, *, #2351, .T. ) ;
#18636=CARTESIAN_POINT ( 'NONE',  ( 12.43234888807521976, -3576.659528385393969, 2249.195257278045574 ) ) ;
#18638=CARTESIAN_POINT ( 'NONE',  ( 141.8494091026127819, -3581.358993298141741, 2248.752437981420371 ) ) ;
#18646=ORIENTED_EDGE ( 'NONE', *, *, #16559, .F. ) ;
#18648=EDGE_LOOP ( 'NONE', ( #614, #10280, #15129, #11675, #15633, #12989, #21496, #8341 ) ) ;
#18654=EDGE_LOOP ( 'NONE', ( #4043, #8904, #1721, #5181 ) ) ;
#18656=DIRECTION ( 'NONE',  ( 1.097617497454356000E-13, 0.000000000000000000, 1.000000000000000000 ) ) ;
#18658=CARTESIAN_POINT ( 'NONE',  ( 7.015536193038670376, -3658.914394104701387, 2244.824399554300726 ) ) ;
#18659=EDGE_CURVE ( 'NONE', #22036, #15032, #12749, .T. ) ;
#18665=PLANE ( 'NONE',  #15789 ) ;
#18666=LINE ( 'NONE', #4063, #14155 ) ;
#18671=ORIENTED_EDGE ( 'NONE', *, *, #132, .T. ) ;
#18672=CARTESIAN_POINT ( 'NONE',  ( 137.0197613996714381, -3543.693183278374363, 2255.422803182008920 ) ) ;
#18673=EDGE_CURVE ( 'NONE', #8713, #9808, #14028, .T. ) ;
#18674=ORIENTED_EDGE ( 'NONE', *, *, #7737, .F. ) ;
#18681=CARTESIAN_POINT ( 'NONE',  ( 18.37960467573999779, -3578.859731361000286, 2244.547525601999951 ) ) ;
#18683=FACE_OUTER_BOUND ( 'NONE', #17264, .T. ) ;
#18684=DIRECTION ( 'NONE',  ( -1.000000000000000000, 0.000000000000000000, 0.000000000000000000 ) ) ;
#18685=DIRECTION ( 'NONE',  ( 0.000000000000000000, 0.000000000000000000, -1.000000000000000000 ) ) ;
#18689=EDGE_CURVE ( 'NONE', #16281, #15707, #21509, .T. ) ;
#18691=AXIS2_PLACEMENT_3D ( 'NONE', #3862, #19922, #5978 ) ;
#18692=CARTESIAN_POINT ( 'NONE',  ( 127.0000000000000000, -3660.140000000000327, 2247.392000000000280 ) ) ;
#18695=ORIENTED_EDGE ( 'NONE', *, *, #17795, .F. ) ;
#18698=CARTESIAN_POINT ( 'NONE',  ( 53.64479999999999649, -3619.500000000000000, 2239.771999999999935 ) ) ;
#18700=ORIENTED_EDGE ( 'NONE', *, *, #3073, .T. ) ;
#18701=DIRECTION ( 'NONE',  ( 0.000000000000000000, 0.000000000000000000, -1.000000000000000000 ) ) ;
#18702=CARTESIAN_POINT ( 'NONE',  ( 15.09589954392630595, -3661.040808043710513, 2250.091324297367009 ) ) ;
#18703=DIRECTION ( 'NONE',  ( 0.000000000000000000, 0.000000000000000000, -1.000000000000000000 ) ) ;
#18704=EDGE_LOOP ( 'NONE', ( #13382, #12344, #13140, #14583 ) ) ;
#18712=VERTEX_POINT ( 'NONE', #4636 ) ;
#18713=CARTESIAN_POINT ( 'NONE',  ( 5.080000000000000071, -3544.570000000000164, 2260.600000000000364 ) ) ;
#18714=VERTEX_POINT ( 'NONE', #4301 ) ;
#18719=ADVANCED_FACE ( 'NONE', ( #9686 ), #4414, .F. ) ;
#18720=CARTESIAN_POINT ( 'NONE',  ( 17.66446110557347637, -3662.336897614723057, 2245.582878452307796 ) ) ;
#18724=CARTESIAN_POINT ( 'NONE',  ( 4.572920519510000226, -3543.299999999999727, 2259.329999999999927 ) ) ;
#18728=DIRECTION ( 'NONE',  ( -1.000000000000000000, 0.000000000000000000, 0.000000000000000000 ) ) ;
#18729=CARTESIAN_POINT ( 'NONE',  ( 114.2999999999999972, -3594.099999999999909, 2261.869999999999891 ) ) ;
#18730=ORIENTED_EDGE ( 'NONE', *, *, #13869, .F. ) ;
#18732=CARTESIAN_POINT ( 'NONE',  ( 15.44174945842176250, -3543.555041883176273, 2255.268480148888102 ) ) ;
#18733=EDGE_CURVE ( 'NONE', #6015, #825, #905, .T. ) ;
#18734=VERTEX_POINT ( 'NONE', #18698 ) ;
#18735=AXIS2_PLACEMENT_3D ( 'NONE', #14351, #9189, #21615 ) ;
#18737=EDGE_LOOP ( 'NONE', ( #17208, #16465, #5322 ) ) ;
#18742=CARTESIAN_POINT ( 'NONE',  ( 50.79999999999999716, -3619.500000000000000, 2239.771999999999935 ) ) ;
#18743=CARTESIAN_POINT ( 'NONE',  ( 11.08675752506961132, -3577.151045551118386, 2249.666716971718870 ) ) ;
#18746=CARTESIAN_POINT ( 'NONE',  ( 142.4841666229198722, -3580.081058733761438, 2249.961449664135216 ) ) ;
#18747=ORIENTED_EDGE ( 'NONE', *, *, #1892, .T. ) ;
#18752=CARTESIAN_POINT ( 'NONE',  ( 20.67266563390785095, -3543.360310295285217, 2259.716802593130069 ) ) ;
#18753=AXIS2_PLACEMENT_3D ( 'NONE', #17513, #6521, #6643 ) ;
#18757=ORIENTED_EDGE ( 'NONE', *, *, #14688, .F. ) ;
#18761=EDGE_LOOP ( 'NONE', ( #5268, #286 ) ) ;
#18762=CARTESIAN_POINT ( 'NONE',  ( 53.64479999999999649, -3568.700000000000273, 2259.837999999999738 ) ) ;
#18764=EDGE_LOOP ( 'NONE', ( #15036, #21215 ) ) ;
#18766=CARTESIAN_POINT ( 'NONE',  ( 12.69999999999999929, -3659.504999999999654, 2246.630000000000109 ) ) ;
#18770=CARTESIAN_POINT ( 'NONE',  ( 6.985153502415999860, -3659.505556594000154, 2244.618656866000038 ) ) ;
#18772=B_SPLINE_CURVE_WITH_KNOTS ( 'NONE', 3,
 ( #757, #6289, #9778, #15414, #18581, #13420, #20555, #4626, #2874, #7918, #22545, #18923, #10131, #20798, #4748, #11897, #2531, #16924, #19047, #2984, #9675, #658, #6866 ),
 .UNSPECIFIED., .F., .F.,
 ( 4, 2, 2, 1, 1, 2, 2, 2, 2, 1, 2, 2, 4 ),
 ( 0.000000000000000000, 0.1250000000062300443, 0.1875000000093439700, 0.2187500000104950215, 0.2343750000109342535, 0.2421875000111524123, 0.2500000000113705712, 0.3750000000063293260, 0.4375000000038087311, 0.4687500000027571279, 0.4843750000025556779, 0.5000000000023542279, 1.000000000000000000 ),
 .UNSPECIFIED. ) ;
#18776=ORIENTED_EDGE ( 'NONE', *, *, #8936, .T. ) ;
#18785=CARTESIAN_POINT ( 'NONE',  ( 136.9171347365734732, -3543.485052021662341, 2255.165528817252380 ) ) ;
#18788=ORIENTED_EDGE ( 'NONE', *, *, #8594, .T. ) ;
#18791=CARTESIAN_POINT ( 'NONE',  ( 18.41519309054999454, -3659.279547307537541, 2244.670610241967097 ) ) ;
#18794=CARTESIAN_POINT ( 'NONE',  ( 72.59320000000001016, -3670.300000000000182, 2260.600000000000364 ) ) ;
#18796=AXIS2_PLACEMENT_3D ( 'NONE', #2512, #8134, #6033 ) ;
#18798=CARTESIAN_POINT ( 'NONE',  ( 101.5999999999999943, -3619.500000000000000, 2239.009999999999764 ) ) ;
#18799=FACE_OUTER_BOUND ( 'NONE', #13212, .T. ) ;
#18801=CIRCLE ( 'NONE', #6865, 3.606799999999001027 ) ;
#18802=CARTESIAN_POINT ( 'NONE',  ( 116.8400000000000034, -3670.300000000000182, 2244.547199999999975 ) ) ;
#18803=ORIENTED_EDGE ( 'NONE', *, *, #19838, .F. ) ;
#18806=ORIENTED_EDGE ( 'NONE', *, *, #18279, .F. ) ;
#18807=CARTESIAN_POINT ( 'NONE',  ( 145.3093031406643547, -3658.378945273449972, 2245.143073186572110 ) ) ;
#18808=B_SPLINE_CURVE_WITH_KNOTS ( 'NONE', 3,
 ( #19408, #8975, #23025, #17522, #19636, #8865, #16008, #22905, #6998, #5469, #17993, #19765, #17639, #15778, #19522, #3694, #6880 ),
 .UNSPECIFIED., .F., .F.,
 ( 4, 2, 2, 1, 2, 2, 2, 2, 4 ),
 ( 0.000000000000000000, 0.1250000000007305545, 0.1875000000009396095, 0.2187500000009092449, 0.2343750000009681977, 0.2500000000010271228, 0.5000000000006847856, 0.7500000000003423928, 1.000000000000000000 ),
 .UNSPECIFIED. ) ;
#18813=AXIS2_PLACEMENT_3D ( 'NONE', #19204, #1385, #908 ) ;
#18815=EDGE_CURVE ( 'NONE', #13878, #22201, #2886, .T. ) ;
#18816=CARTESIAN_POINT ( 'NONE',  ( 144.7049814936195560, -3662.264031039746897, 2245.499284825724772 ) ) ;
#18819=CARTESIAN_POINT ( 'NONE',  ( 54.40679999999999694, -3568.700000000000273, 2239.771999999999935 ) ) ;
#18820=ADVANCED_FACE ( 'NONE', ( #1117 ), #4645, .T. ) ;
#18821=CARTESIAN_POINT ( 'NONE',  ( 14.40783068962525704, -3661.780600406073518, 2249.716311546600082 ) ) ;
#18822=EDGE_CURVE ( 'NONE', #17874, #16212, #4183, .T. ) ;
#18823=AXIS2_PLACEMENT_3D ( 'NONE', #17470, #20996, #1420 ) ;
#18825=ORIENTED_EDGE ( 'NONE', *, *, #9676, .F. ) ;
#18826=CARTESIAN_POINT ( 'NONE',  ( 76.20000000000000284, -3568.700000000000273, 2239.009999999999764 ) ) ;
#18834=VECTOR ( 'NONE', #9561, 1000.000000000000000 ) ;
#18835=LINE ( 'NONE', #22457, #7212 ) ;
#18838=CARTESIAN_POINT ( 'NONE',  ( 9.652920519510999497, -3543.299999999999727, 2254.503999999999905 ) ) ;
#18840=TOROIDAL_SURFACE ( 'NONE', #6886, 3.606799999998999695, 0.7620000000000000107 ) ;
#18841=FACE_OUTER_BOUND ( 'NONE', #11050, .T. ) ;
#18843=CARTESIAN_POINT ( 'NONE',  ( 17.76256148820106873, -3662.156670368803134, 2245.385473685605120 ) ) ;
#18847=ORIENTED_EDGE ( 'NONE', *, *, #23017, .F. ) ;
#18850=EDGE_CURVE ( 'NONE', #15816, #159, #5044, .T. ) ;
#18853=ORIENTED_EDGE ( 'NONE', *, *, #5725, .T. ) ;
#18855=B_SPLINE_CURVE_WITH_KNOTS ( 'NONE', 3,
 ( #19489, #17724, #1672, #8829, #15977, #23109, #17960, #21714, #9299, #5787, #4128, #4020, #19961, #16549, #3665, #9056, #5669, #158, #16207, #1908, #20082, #7423, #21938, #10816, #9515, #7306, #11046, #386, #14687, #21608, #280, #19842, #2154, #12806, #16434, #21832, #14800, #12921, #5560, #9412, #14460, #12692, #22046, #16660, #11169, #3897, #3775, #18422, #14574, #16327, #18307, #10929, #5904, #11276, #18194, #2263, #7531, #502, #13041, #18079, #7640, #2029, #20190, #2379, #613, #9180, #7768, #14918, #6014, #13146, #17118, #4247, #11500, #11849, #8220, #8115, #10082, #1061 ),
 .UNSPECIFIED., .F., .F.,
 ( 4, 2, 2, 1, 2, 2, 2, 1, 2, 2, 2, 1, 2, 2, 2, 2, 2, 2, 1, 2, 2, 2, 2, 2, 1, 2, 2, 2, 2, 2, 2, 1, 2, 2, 2, 1, 2, 2, 2, 1, 2, 2, 4 ),
 ( 0.000000000000000000, 0.06249999999963576358, 0.09374999999935469674, 0.1093749999993084698, 0.1171874999992827404, 0.1249999999992570110, 0.1562499999990260291, 0.1718749999989712951, 0.1796874999989692134, 0.1874999999989671595, 0.2187499999990615007, 0.2343749999990822341, 0.2421874999990623334, 0.2499999999990424882, 0.2812499999990388244, 0.2968749999990641375, 0.3124999999990893951, 0.3437499999991340260, 0.3593749999991605604, 0.3671874999991988631, 0.3749999999992371658, 0.5000000000001054712, 0.5625000000005331291, 0.5937500000007637224, 0.6093750000008819612, 0.6171875000009465762, 0.6250000000010110801, 0.6562500000011579626, 0.6718750000012543300, 0.6875000000013506973, 0.7187500000014223067, 0.7343750000014820367, 0.7421875000015212276, 0.7500000000015604185, 0.7812500000013671286, 0.7968750000012251311, 0.8046875000011541879, 0.8125000000010832446, 0.8437500000008643086, 0.8593750000007152057, 0.8671875000006794565, 0.8750000000006435963, 1.000000000000000000 ),
 .UNSPECIFIED. ) ;
#18856=CARTESIAN_POINT ( 'NONE',  ( 10.32556948557736831, -3657.938223185949937, 2249.193569921440940 ) ) ;
#18857=EDGE_CURVE ( 'NONE', #12867, #17851, #18870, .T. ) ;
#18860=VERTEX_POINT ( 'NONE', #17398 ) ;
#18866=CARTESIAN_POINT ( 'NONE',  ( 141.9451864939326526, -3581.242051290370000, 2248.947253967675806 ) ) ;
#18870=CIRCLE ( 'NONE', #6921, 2.844800000000001550 ) ;
#18872=AXIS2_PLACEMENT_3D ( 'NONE', #8871, #12147, #3241 ) ;
#18874=CARTESIAN_POINT ( 'NONE',  ( 20.57361267289067186, -3543.469596741131681, 2259.964971591370613 ) ) ;
#18876=CARTESIAN_POINT ( 'NONE',  ( 12.69999999999999929, -3659.504999999999654, 2239.771999999999935 ) ) ;
#18879=CARTESIAN_POINT ( 'NONE',  ( 0.000000000000000000, -3694.430000000000291, 2240.279999999999745 ) ) ;
#18883=AXIS2_PLACEMENT_3D ( 'NONE', #7340, #419, #12953 ) ;
#18885=DIRECTION ( 'NONE',  ( -1.000000000000000000, 0.000000000000000000, 0.000000000000000000 ) ) ;
#18886=CIRCLE ( 'NONE', #19649, 2.844800000000091700 ) ;
#18887=ORIENTED_EDGE ( 'NONE', *, *, #14046, .T. ) ;
#18889=DIRECTION ( 'NONE',  ( -1.000000000000000000, 0.000000000000000000, 0.000000000000000000 ) ) ;
#18890=ORIENTED_EDGE ( 'NONE', *, *, #1403, .F. ) ;
#18893=DIRECTION ( 'NONE',  ( -1.000000000000000000, 0.000000000000000000, 0.000000000000000000 ) ) ;
#18895=DIRECTION ( 'NONE',  ( -1.000000000000000000, 0.000000000000000000, 0.000000000000000000 ) ) ;
#18899=AXIS2_PLACEMENT_3D ( 'NONE', #2497, #18885, #9416 ) ;
#18900=CIRCLE ( 'NONE', #947, 3.606799999998994366 ) ;
#18903=CYLINDRICAL_SURFACE ( 'NONE', #14339, 1.269999999999882334 ) ;
#18905=ORIENTED_EDGE ( 'NONE', *, *, #20842, .F. ) ;
#18906=CARTESIAN_POINT ( 'NONE',  ( 88.90000000000000568, -3594.099999999999909, 2259.837999999999738 ) ) ;
#18907=ORIENTED_EDGE ( 'NONE', *, *, #1830, .T. ) ;
#18908=FACE_OUTER_BOUND ( 'NONE', #19793, .T. ) ;
#18909=CARTESIAN_POINT ( 'NONE',  ( 18.26114034560631438, -3658.187853388129042, 2245.322692878756698 ) ) ;
#18914=CARTESIAN_POINT ( 'NONE',  ( 20.09942059832000183, -3694.430000000000291, 2260.390449568000349 ) ) ;
#18916=LINE ( 'NONE', #655, #15581 ) ;
#18918=VERTEX_POINT ( 'NONE', #4998 ) ;
#18921=DIRECTION ( 'NONE',  ( 0.000000000000000000, 0.000000000000000000, 1.000000000000000000 ) ) ;
#18923=CARTESIAN_POINT ( 'NONE',  ( 20.63606354183824365, -3695.608900718220866, 2259.808339625531517 ) ) ;
#18925=ORIENTED_EDGE ( 'NONE', *, *, #15516, .T. ) ;
#18927=ORIENTED_EDGE ( 'NONE', *, *, #23023, .T. ) ;
#18928=CIRCLE ( 'NONE', #10329, 4.114799999999974034 ) ;
#18930=CARTESIAN_POINT ( 'NONE',  ( 9.956787186801534517, -3580.253871043101753, 2249.873812345001170 ) ) ;
#18931=DIRECTION ( 'NONE',  ( 0.000000000000000000, 0.000000000000000000, -1.000000000000000000 ) ) ;
#18934=CIRCLE ( 'NONE', #6978, 5.715000000000001634 ) ;
#18935=CARTESIAN_POINT ( 'NONE',  ( 38.10000000000000142, -3644.899999999999636, 2260.600000000000364 ) ) ;
#18938=CARTESIAN_POINT ( 'NONE',  ( 145.3645409109730338, -3660.264428733753448, 2244.549527799832958 ) ) ;
#18939=EDGE_LOOP ( 'NONE', ( #11111, #11615, #13870, #4914 ) ) ;
#18941=CARTESIAN_POINT ( 'NONE',  ( 15.24000000000000021, -3578.213872745999652, 2255.774000000000342 ) ) ;
#18943=CARTESIAN_POINT ( 'NONE',  ( 13.58859980245300925, -3662.207521219565933, 2249.346108138774980 ) ) ;
#18945=ORIENTED_EDGE ( 'NONE', *, *, #14986, .F. ) ;
#18947=CARTESIAN_POINT ( 'NONE',  ( 63.50000000000000000, -3594.099999999999909, 2261.869999999999891 ) ) ;
#18951=CARTESIAN_POINT ( 'NONE',  ( 54.40679999999999694, -3619.500000000000000, 2239.009999999999764 ) ) ;
#18952=DIRECTION ( 'NONE',  ( 0.000000000000000000, 0.000000000000000000, -1.000000000000000000 ) ) ;
#18953=ORIENTED_EDGE ( 'NONE', *, *, #15467, .T. ) ;
#18954=ORIENTED_EDGE ( 'NONE', *, *, #11274, .F. ) ;
#18959=EDGE_CURVE ( 'NONE', #3211, #13045, #2417, .T. ) ;
#18962=CARTESIAN_POINT ( 'NONE',  ( 9.850976268665682767, -3543.400907226547588, 2255.000110291591682 ) ) ;
#18966=CARTESIAN_POINT ( 'NONE',  ( 116.8400000000000034, -3568.700000000000273, 2247.392000000000280 ) ) ;
#18967=CARTESIAN_POINT ( 'NONE',  ( 34.49320000000000164, -3594.099999999999909, 2239.771999999999935 ) ) ;
#18976=VECTOR ( 'NONE', #21624, 1000.000000000000000 ) ;
#18979=ADVANCED_FACE ( 'NONE', ( #1237 ), #14766, .T. ) ;
#18981=CARTESIAN_POINT ( 'NONE',  ( 10.54044424447347872, -3657.652706350100743, 2248.773822481034131 ) ) ;
#18983=EDGE_LOOP ( 'NONE', ( #5093, #165 ) ) ;
#18985=CARTESIAN_POINT ( 'NONE',  ( 134.2831716143903691, -3581.316932381290826, 2245.957881525630000 ) ) ;
#18990=CARTESIAN_POINT ( 'NONE',  ( 142.3276510892873148, -3580.585198262936956, 2249.654023945091012 ) ) ;
#18991=VERTEX_POINT ( 'NONE', #15541 ) ;
#18992=DIRECTION ( 'NONE',  ( 0.000000000000000000, 0.000000000000000000, 1.000000000000000000 ) ) ;
#18994=EDGE_CURVE ( 'NONE', #16380, #9946, #10269, .T. ) ;
#18995=AXIS2_PLACEMENT_3D ( 'NONE', #13033, #18525, #20622 ) ;
#18996=DIRECTION ( 'NONE',  ( 0.000000000000000000, 0.000000000000000000, -1.000000000000000000 ) ) ;
#18997=CARTESIAN_POINT ( 'NONE',  ( 14.69151175564311451, -3581.526608352788571, 2248.384429562235255 ) ) ;
#19000=FACE_OUTER_BOUND ( 'NONE', #4342, .T. ) ;
#19003=DIRECTION ( 'NONE',  ( 1.000000000000000000, 0.000000000000000000, 0.000000000000000000 ) ) ;
#19006=DIRECTION ( 'NONE',  ( 0.000000000000000000, 0.000000000000000000, -1.000000000000000000 ) ) ;
#19008=ORIENTED_EDGE ( 'NONE', *, *, #20859, .T. ) ;
#19010=CARTESIAN_POINT ( 'NONE',  ( 25.39999999999999858, -3578.860000000000127, 2247.392000000000280 ) ) ;
#19012=CIRCLE ( 'NONE', #3287, 1.269999999999882334 ) ;
#19013=DIRECTION ( 'NONE',  ( 0.000000000000000000, 0.000000000000000000, 1.000000000000000000 ) ) ;
#19014=DIRECTION ( 'NONE',  ( 0.000000000000000000, 0.000000000000000000, -1.000000000000000000 ) ) ;
#19021=CARTESIAN_POINT ( 'NONE',  ( 63.50000000000000000, -3644.899999999999636, 2260.600000000000364 ) ) ;
#19023=CARTESIAN_POINT ( 'NONE',  ( 141.4940465161450902, -3657.297238990916867, 2247.526929148741146 ) ) ;
#19025=DIRECTION ( 'NONE',  ( -1.000000000000000000, 0.000000000000000000, 0.000000000000000000 ) ) ;
#19028=CARTESIAN_POINT ( 'NONE',  ( 137.1570006975785816, -3544.409801988883373, 2255.766426251236680 ) ) ;
#19029=EDGE_CURVE ( 'NONE', #650, #5595, #541, .T. ) ;
#19031=CARTESIAN_POINT ( 'NONE',  ( 4.618254035022729020, -3695.699999999998909, 2259.443539527655957 ) ) ;
#19036=DIRECTION ( 'NONE',  ( -1.000000000000000000, 0.000000000000000000, 0.000000000000000000 ) ) ;
#19037=LINE ( 'NONE', #13527, #17440 ) ;
#19040=DIRECTION ( 'NONE',  ( 1.000000000000000000, 0.000000000000000000, 0.000000000000000000 ) ) ;
#19047=CARTESIAN_POINT ( 'NONE',  ( 20.52513111806586465, -3695.450320587698570, 2260.086246565152578 ) ) ;
#19052=CARTESIAN_POINT ( 'NONE',  ( 10.31734595597029625, -3581.049170776430856, 2249.208705551349340 ) ) ;
#19054=ORIENTED_EDGE ( 'NONE', *, *, #898, .F. ) ;
#19055=DIRECTION ( 'NONE',  ( 0.000000000000000000, 0.000000000000000000, -1.000000000000000000 ) ) ;
#19056=CIRCLE ( 'NONE', #14944, 3.606799999999993567 ) ;
#19058=CARTESIAN_POINT ( 'NONE',  ( 144.4943168350663143, -3662.615994720476920, 2245.990590281715413 ) ) ;
#19059=VECTOR ( 'NONE', #21644, 1000.000000000000000 ) ;
#19060=DIRECTION ( 'NONE',  ( 0.000000000000000000, 0.000000000000000000, -1.000000000000000000 ) ) ;
#19062=CARTESIAN_POINT ( 'NONE',  ( 147.3506172137967098, -3544.133557168236621, 2260.523297438373447 ) ) ;
#19063=EDGE_LOOP ( 'NONE', ( #15606, #10841 ) ) ;
#19069=ORIENTED_EDGE ( 'NONE', *, *, #1841, .F. ) ;
#19070=AXIS2_PLACEMENT_3D ( 'NONE', #9262, #16400, #11347 ) ;
#19071=DIRECTION ( 'NONE',  ( 0.000000000000000000, 0.000000000000000000, -1.000000000000000000 ) ) ;
#19074=CIRCLE ( 'NONE', #20550, 2.844799999999052531 ) ;
#19088=DIRECTION ( 'NONE',  ( 0.000000000000000000, 0.000000000000000000, -1.000000000000000000 ) ) ;
#19089=ORIENTED_EDGE ( 'NONE', *, *, #133, .T. ) ;
#19093=CARTESIAN_POINT ( 'NONE',  ( 10.05440704136412222, -3658.459147675929671, 2249.687161261317669 ) ) ;
#19094=EDGE_CURVE ( 'NONE', #15095, #4452, #19278, .T. ) ;
#19096=ORIENTED_EDGE ( 'NONE', *, *, #13572, .T. ) ;
#19097=CARTESIAN_POINT ( 'NONE',  ( 133.9977473889447879, -3579.940010871619506, 2244.748233079255897 ) ) ;
#19098=ORIENTED_EDGE ( 'NONE', *, *, #11232, .F. ) ;
#19107=DIRECTION ( 'NONE',  ( 0.7249994335945011414, 0.000000000000000000, 0.6887494619146010688 ) ) ;
#19108=B_SPLINE_CURVE_WITH_KNOTS ( 'NONE', 3,
 ( #6802, #13943, #5036, #3386, #12181, #10537 ),
 .UNSPECIFIED., .F., .F.,
 ( 4, 1, 1, 4 ),
 ( 0.000000000000000000, 0.3333333333333000081, 0.6666666666667000474, 1.000000000000000000 ),
 .UNSPECIFIED. ) ;
#19110=CARTESIAN_POINT ( 'NONE',  ( 14.74624570788535394, -3581.471973361198252, 2248.523728683949685 ) ) ;
#19112=CARTESIAN_POINT ( 'NONE',  ( 38.10000000000000142, -3644.899999999999636, 2239.771999999999935 ) ) ;
#19114=CARTESIAN_POINT ( 'NONE',  ( 15.59751622981730534, -3695.643849727398901, 2254.879165046700564 ) ) ;
#19117=ORIENTED_EDGE ( 'NONE', *, *, #19810, .F. ) ;
#19118=DIRECTION ( 'NONE',  ( -1.000000000000000000, 0.000000000000000000, 0.000000000000000000 ) ) ;
#19122=ORIENTED_EDGE ( 'NONE', *, *, #13239, .T. ) ;
#19123=ORIENTED_EDGE ( 'NONE', *, *, #9392, .T. ) ;
#19125=CARTESIAN_POINT ( 'NONE',  ( 133.9849999999999852, -3659.504999999999654, 2239.771999999999935 ) ) ;
#19128=FACE_BOUND ( 'NONE', #3672, .T. ) ;
#19129=DIRECTION ( 'NONE',  ( 0.000000000000000000, 0.000000000000000000, -1.000000000000000000 ) ) ;
#19133=AXIS2_PLACEMENT_3D ( 'NONE', #7812, #14854, #5950 ) ;
#19137=CARTESIAN_POINT ( 'NONE',  ( 151.4000000000000057, -3578.860000000000127, 2250.265832635400784 ) ) ;
#19140=EDGE_CURVE ( 'NONE', #11962, #22306, #12489, .T. ) ;
#19141=CARTESIAN_POINT ( 'NONE',  ( 141.6348846241527895, -3657.419409829039068, 2248.223748579871426 ) ) ;
#19142=ORIENTED_EDGE ( 'NONE', *, *, #10667, .F. ) ;
#19143=CARTESIAN_POINT ( 'NONE',  ( 136.8057571348549288, -3543.355825686663138, 2254.886068102028275 ) ) ;
#19145=CIRCLE ( 'NONE', #11299, 0.7619999999999294005 ) ;
#19146=CARTESIAN_POINT ( 'NONE',  ( 22.55520000000100111, -3670.300000000000182, 2259.837999999999738 ) ) ;
#19147=AXIS2_PLACEMENT_3D ( 'NONE', #12209, #3178, #22973 ) ;
#19149=ORIENTED_EDGE ( 'NONE', *, *, #21483, .T. ) ;
#19150=ORIENTED_EDGE ( 'NONE', *, *, #7283, .F. ) ;
#19152=DIRECTION ( 'NONE',  ( 0.000000000000000000, 0.000000000000000000, -1.000000000000000000 ) ) ;
#19153=CARTESIAN_POINT ( 'NONE',  ( 72.59320000000001016, -3568.700000000000273, 2260.600000000000364 ) ) ;
#19157=DIRECTION ( 'NONE',  ( 1.000000000000000000, 0.000000000000000000, 0.000000000000000000 ) ) ;
#19160=DIRECTION ( 'NONE',  ( 1.000000000000000000, 0.000000000000000000, 0.000000000000000000 ) ) ;
#19164=ORIENTED_EDGE ( 'NONE', *, *, #21025, .T. ) ;
#19170=CARTESIAN_POINT ( 'NONE',  ( 50.79999999999999716, -3619.500000000000000, 2261.869999999999891 ) ) ;
#19171=ORIENTED_EDGE ( 'NONE', *, *, #3988, .T. ) ;
#19172=EDGE_CURVE ( 'NONE', #3301, #10484, #5433, .T. ) ;
#19173=FACE_OUTER_BOUND ( 'NONE', #12010, .T. ) ;
#19176=CARTESIAN_POINT ( 'NONE',  ( 144.6754166191346940, -3662.317343768547744, 2245.560154884797612 ) ) ;
#19179=CARTESIAN_POINT ( 'NONE',  ( 11.19369693972251412, -3661.918311847638961, 2249.612478909842594 ) ) ;
#19182=CIRCLE ( 'NONE', #99, 2.844799999999994444 ) ;
#19183=CARTESIAN_POINT ( 'NONE',  ( 47.95519999999999783, -3670.300000000000182, 2259.837999999999738 ) ) ;
#19184=AXIS2_PLACEMENT_3D ( 'NONE', #11425, #755, #17625 ) ;
#19185=DIRECTION ( 'NONE',  ( 0.000000000000000000, 0.000000000000000000, -1.000000000000000000 ) ) ;
#19188=CARTESIAN_POINT ( 'NONE',  ( 63.50000000000000000, -3644.899999999999636, 2239.771999999999935 ) ) ;
#19189=CARTESIAN_POINT ( 'NONE',  ( 15.39205606714550711, -3658.584397266909491, 2249.774343474533453 ) ) ;
#19191=EDGE_LOOP ( 'NONE', ( #5958, #20885, #3053, #10125 ) ) ;
#19192=VERTEX_POINT ( 'NONE', #22739 ) ;
#19193=ORIENTED_EDGE ( 'NONE', *, *, #468, .F. ) ;
#19196=AXIS2_PLACEMENT_3D ( 'NONE', #15256, #3049, #13484 ) ;
#19197=DIRECTION ( 'NONE',  ( 0.000000000000000000, 0.000000000000000000, -1.000000000000000000 ) ) ;
#19202=AXIS2_PLACEMENT_3D ( 'NONE', #7916, #2872, #18684 ) ;
#19204=CARTESIAN_POINT ( 'NONE',  ( 35.56000000000000227, -3544.570000000000164, 2247.392000000000280 ) ) ;
#19206=FACE_OUTER_BOUND ( 'NONE', #13149, .T. ) ;
#19212=CARTESIAN_POINT ( 'NONE',  ( 10.73839315088192592, -3657.443723703987416, 2248.304826634740948 ) ) ;
#19213=CIRCLE ( 'NONE', #13958, 0.7619999999999987894 ) ;
#19214=ORIENTED_EDGE ( 'NONE', *, *, #9872, .F. ) ;
#19215=ORIENTED_EDGE ( 'NONE', *, *, #17685, .T. ) ;
#19216=CARTESIAN_POINT ( 'NONE',  ( 134.1499366578294428, -3580.855533714581725, 2245.364243621502283 ) ) ;
#19218=ORIENTED_EDGE ( 'NONE', *, *, #22168, .F. ) ;
#19221=CARTESIAN_POINT ( 'NONE',  ( 20.82707948048999924, -3543.299999999999727, 2259.329999999999927 ) ) ;
#19223=CARTESIAN_POINT ( 'NONE',  ( 15.24000000000000021, -3580.776127254000130, 2255.774000000000342 ) ) ;
#19224=EDGE_LOOP ( 'NONE', ( #4188, #12420, #5125, #19553 ) ) ;
#19225=CARTESIAN_POINT ( 'NONE',  ( 132.0583097651000060, -3694.797466901999996, 2260.545675974999995 ) ) ;
#19227=EDGE_CURVE ( 'NONE', #22764, #3735, #14833, .T. ) ;
#19228=CARTESIAN_POINT ( 'NONE',  ( -0.2667862122801000213, -3694.430000000000291, 2239.290827591999914 ) ) ;
#19229=CARTESIAN_POINT ( 'NONE',  ( 15.21492942528371373, -3580.825415784637698, 2249.449528553973778 ) ) ;
#19230=AXIS2_PLACEMENT_3D ( 'NONE', #4545, #2790, #17082 ) ;
#19231=CARTESIAN_POINT ( 'NONE',  ( 134.0541150472915888, -3658.613793347861701, 2244.987821917966812 ) ) ;
#19233=ORIENTED_EDGE ( 'NONE', *, *, #9137, .T. ) ;
#19234=CARTESIAN_POINT ( 'NONE',  ( 15.55240168165168058, -3695.602652332858270, 2254.991658124059086 ) ) ;
#19237=FACE_OUTER_BOUND ( 'NONE', #15925, .T. ) ;
#19238=CARTESIAN_POINT ( 'NONE',  ( 35.56000000000000227, -3694.430000000000291, 2247.392000000000280 ) ) ;
#19240=ORIENTED_EDGE ( 'NONE', *, *, #3776, .T. ) ;
#19241=CYLINDRICAL_SURFACE ( 'NONE', #2311, 2.844799999998995244 ) ;
#19242=CARTESIAN_POINT ( 'NONE',  ( 134.0191424391260568, -3660.128805427137195, 2244.547198930071318 ) ) ;
#19243=VECTOR ( 'NONE', #21108, 1000.000000000000000 ) ;
#19244=ORIENTED_EDGE ( 'NONE', *, *, #281, .F. ) ;
#19248=CARTESIAN_POINT ( 'NONE',  ( 136.6539306146721913, -3657.399154367426945, 2246.629994581112896 ) ) ;
#19249=CARTESIAN_POINT ( 'NONE',  ( 59.89320000000000022, -3644.899999999999636, 2239.771999999999935 ) ) ;
#19250=AXIS2_PLACEMENT_3D ( 'NONE', #22568, #9801, #6537 ) ;
#19254=CARTESIAN_POINT ( 'NONE',  ( 35.56000000000000227, -3670.300000000000182, 2244.547199999999975 ) ) ;
#19256=DIRECTION ( 'NONE',  ( 0.000000000000000000, 0.000000000000000000, -1.000000000000000000 ) ) ;
#19258=EDGE_CURVE ( 'NONE', #11298, #10072, #2516, .T. ) ;
#19259=CARTESIAN_POINT ( 'NONE',  ( 142.0244369740106833, -3657.864944588135131, 2249.100147049036877 ) ) ;
#19264=ORIENTED_EDGE ( 'NONE', *, *, #3055, .T. ) ;
#19265=TOROIDAL_SURFACE ( 'NONE', #14403, 4.114799999999999791, 1.270000000000000018 ) ;
#19272=LINE ( 'NONE', #19389, #12151 ) ;
#19274=EDGE_LOOP ( 'NONE', ( #22871, #18890, #19743, #2674 ) ) ;
#19278=CIRCLE ( 'NONE', #2786, 2.844799999999994444 ) ;
#19282=AXIS2_PLACEMENT_3D ( 'NONE', #6332, #13707, #2681 ) ;
#19284=CIRCLE ( 'NONE', #13674, 5.715000000000997282 ) ;
#19286=EDGE_CURVE ( 'NONE', #16839, #923, #20879, .T. ) ;
#19287=CARTESIAN_POINT ( 'NONE',  ( 10.87999328488129969, -3581.681618670022090, 2247.764026984493739 ) ) ;
#19295=CARTESIAN_POINT ( 'NONE',  ( 144.8951781795001068, -3661.886301090974939, 2245.146221596522082 ) ) ;
#19300=CARTESIAN_POINT ( 'NONE',  ( 147.3828687998903035, -3543.951823051294468, 2260.442383242537289 ) ) ;
#19301=AXIS2_PLACEMENT_3D ( 'NONE', #6072, #7938, #20473 ) ;
#19303=CARTESIAN_POINT ( 'NONE',  ( 142.2400000000000091, -3580.776127254000130, 2255.774000000000342 ) ) ;
#19306=CARTESIAN_POINT ( 'NONE',  ( 15.07032488946356352, -3657.931869745440963, 2249.185847854341773 ) ) ;
#19313=EDGE_LOOP ( 'NONE', ( #17965, #22388, #15930, #12188 ) ) ;
#19317=CARTESIAN_POINT ( 'NONE',  ( 12.69999999999999929, -3659.504999999999654, 2246.630000000000109 ) ) ;
#19318=CIRCLE ( 'NONE', #17424, 3.606799999999993567 ) ;
#19325=DIRECTION ( 'NONE',  ( 0.000000000000000000, -1.000000000000000000, 0.000000000000000000 ) ) ;
#19326=ORIENTED_EDGE ( 'NONE', *, *, #15595, .T. ) ;
#19330=CARTESIAN_POINT ( 'NONE',  ( 10.19155798493820697, -3658.160642684393679, 2249.438182561015310 ) ) ;
#19334=ADVANCED_FACE ( 'NONE', ( #21344 ), #7305, .T. ) ;
#19337=CARTESIAN_POINT ( 'NONE',  ( 12.69999999999999929, -3579.494999999999891, 2239.771999999999935 ) ) ;
#19339=CARTESIAN_POINT ( 'NONE',  ( 130.6067999999989979, -3568.700000000000273, 2239.771999999999935 ) ) ;
#19343=CARTESIAN_POINT ( 'NONE',  ( 7.020348529275000082, -3578.860230781999689, 2244.548186305999934 ) ) ;
#19346=CARTESIAN_POINT ( 'NONE',  ( 134.2542439495752262, -3657.771239293389954, 2245.816275623240472 ) ) ;
#19348=CARTESIAN_POINT ( 'NONE',  ( 127.0000000000000000, -3568.700000000000273, 2239.771999999999935 ) ) ;
#19349=ORIENTED_EDGE ( 'NONE', *, *, #4140, .T. ) ;
#19353=ORIENTED_EDGE ( 'NONE', *, *, #15293, .F. ) ;
#19354=CARTESIAN_POINT ( 'NONE',  ( 57.14999999999999858, -3694.430000000000291, 2247.392000000000280 ) ) ;
#19358=DIRECTION ( 'NONE',  ( 1.000000000000000000, 0.000000000000000000, 0.000000000000000000 ) ) ;
#19363=DIRECTION ( 'NONE',  ( -1.000000000000000000, 0.000000000000000000, 0.000000000000000000 ) ) ;
#19365=CARTESIAN_POINT ( 'NONE',  ( 15.54478274857000031, -3659.509919104000346, 2250.166342301999521 ) ) ;
#19368=CIRCLE ( 'NONE', #5533, 3.606799999999993567 ) ;
#19369=AXIS2_PLACEMENT_3D ( 'NONE', #8568, #10197, #3046 ) ;
#19372=CARTESIAN_POINT ( 'NONE',  ( 18.37347785155967728, -3580.182493284099110, 2244.873281192540617 ) ) ;
#19373=CARTESIAN_POINT ( 'NONE',  ( 141.5058393440477005, -3657.306719107069966, 2247.135511502391637 ) ) ;
#19374=EDGE_LOOP ( 'NONE', ( #3319, #5438, #19929, #19164 ) ) ;
#19378=EDGE_LOOP ( 'NONE', ( #16629, #10876 ) ) ;
#19386=CARTESIAN_POINT ( 'NONE',  ( 4.771292762646392127, -3543.401189131885076, 2259.826759462805512 ) ) ;
#19387=EDGE_CURVE ( 'NONE', #9415, #10881, #10323, .T. ) ;
#19389=CARTESIAN_POINT ( 'NONE',  ( 15.54479999999999862, -3579.494999999999891, 2272.030000000000200 ) ) ;
#19390=CARTESIAN_POINT ( 'NONE',  ( 47.19319999999999737, -3619.500000000000000, 2259.837999999999738 ) ) ;
#19391=ADVANCED_FACE ( 'NONE', ( #15721 ), #10287, .T. ) ;
#19393=CARTESIAN_POINT ( 'NONE',  ( 136.8551999999999964, -3579.494999999999891, 2256.063560000000052 ) ) ;
#19394=CARTESIAN_POINT ( 'NONE',  ( 10.16000000000000014, -3580.776127254000130, 2255.774000000000342 ) ) ;
#19397=EDGE_LOOP ( 'NONE', ( #6697, #18011, #6215, #5984, #4931, #19233, #10993, #21144 ) ) ;
#19401=DIRECTION ( 'NONE',  ( 0.000000000000000000, -1.000000000000000000, 0.000000000000000000 ) ) ;
#19402=CARTESIAN_POINT ( 'NONE',  ( 25.39999999999999858, -3619.500000000000000, 2259.837999999999738 ) ) ;
#19403=DIRECTION ( 'NONE',  ( -1.000000000000000000, 0.000000000000000000, 0.000000000000000000 ) ) ;
#19408=CARTESIAN_POINT ( 'NONE',  ( 144.3113860273000171, -3576.119152860999748, 2246.630000000000109 ) ) ;
#19410=CARTESIAN_POINT ( 'NONE',  ( 11.26131265196617193, -3661.959416329594205, 2249.579061434116738 ) ) ;
#19411=ORIENTED_EDGE ( 'NONE', *, *, #4541, .F. ) ;
#19414=CARTESIAN_POINT ( 'NONE',  ( 142.4431999999993366, -3580.373257047432162, 2255.967040000000907 ) ) ;
#19416=ADVANCED_FACE ( 'NONE', ( #14315 ), #18151, .T. ) ;
#19420=CARTESIAN_POINT ( 'NONE',  ( 15.33695353576711007, -3658.437581818261151, 2249.671216759049457 ) ) ;
#19421=FACE_OUTER_BOUND ( 'NONE', #8744, .T. ) ;
#19422=EDGE_LOOP ( 'NONE', ( #3262, #11187, #5673, #10349 ) ) ;
#19423=CARTESIAN_POINT ( 'NONE',  ( 10.27280990245528258, -3578.011077221096457, 2250.107236679559264 ) ) ;
#19425=CARTESIAN_POINT ( 'NONE',  ( 88.90000000000000568, -3594.099999999999909, 2259.837999999999738 ) ) ;
#19427=CYLINDRICAL_SURFACE ( 'NONE', #10778, 2.844799999999994444 ) ;
#19429=DIRECTION ( 'NONE',  ( 1.000000000000000000, 0.000000000000000000, 0.000000000000000000 ) ) ;
#19433=AXIS2_PLACEMENT_3D ( 'NONE', #19884, #21528, #7460 ) ;
#19434=DIRECTION ( 'NONE',  ( 0.000000000000000000, 0.000000000000000000, -1.000000000000000000 ) ) ;
#19435=CARTESIAN_POINT ( 'NONE',  ( 17.51847272801180466, -3576.421590885849128, 2245.925646346420308 ) ) ;
#19439=CARTESIAN_POINT ( 'NONE',  ( 6.222999999999998977, -3579.494999999999891, 2239.771999999999935 ) ) ;
#19440=ORIENTED_EDGE ( 'NONE', *, *, #7879, .T. ) ;
#19441=DIRECTION ( 'NONE',  ( -1.000000000000000000, 0.000000000000000000, 0.000000000000000000 ) ) ;
#19442=EDGE_LOOP ( 'NONE', ( #10829, #1351 ) ) ;
#19443=CARTESIAN_POINT ( 'NONE',  ( 134.1618273608623610, -3580.901497745790493, 2245.410526384101104 ) ) ;
#19449=ADVANCED_FACE ( 'NONE', ( #15835 ), #22620, .T. ) ;
#19451=EDGE_CURVE ( 'NONE', #10440, #22481, #15919, .T. ) ;
#19454=CARTESIAN_POINT ( 'NONE',  ( 101.5999999999999943, -3619.500000000000000, 2239.009999999999764 ) ) ;
#19462=ORIENTED_EDGE ( 'NONE', *, *, #7379, .F. ) ;
#19464=EDGE_CURVE ( 'NONE', #830, #20690, #13122, .T. ) ;
#19465=EDGE_CURVE ( 'NONE', #12928, #1840, #11765, .T. ) ;
#19467=ORIENTED_EDGE ( 'NONE', *, *, #22303, .F. ) ;
#19468=CARTESIAN_POINT ( 'NONE',  ( 88.90000000000000568, -3594.099999999999909, 2239.771999999999935 ) ) ;
#19469=CARTESIAN_POINT ( 'NONE',  ( 20.09942059832000183, -3544.570000000000164, 2260.390449568000349 ) ) ;
#19473=AXIS2_PLACEMENT_3D ( 'NONE', #12512, #17901, #12287 ) ;
#19475=CARTESIAN_POINT ( 'NONE',  ( 9.956800000000452400, -3658.626742952519635, 2255.967039999999997 ) ) ;
#19476=EDGE_CURVE ( 'NONE', #15258, #22364, #1671, .T. ) ;
#19477=DIRECTION ( 'NONE',  ( 1.000000000000000000, 0.000000000000000000, 0.000000000000000000 ) ) ;
#19484=CARTESIAN_POINT ( 'NONE',  ( 134.0204252830999962, -3660.140268639000169, 2244.547525601999951 ) ) ;
#19486=DIRECTION ( 'NONE',  ( -1.224646799147353207E-16, 1.000000000000000000, 0.000000000000000000 ) ) ;
#19487=CARTESIAN_POINT ( 'NONE',  ( 137.9049381359793358, -3657.298025595380295, 2247.542742861386614 ) ) ;
#19489=CARTESIAN_POINT ( 'NONE',  ( 136.9269649396999853, -3660.140004248000423, 2250.236800000000130 ) ) ;
#19494=ORIENTED_EDGE ( 'NONE', *, *, #21693, .F. ) ;
#19495=CARTESIAN_POINT ( 'NONE',  ( 47.95519999999999783, -3568.700000000000273, 2261.869999999999891 ) ) ;
#19496=VERTEX_POINT ( 'NONE', #20162 ) ;
#19498=CARTESIAN_POINT ( 'NONE',  ( 4.926372769448470024, -3543.659322604134104, 2260.215249077962198 ) ) ;
#19500=CARTESIAN_POINT ( 'NONE',  ( 117.9067999999989951, -3644.899999999999636, 2239.009999999999764 ) ) ;
#19501=CYLINDRICAL_SURFACE ( 'NONE', #23043, 2.844799999998995244 ) ;
#19502=ORIENTED_EDGE ( 'NONE', *, *, #16299, .T. ) ;
#19504=CARTESIAN_POINT ( 'NONE',  ( 86.05520000000001346, -3594.099999999999909, 2259.837999999999738 ) ) ;
#19508=ORIENTED_EDGE ( 'NONE', *, *, #17026, .T. ) ;
#19511=CARTESIAN_POINT ( 'NONE',  ( 131.8608732113245026, -3543.522855673919821, 2260.051190815687278 ) ) ;
#19513=LINE ( 'NONE', #10609, #17677 ) ;
#19516=ORIENTED_EDGE ( 'NONE', *, *, #115, .T. ) ;
#19517=VECTOR ( 'NONE', #9681, 1000.000000000000000 ) ;
#19518=FACE_BOUND ( 'NONE', #9021, .T. ) ;
#19519=EDGE_CURVE ( 'NONE', #18590, #10446, #15080, .T. ) ;
#19520=CIRCLE ( 'NONE', #21766, 2.844799999999046758 ) ;
#19521=DIRECTION ( 'NONE',  ( 0.000000000000000000, -1.000000000000000000, 0.000000000000000000 ) ) ;
#19522=CARTESIAN_POINT ( 'NONE',  ( 145.2927459769028644, -3578.276998771325452, 2244.591060091298004 ) ) ;
#19523=DIRECTION ( 'NONE',  ( -0.000000000000000000, -1.000000000000000000, -0.000000000000000000 ) ) ;
#19524=CARTESIAN_POINT ( 'NONE',  ( 10.09961440033846181, -3660.701366163754301, 2250.195255585644190 ) ) ;
#19528=CARTESIAN_POINT ( 'NONE',  ( 76.20000000000000284, -3670.300000000000182, 2239.771999999999935 ) ) ;
#19530=CARTESIAN_POINT ( 'NONE',  ( 142.4730239663999782, -3578.859999866000180, 2250.236800057000437 ) ) ;
#19531=CARTESIAN_POINT ( 'NONE',  ( 14.82309358269936261, -3657.611473550246956, 2248.695702319098473 ) ) ;
#19532=CYLINDRICAL_SURFACE ( 'NONE', #19556, 2.844800000000001550 ) ;
#19533=ORIENTED_EDGE ( 'NONE', *, *, #8556, .F. ) ;
#19534=CARTESIAN_POINT ( 'NONE',  ( 9.926985991717000246, -3578.860012824000023, 2250.236835079999764 ) ) ;
#19538=CARTESIAN_POINT ( 'NONE',  ( 132.2269032045000188, -3544.443975155000317, 2260.454626673999883 ) ) ;
#19543=EDGE_CURVE ( 'NONE', #17962, #15313, #13652, .T. ) ;
#19548=DIRECTION ( 'NONE',  ( 1.000000000000000000, 0.000000000000000000, 0.000000000000000000 ) ) ;
#19550=CARTESIAN_POINT ( 'NONE',  ( 17.37165482607458245, -3576.201487277430260, 2246.367956099597450 ) ) ;
#19552=PLANE ( 'NONE',  #18121 ) ;
#19553=ORIENTED_EDGE ( 'NONE', *, *, #3295, .T. ) ;
#19554=AXIS2_PLACEMENT_3D ( 'NONE', #16484, #11105, #16147 ) ;
#19555=DIRECTION ( 'NONE',  ( 1.224646799147353207E-16, 1.000000000000000000, -0.000000000000000000 ) ) ;
#19556=AXIS2_PLACEMENT_3D ( 'NONE', #14268, #1954, #10508 ) ;
#19559=CARTESIAN_POINT ( 'NONE',  ( 116.8400000000000034, -3543.300000000000182, 2251.506800000000112 ) ) ;
#19561=DIRECTION ( 'NONE',  ( 1.000000000000000000, 0.000000000000000000, 0.000000000000000000 ) ) ;
#19563=ADVANCED_FACE ( 'NONE', ( #12895 ), #12535, .T. ) ;
#19567=ORIENTED_EDGE ( 'NONE', *, *, #7816, .T. ) ;
#19568=CIRCLE ( 'NONE', #22544, 0.7619999999999294005 ) ;
#19569=CYLINDRICAL_SURFACE ( 'NONE', #1389, 2.844800000000091700 ) ;
#19572=LINE ( 'NONE', #17920, #20947 ) ;
#19575=ADVANCED_FACE ( 'NONE', ( #12664 ), #11419, .T. ) ;
#19577=DIRECTION ( 'NONE',  ( 0.000000000000000000, 0.000000000000000000, -1.000000000000000000 ) ) ;
#19578=ORIENTED_EDGE ( 'NONE', *, *, #2060, .F. ) ;
#19580=CARTESIAN_POINT ( 'NONE',  ( 15.54875643158000642, -3695.598810868058536, 2255.000779105261699 ) ) ;
#19581=ADVANCED_FACE ( 'NONE', ( #20276 ), #7324, .T. ) ;
#19582=EDGE_CURVE ( 'NONE', #6627, #20964, #18900, .T. ) ;
#19583=DIRECTION ( 'NONE',  ( 0.000000000000000000, 0.000000000000000000, -1.000000000000000000 ) ) ;
#19584=ORIENTED_EDGE ( 'NONE', *, *, #2524, .F. ) ;
#19585=CARTESIAN_POINT ( 'NONE',  ( 4.752492555451421907, -3695.617810901896064, 2259.779947940402053 ) ) ;
#19586=CARTESIAN_POINT ( 'NONE',  ( 15.24000000000000021, -3544.570000000000164, 2255.774000000000342 ) ) ;
#19588=TOROIDAL_SURFACE ( 'NONE', #4605, 4.114799999999999791, 1.270000000000000018 ) ;
#19589=CARTESIAN_POINT ( 'NONE',  ( 116.8400000000000034, -3670.300000000000182, 2247.392000000000280 ) ) ;
#19590=EDGE_LOOP ( 'NONE', ( #10368, #19122, #18076, #16265 ) ) ;
#19591=DIRECTION ( 'NONE',  ( 0.000000000000000000, 0.000000000000000000, -1.000000000000000000 ) ) ;
#19592=CARTESIAN_POINT ( 'NONE',  ( 73.35520000000001062, -3568.700000000000273, 2259.837999999999738 ) ) ;
#19594=CARTESIAN_POINT ( 'NONE',  ( 25.39999999999999858, -3619.500000000000000, 2261.869999999999891 ) ) ;
#19596=CARTESIAN_POINT ( 'NONE',  ( 18.03837739911582716, -3577.416356074214946, 2244.919848787751107 ) ) ;
#19601=VERTEX_POINT ( 'NONE', #18164 ) ;
#19603=CARTESIAN_POINT ( 'NONE',  ( 9.958250541862835092, -3695.444958116419457, 2255.268480149500647 ) ) ;
#19604=ORIENTED_EDGE ( 'NONE', *, *, #22684, .F. ) ;
#19606=CARTESIAN_POINT ( 'NONE',  ( 137.9036726380650748, -3657.299095976264653, 2247.222869807297684 ) ) ;
#19608=DIRECTION ( 'NONE',  ( -1.000000000000000000, 0.000000000000000000, 0.000000000000000000 ) ) ;
#19610=ORIENTED_EDGE ( 'NONE', *, *, #2958, .F. ) ;
#19611=ORIENTED_EDGE ( 'NONE', *, *, #19172, .T. ) ;
#19612=ORIENTED_EDGE ( 'NONE', *, *, #7805, .T. ) ;
#19613=CIRCLE ( 'NONE', #7630, 0.7619999999999294005 ) ;
#19617=CARTESIAN_POINT ( 'NONE',  ( 4.752632297182751486, -3543.382189098389972, 2259.779892145590566 ) ) ;
#19620=CARTESIAN_POINT ( 'NONE',  ( 151.4000000000000057, -3694.430000000000291, 2260.570967364599255 ) ) ;
#19621=VERTEX_POINT ( 'NONE', #16519 ) ;
#19622=DIRECTION ( 'NONE',  ( 0.000000000000000000, 0.000000000000000000, -1.000000000000000000 ) ) ;
#19623=DIRECTION ( 'NONE',  ( 0.000000000000000000, 1.000000000000000000, 0.000000000000000000 ) ) ;
#19626=EDGE_CURVE ( 'NONE', #16091, #8900, #4681, .T. ) ;
#19629=AXIS2_PLACEMENT_3D ( 'NONE', #20354, #6069, #16825 ) ;
#19632=CIRCLE ( 'NONE', #14770, 3.606800000000000228 ) ;
#19633=ORIENTED_EDGE ( 'NONE', *, *, #15254, .F. ) ;
#19636=CARTESIAN_POINT ( 'NONE',  ( 144.4597169060923534, -3576.330748743867389, 2246.087205944029847 ) ) ;
#19637=FACE_OUTER_BOUND ( 'NONE', #13595, .T. ) ;
#19638=FACE_OUTER_BOUND ( 'NONE', #16687, .T. ) ;
#19640=CARTESIAN_POINT ( 'NONE',  ( 18.22188905710634899, -3658.031438926708688, 2245.481214767577967 ) ) ;
#19642=TOROIDAL_SURFACE ( 'NONE', #14835, 4.114799999999999791, 1.270000000000000018 ) ;
#19643=DIRECTION ( 'NONE',  ( 0.000000000000000000, 0.000000000000000000, -1.000000000000000000 ) ) ;
#19647=APPLICATION_CONTEXT ( 'configuration controlled 3d designs of mechanical parts and assemblies' ) ;
#19648=DIRECTION ( 'NONE',  ( 0.000000000000000000, 1.000000000000000000, 0.000000000000000000 ) ) ;
#19649=AXIS2_PLACEMENT_3D ( 'NONE', #7888, #9863, #18656 ) ;
#19650=CARTESIAN_POINT ( 'NONE',  ( 14.65200945848731351, -3657.435257283903866, 2248.274806926763176 ) ) ;
#19652=VERTEX_POINT ( 'NONE', #11696 ) ;
#19658=DIRECTION ( 'NONE',  ( -1.000000000000000000, 0.000000000000000000, 0.000000000000000000 ) ) ;
#19660=CARTESIAN_POINT ( 'NONE',  ( 151.1299999999999955, -3543.299999999999727, 2259.329999999999927 ) ) ;
#19661=AXIS2_PLACEMENT_3D ( 'NONE', #16555, #15265, #507 ) ;
#19664=AXIS2_PLACEMENT_3D ( 'NONE', #18826, #780, #11666 ) ;
#19665=CIRCLE ( 'NONE', #9558, 2.844800000000091700 ) ;
#19666=ORIENTED_EDGE ( 'NONE', *, *, #17016, .F. ) ;
#19667=CARTESIAN_POINT ( 'NONE',  ( 50.79999999999999716, -3670.300000000000182, 2259.837999999999738 ) ) ;
#19669=FACE_OUTER_BOUND ( 'NONE', #16454, .T. ) ;
#19671=DIRECTION ( 'NONE',  ( -1.000000000000000000, 0.000000000000000000, 0.000000000000000000 ) ) ;
#19673=ORIENTED_EDGE ( 'NONE', *, *, #2549, .F. ) ;
#19675=ADVANCED_FACE ( 'NONE', ( #17202 ), #20408, .T. ) ;
#19676=ORIENTED_EDGE ( 'NONE', *, *, #17890, .T. ) ;
#19677=CARTESIAN_POINT ( 'NONE',  ( 142.2521248979318784, -3694.709202398072648, 2255.743570596264817 ) ) ;
#19678=DIRECTION ( 'NONE',  ( 0.000000000000000000, 0.000000000000000000, 1.000000000000000000 ) ) ;
#19681=CIRCLE ( 'NONE', #1711, 0.7619999999999294005 ) ;
#19682=VERTEX_POINT ( 'NONE', #22240 ) ;
#19684=EDGE_CURVE ( 'NONE', #6769, #17073, #2821, .T. ) ;
#19687=AXIS2_PLACEMENT_3D ( 'NONE', #9242, #4075, #10994 ) ;
#19688=CARTESIAN_POINT ( 'NONE',  ( 137.5277363187835249, -3581.332105450641393, 2248.799968448360687 ) ) ;
#19689=ORIENTED_EDGE ( 'NONE', *, *, #4385, .T. ) ;
#19690=CARTESIAN_POINT ( 'NONE',  ( 142.7470794804999912, -3543.299999999999727, 2254.503999999999905 ) ) ;
#19693=VECTOR ( 'NONE', #6456, 1000.000000000000000 ) ;
#19696=DIRECTION ( 'NONE',  ( 1.000000000000000000, 0.000000000000000000, 0.000000000000000000 ) ) ;
#19700=EDGE_CURVE ( 'NONE', #8573, #21672, #21174, .T. ) ;
#19704=CARTESIAN_POINT ( 'NONE',  ( 134.0212987838334584, -3578.851531742024690, 2244.547209130087140 ) ) ;
#19707=VERTEX_POINT ( 'NONE', #9939 ) ;
#19708=CARTESIAN_POINT ( 'NONE',  ( 4.891028678428722465, -3695.419680866766612, 2260.126887239455755 ) ) ;
#19715=ORIENTED_EDGE ( 'NONE', *, *, #1097, .T. ) ;
#19716=ADVANCED_FACE ( 'NONE', ( #6330 ), #13586, .F. ) ;
#19718=CARTESIAN_POINT ( 'NONE',  ( 15.47299515201000020, -3578.859991782000179, 2250.236800948000109 ) ) ;
#19720=CARTESIAN_POINT ( 'NONE',  ( 129.8447999999989975, -3670.300000000000182, 2261.869999999999891 ) ) ;
#19724=DIRECTION ( 'NONE',  ( 0.000000000000000000, 0.000000000000000000, 1.000000000000000000 ) ) ;
#19729=CARTESIAN_POINT ( 'NONE',  ( 137.8417952671095179, -3657.349591785569828, 2246.808273363673834 ) ) ;
#19730=EDGE_LOOP ( 'NONE', ( #922, #17203, #14012, #4172 ) ) ;
#19732=VERTEX_POINT ( 'NONE', #2795 ) ;
#19734=ORIENTED_EDGE ( 'NONE', *, *, #18673, .F. ) ;
#19735=AXIS2_PLACEMENT_3D ( 'NONE', #7179, #12682, #14447 ) ;
#19736=DIRECTION ( 'NONE',  ( 0.000000000000000000, 1.000000000000000000, 0.000000000000000000 ) ) ;
#19737=EDGE_LOOP ( 'NONE', ( #23148, #20657, #11457, #8971 ) ) ;
#19739=CYLINDRICAL_SURFACE ( 'NONE', #22863, 2.844799999998998796 ) ;
#19741=DIRECTION ( 'NONE',  ( -1.000000000000000000, 0.000000000000000000, 0.000000000000000000 ) ) ;
#19742=DIRECTION ( 'NONE',  ( -1.000000000000000000, 0.000000000000000000, 0.000000000000000000 ) ) ;
#19743=ORIENTED_EDGE ( 'NONE', *, *, #8824, .T. ) ;
#19745=PLANE ( 'NONE',  #13711 ) ;
#19746=AXIS2_PLACEMENT_3D ( 'NONE', #9509, #22039, #13138 ) ;
#19754=CARTESIAN_POINT ( 'NONE',  ( 131.7615871309722877, -3543.390959416002715, 2259.802598284109536 ) ) ;
#19757=CARTESIAN_POINT ( 'NONE',  ( 12.69999999999999929, -3659.504999999999654, 2255.774000000000342 ) ) ;
#19759=DIRECTION ( 'NONE',  ( 0.000000000000000000, 0.000000000000000000, -1.000000000000000000 ) ) ;
#19762=FACE_BOUND ( 'NONE', #20669, .T. ) ;
#19763=TOROIDAL_SURFACE ( 'NONE', #1033, 3.606799999999999784, 0.7620000000000000107 ) ;
#19765=CARTESIAN_POINT ( 'NONE',  ( 144.7935381745138557, -3576.902450837929791, 2245.303073078667239 ) ) ;
#19767=EDGE_CURVE ( 'NONE', #17500, #18712, #8313, .T. ) ;
#19769=EDGE_CURVE ( 'NONE', #6778, #2966, #22591, .T. ) ;
#19770=CARTESIAN_POINT ( 'NONE',  ( 18.11987658286814096, -3657.692177165366502, 2245.942492754456453 ) ) ;
#19771=ORIENTED_EDGE ( 'NONE', *, *, #15419, .F. ) ;
#19772=CARTESIAN_POINT ( 'NONE',  ( 147.4569508202075383, -3695.298184790736741, 2260.256966980285142 ) ) ;
#19773=DIRECTION ( 'NONE',  ( 0.000000000000000000, 0.000000000000000000, 1.000000000000000000 ) ) ;
#19777=CARTESIAN_POINT ( 'NONE',  ( 142.5057674346834915, -3543.452888078422802, 2255.108514515849038 ) ) ;
#19778=CARTESIAN_POINT ( 'NONE',  ( 110.6932000000009992, -3644.899999999999636, 2259.837999999999738 ) ) ;
#19779=CARTESIAN_POINT ( 'NONE',  ( 7.661546442962579029, -3576.797734221649080, 2245.432411850466451 ) ) ;
#19784=FACE_OUTER_BOUND ( 'NONE', #4730, .T. ) ;
#19791=DIRECTION ( 'NONE',  ( -1.000000000000000000, 0.000000000000000000, 0.000000000000000000 ) ) ;
#19792=CYLINDRICAL_SURFACE ( 'NONE', #20425, 1.269999999999900320 ) ;
#19793=EDGE_LOOP ( 'NONE', ( #7251, #22146, #11395, #17961, #7628, #7274 ) ) ;
#19795=ORIENTED_EDGE ( 'NONE', *, *, #17820, .T. ) ;
#19796=CARTESIAN_POINT ( 'NONE',  ( 142.3802386003915785, -3695.306816721881205, 2255.422803181790186 ) ) ;
#19797=CARTESIAN_POINT ( 'NONE',  ( 76.20000000000000284, -3568.700000000000273, 2239.771999999999935 ) ) ;
#19799=ORIENTED_EDGE ( 'NONE', *, *, #9265, .F. ) ;
#19800=CARTESIAN_POINT ( 'NONE',  ( 137.2808927978301199, -3580.991830095288151, 2249.275667250868992 ) ) ;
#19807=SPHERICAL_SURFACE ( 'NONE', #12991, 1.270000000000000018 ) ;
#19809=CARTESIAN_POINT ( 'NONE',  ( 20.62424768829000143, -3694.430000000000291, 2260.600000000000364 ) ) ;
#19810=EDGE_CURVE ( 'NONE', #15062, #16201, #15115, .T. ) ;
#19812=CARTESIAN_POINT ( 'NONE',  ( 138.9181842230315738, -3576.759674807602096, 2249.310742386851871 ) ) ;
#19813=ORIENTED_EDGE ( 'NONE', *, *, #13156, .F. ) ;
#19814=CARTESIAN_POINT ( 'NONE',  ( 142.2400000000000091, -3578.213872745999652, 2255.774000000000342 ) ) ;
#19817=ORIENTED_EDGE ( 'NONE', *, *, #2060, .T. ) ;
#19829=DIRECTION ( 'NONE',  ( 0.000000000000000000, 0.000000000000000000, 1.000000000000000000 ) ) ;
#19832=CARTESIAN_POINT ( 'NONE',  ( 76.20000000000000284, -3670.300000000000182, 2239.771999999999935 ) ) ;
#19835=CARTESIAN_POINT ( 'NONE',  ( 18.03606895320094594, -3581.542328871593327, 2246.419514926349166 ) ) ;
#19837=CARTESIAN_POINT ( 'NONE',  ( 137.4930112367257209, -3657.709449394080366, 2248.871353917016677 ) ) ;
#19838=EDGE_CURVE ( 'NONE', #5090, #22478, #20056, .T. ) ;
#19842=CARTESIAN_POINT ( 'NONE',  ( 138.5760044042908987, -3662.119678798826499, 2249.435431913212142 ) ) ;
#19843=EDGE_CURVE ( 'NONE', #15258, #5300, #11060, .T. ) ;
#19845=EDGE_LOOP ( 'NONE', ( #15725, #6649, #20310, #11568 ) ) ;
#19846=ORIENTED_EDGE ( 'NONE', *, *, #4777, .F. ) ;
#19848=FACE_OUTER_BOUND ( 'NONE', #1682, .T. ) ;
#19849=ORIENTED_EDGE ( 'NONE', *, *, #281, .T. ) ;
#19850=ORIENTED_EDGE ( 'NONE', *, *, #5288, .F. ) ;
#19853=DIRECTION ( 'NONE',  ( -1.000000000000000000, 0.000000000000000000, 0.000000000000000000 ) ) ;
#19855=ORIENTED_EDGE ( 'NONE', *, *, #15390, .T. ) ;
#19857=FACE_OUTER_BOUND ( 'NONE', #283, .T. ) ;
#19861=PLANE ( 'NONE',  #14490 ) ;
#19863=DIRECTION ( 'NONE',  ( -1.000000000000000000, 0.000000000000000000, 0.000000000000000000 ) ) ;
#19865=CARTESIAN_POINT ( 'NONE',  ( 137.1599999999999966, -3544.570000000000164, 2255.774000000000342 ) ) ;
#19867=CARTESIAN_POINT ( 'NONE',  ( 127.0000000000000000, -3619.500000000000000, 2259.837999999999738 ) ) ;
#19869=ORIENTED_EDGE ( 'NONE', *, *, #4910, .T. ) ;
#19876=ADVANCED_FACE ( 'NONE', ( #14286 ), #10643, .F. ) ;
#19877=AXIS2_PLACEMENT_3D ( 'NONE', #10853, #3699, #20117 ) ;
#19879=CARTESIAN_POINT ( 'NONE',  ( 18.07700247900687529, -3657.567912637663994, 2246.174638830017102 ) ) ;
#19881=CARTESIAN_POINT ( 'NONE',  ( 147.3682464508232783, -3694.976217803879081, 2260.479245238027033 ) ) ;
#19882=DIRECTION ( 'NONE',  ( 1.000000000000000000, 0.000000000000000000, 0.000000000000000000 ) ) ;
#19884=CARTESIAN_POINT ( 'NONE',  ( 105.2067999999999870, -3619.500000000000000, 2259.837999999999738 ) ) ;
#19885=CARTESIAN_POINT ( 'NONE',  ( 142.3627463449352604, -3543.741058433257422, 2255.466568423349599 ) ) ;
#19889=CARTESIAN_POINT ( 'NONE',  ( 7.831451107590767791, -3576.501952514877757, 2245.800612488090792 ) ) ;
#19890=VERTEX_POINT ( 'NONE', #7035 ) ;
#19892=DIRECTION ( 'NONE',  ( -0.000000000000000000, -1.000000000000000000, -0.000000000000000000 ) ) ;
#19897=AXIS2_PLACEMENT_3D ( 'NONE', #5414, #11026, #12672 ) ;
#19898=DIRECTION ( 'NONE',  ( 1.000000000000000000, 0.000000000000000000, 0.000000000000000000 ) ) ;
#19900=CYLINDRICAL_SURFACE ( 'NONE', #4462, 2.844800000000001550 ) ;
#19901=DIRECTION ( 'NONE',  ( 0.000000000000000000, 0.000000000000000000, -1.000000000000000000 ) ) ;
#19908=ORIENTED_EDGE ( 'NONE', *, *, #19582, .T. ) ;
#19913=CARTESIAN_POINT ( 'NONE',  ( 142.5942428639083062, -3695.644174312342329, 2254.886068105269260 ) ) ;
#19914=DIRECTION ( 'NONE',  ( 0.000000000000000000, 0.000000000000000000, 1.000000000000000000 ) ) ;
#19916=CARTESIAN_POINT ( 'NONE',  ( 137.5597807309948450, -3581.369168488304695, 2248.732576067342507 ) ) ;
#19918=LINE ( 'NONE', #19690, #17477 ) ;
#19920=AXIS2_PLACEMENT_3D ( 'NONE', #2087, #16599, #20681 ) ;
#19921=EDGE_CURVE ( 'NONE', #982, #16281, #2090, .T. ) ;
#19922=DIRECTION ( 'NONE',  ( 0.000000000000000000, 0.000000000000000000, -1.000000000000000000 ) ) ;
#19923=CARTESIAN_POINT ( 'NONE',  ( 8.088613972621001125, -3662.880847139000252, 2246.630000000000109 ) ) ;
#19925=AXIS2_PLACEMENT_3D ( 'NONE', #8185, #12913, #6434 ) ;
#19926=DIRECTION ( 'NONE',  ( 1.224646799147353207E-16, 1.000000000000000000, -0.000000000000000000 ) ) ;
#19927=AXIS2_PLACEMENT_3D ( 'NONE', #16501, #15094, #14757 ) ;
#19928=CARTESIAN_POINT ( 'NONE',  ( 138.3402197975327113, -3576.994575834084571, 2249.540499101924979 ) ) ;
#19929=ORIENTED_EDGE ( 'NONE', *, *, #939, .T. ) ;
#19930=CARTESIAN_POINT ( 'NONE',  ( 134.0716720153636743, -3578.501212890310853, 2244.568960851739121 ) ) ;
#19932=CARTESIAN_POINT ( 'NONE',  ( 137.1599999999999966, -3578.213872745999652, 2255.774000000000342 ) ) ;
#19935=CARTESIAN_POINT ( 'NONE',  ( 95.25000000000000000, -3568.700000000000273, 2247.392000000000280 ) ) ;
#19936=AXIS2_PLACEMENT_3D ( 'NONE', #18557, #17022, #968 ) ;
#19938=ORIENTED_EDGE ( 'NONE', *, *, #16012, .T. ) ;
#19942=EDGE_LOOP ( 'NONE', ( #1272, #8451, #19123, #17822 ) ) ;
#19944=DIRECTION ( 'NONE',  ( 0.000000000000000000, 1.000000000000000000, 0.000000000000000000 ) ) ;
#19946=B_SPLINE_CURVE_WITH_KNOTS ( 'NONE', 3,
 ( #17559, #5160, #8559, #6914, #11830, #2926, #21091, #6691, #18985, #10066, #21214, #13594, #17209, #1156, #19443, #19216, #1508, #6451, #8319, #19097, #15464, #14058 ),
 .UNSPECIFIED., .F., .F.,
 ( 4, 2, 2, 1, 2, 2, 2, 1, 2, 2, 2, 4 ),
 ( 0.000000000000000000, 0.1250000000009205414, 0.1875000000011848578, 0.2187500000013189450, 0.2343750000014777624, 0.2500000000016365798, 0.3750000000026065816, 0.4375000000028015368, 0.4687500000027456371, 0.5000000000026897373, 0.7500000000013449242, 1.000000000000000000 ),
 .UNSPECIFIED. ) ;
#19953=DIRECTION ( 'NONE',  ( 0.000000000000000000, -2.331176954594000018E-14, -1.000000000000000000 ) ) ;
#19954=FACE_OUTER_BOUND ( 'NONE', #2130, .T. ) ;
#19955=EDGE_LOOP ( 'NONE', ( #12761, #7262, #19964, #7668 ) ) ;
#19957=CARTESIAN_POINT ( 'NONE',  ( 137.7687556490391785, -3657.415903659005380, 2248.216200637740712 ) ) ;
#19960=VECTOR ( 'NONE', #22058, 1000.000000000000000 ) ;
#19961=CARTESIAN_POINT ( 'NONE',  ( 137.4266760222526500, -3661.215795996489760, 2250.025794176416184 ) ) ;
#19964=ORIENTED_EDGE ( 'NONE', *, *, #22888, .T. ) ;
#19969=ORIENTED_EDGE ( 'NONE', *, *, #829, .F. ) ;
#19973=EDGE_LOOP ( 'NONE', ( #21269, #2875, #12126, #12660 ) ) ;
#19975=EDGE_CURVE ( 'NONE', #16187, #19707, #20963, .T. ) ;
#19977=CARTESIAN_POINT ( 'NONE',  ( 7.231857318210721530, -3581.156156794382696, 2245.707491121732346 ) ) ;
#19980=DIRECTION ( 'NONE',  ( 0.000000000000000000, -1.000000000000000000, 0.000000000000000000 ) ) ;
#19982=EDGE_CURVE ( 'NONE', #11744, #10812, #12176, .T. ) ;
#19986=DIRECTION ( 'NONE',  ( 0.000000000000000000, 0.000000000000000000, -1.000000000000000000 ) ) ;
#19987=EDGE_CURVE ( 'NONE', #22201, #19890, #15178, .T. ) ;
#19988=ADVANCED_FACE ( 'NONE', ( #9356 ), #9468, .F. ) ;
#19990=ORIENTED_EDGE ( 'NONE', *, *, #13883, .F. ) ;
#19992=DIRECTION ( 'NONE',  ( -0.7249994335945012525, 0.000000000000000000, 0.6887494619146010688 ) ) ;
#19993=CIRCLE ( 'NONE', #2753, 2.844799999999994444 ) ;
#19994=ADVANCED_FACE ( 'NONE', ( #14634 ), #19792, .T. ) ;
#19996=DIRECTION ( 'NONE',  ( -0.000000000000000000, -1.000000000000000000, -0.000000000000000000 ) ) ;
#19999=DIRECTION ( 'NONE',  ( 0.000000000000000000, 0.000000000000000000, -1.000000000000000000 ) ) ;
#20001=CARTESIAN_POINT ( 'NONE',  ( 147.7813568978695002, -3695.700000000000728, 2259.444513961513167 ) ) ;
#20002=CARTESIAN_POINT ( 'NONE',  ( 25.39999999999999858, -3578.860000000000127, 2247.392000000000280 ) ) ;
#20006=AXIS2_PLACEMENT_3D ( 'NONE', #9822, #13347, #22237 ) ;
#20007=CARTESIAN_POINT ( 'NONE',  ( 7.478703374698133288, -3577.171362236310415, 2245.102579701181639 ) ) ;
#20008=VERTEX_POINT ( 'NONE', #7591 ) ;
#20012=CARTESIAN_POINT ( 'NONE',  ( 124.1552000000010025, -3568.700000000000273, 2259.837999999999738 ) ) ;
#20017=EDGE_CURVE ( 'NONE', #22588, #20273, #11221, .T. ) ;
#20020=EDGE_LOOP ( 'NONE', ( #19584, #2419, #17678, #15405 ) ) ;
#20021=FACE_OUTER_BOUND ( 'NONE', #22324, .T. ) ;
#20026=CARTESIAN_POINT ( 'NONE',  ( 79.04479999999999507, -3568.700000000000273, 2261.869999999999891 ) ) ;
#20028=CARTESIAN_POINT ( 'NONE',  ( 54.40679999999999694, -3619.500000000000000, 2260.600000000000364 ) ) ;
#20029=ADVANCED_FACE ( 'NONE', ( #16156 ), #11806, .T. ) ;
#20030=ORIENTED_EDGE ( 'NONE', *, *, #15180, .T. ) ;
#20031=CARTESIAN_POINT ( 'NONE',  ( 35.25520000000000209, -3594.099999999999909, 2261.869999999999891 ) ) ;
#20032=DIRECTION ( 'NONE',  ( 0.000000000000000000, 0.000000000000000000, 1.000000000000000000 ) ) ;
#20034=CARTESIAN_POINT ( 'NONE',  ( 137.7875023037999824, -3581.600928630999988, 2246.630000000000109 ) ) ;
#20036=AXIS2_PLACEMENT_3D ( 'NONE', #19238, #6477, #3296 ) ;
#20038=CARTESIAN_POINT ( 'NONE',  ( 145.4114788387173292, -3579.724573821726153, 2244.678944975163631 ) ) ;
#20043=VECTOR ( 'NONE', #23088, 1000.000000000000000 ) ;
#20044=FACE_OUTER_BOUND ( 'NONE', #20911, .T. ) ;
#20045=EDGE_CURVE ( 'NONE', #22687, #14575, #19681, .T. ) ;
#20047=CARTESIAN_POINT ( 'NONE',  ( 132.0583097651000060, -3544.202533098000458, 2260.545675974999995 ) ) ;
#20049=CARTESIAN_POINT ( 'NONE',  ( 141.4648100392906542, -3577.263639210850670, 2249.746746628647998 ) ) ;
#20051=ORIENTED_EDGE ( 'NONE', *, *, #16247, .F. ) ;
#20052=CARTESIAN_POINT ( 'NONE',  ( 134.4864491364314176, -3577.154038986648629, 2245.115470800847106 ) ) ;
#20053=ORIENTED_EDGE ( 'NONE', *, *, #12439, .F. ) ;
#20055=CARTESIAN_POINT ( 'NONE',  ( 137.1599999999999966, -3658.223872745999870, 2255.774000000000342 ) ) ;
#20056=CIRCLE ( 'NONE', #6572, 2.844799999999994444 ) ;
#20063=VECTOR ( 'NONE', #1415, 1000.000000000000000 ) ;
#20066=CARTESIAN_POINT ( 'NONE',  ( 15.22954893437939283, -3578.192778017456476, 2250.157666245888777 ) ) ;
#20068=PLANE ( 'NONE',  #22897 ) ;
#20073=CARTESIAN_POINT ( 'NONE',  ( 151.1299999999999955, -3695.699999999999818, 2259.329999999999927 ) ) ;
#20081=TOROIDAL_SURFACE ( 'NONE', #18556, 3.606799999999999784, 0.7620000000000000107 ) ;
#20082=CARTESIAN_POINT ( 'NONE',  ( 137.8325232038615127, -3661.651965462245698, 2249.802177248667249 ) ) ;
#20087=ORIENTED_EDGE ( 'NONE', *, *, #13388, .F. ) ;
#20089=CYLINDRICAL_SURFACE ( 'NONE', #7667, 2.844799999999994444 ) ;
#20090=EDGE_LOOP ( 'NONE', ( #1264, #14689, #166, #18416 ) ) ;
#20092=CARTESIAN_POINT ( 'NONE',  ( 136.6529205195000145, -3695.699999999999818, 2254.503999999999905 ) ) ;
#20093=FACE_BOUND ( 'NONE', #16528, .T. ) ;
#20094=CARTESIAN_POINT ( 'NONE',  ( 131.5729205195000020, -3543.299999999999727, 2259.329999999999927 ) ) ;
#20099=ORIENTED_EDGE ( 'NONE', *, *, #18454, .F. ) ;
#20101=CARTESIAN_POINT ( 'NONE',  ( 142.4930772826777456, -3658.963397008600623, 2249.982107089370857 ) ) ;
#20103=CARTESIAN_POINT ( 'NONE',  ( 7.107063980692033489, -3660.720702668381364, 2244.590566913373550 ) ) ;
#20105=AXIS2_PLACEMENT_3D ( 'NONE', #21450, #16171, #16056 ) ;
#20106=PLANE ( 'NONE',  #17056 ) ;
#20107=AXIS2_PLACEMENT_3D ( 'NONE', #11512, #15273, #17015 ) ;
#20109=EDGE_CURVE ( 'NONE', #15378, #13988, #7939, .T. ) ;
#20114=VERTEX_POINT ( 'NONE', #16725 ) ;
#20115=CARTESIAN_POINT ( 'NONE',  ( 18.13064428604669942, -3657.724554382803944, 2245.888502604037512 ) ) ;
#20116=VERTEX_POINT ( 'NONE', #16830 ) ;
#20117=DIRECTION ( 'NONE',  ( 1.000000000000000000, 0.000000000000000000, 0.000000000000000000 ) ) ;
#20120=CYLINDRICAL_SURFACE ( 'NONE', #17932, 2.844800000000091700 ) ;
#20121=CARTESIAN_POINT ( 'NONE',  ( 142.7470794804999912, -3543.299999999999727, 2254.503999999999905 ) ) ;
#20124=CARTESIAN_POINT ( 'NONE',  ( 7.114657506406928178, -3578.282732473625401, 2244.605386419569641 ) ) ;
#20125=ORIENTED_EDGE ( 'NONE', *, *, #17425, .F. ) ;
#20128=DIRECTION ( 'NONE',  ( 0.000000000000000000, -1.000000000000000000, 0.000000000000000000 ) ) ;
#20130=CIRCLE ( 'NONE', #14893, 2.844799999998998796 ) ;
#20134=ORIENTED_EDGE ( 'NONE', *, *, #1625, .T. ) ;
#20136=ORIENTED_EDGE ( 'NONE', *, *, #10226, .F. ) ;
#20144=ORIENTED_EDGE ( 'NONE', *, *, #4933, .T. ) ;
#20145=DIRECTION ( 'NONE',  ( -1.000000000000000000, 0.000000000000000000, 0.000000000000000000 ) ) ;
#20146=DIRECTION ( 'NONE',  ( 0.000000000000000000, -1.000000000000000000, 0.000000000000000000 ) ) ;
#20147=CIRCLE ( 'NONE', #6295, 2.844799999998998796 ) ;
#20148=EDGE_LOOP ( 'NONE', ( #16594, #15459, #8844, #4395, #23116, #16874, #5894, #20282 ) ) ;
#20150=DIRECTION ( 'NONE',  ( -1.000000000000000000, 0.000000000000000000, 0.000000000000000000 ) ) ;
#20151=ORIENTED_EDGE ( 'NONE', *, *, #18401, .T. ) ;
#20154=CARTESIAN_POINT ( 'NONE',  ( 145.3077377672685202, -3580.597427896025692, 2245.138331176687188 ) ) ;
#20156=CARTESIAN_POINT ( 'NONE',  ( 145.3824765374318133, -3578.886079828094807, 2244.547288873628986 ) ) ;
#20157=CARTESIAN_POINT ( 'NONE',  ( 18.28255762641966342, -3660.729247660008696, 2244.607872304181456 ) ) ;
#20158=DIRECTION ( 'NONE',  ( 0.000000000000000000, 0.000000000000000000, -1.000000000000000000 ) ) ;
#20159=DIRECTION ( 'NONE',  ( -1.000000000000000000, 0.000000000000000000, 0.000000000000000000 ) ) ;
#20160=CARTESIAN_POINT ( 'NONE',  ( 138.9028968162981243, -3576.764073753475259, 2249.315552100089917 ) ) ;
#20162=CARTESIAN_POINT ( 'NONE',  ( 59.89320000000000022, -3594.099999999999909, 2239.009999999999764 ) ) ;
#20164=PLANE ( 'NONE',  #23013 ) ;
#20168=EDGE_LOOP ( 'NONE', ( #85, #744, #13894, #16955, #15640, #14643, #21940, #21778, #15841, #1986 ) ) ;
#20171=CARTESIAN_POINT ( 'NONE',  ( 15.49342176171425223, -3658.963902681101899, 2249.982338889249604 ) ) ;
#20173=DIRECTION ( 'NONE',  ( 0.000000000000000000, 0.000000000000000000, 1.000000000000000000 ) ) ;
#20174=CARTESIAN_POINT ( 'NONE',  ( 14.78006840248709608, -3577.552158459792736, 2249.919509794231089 ) ) ;
#20176=DIRECTION ( 'NONE',  ( 0.6887494619146010688, 0.000000000000000000, -0.7249994335945012525 ) ) ;
#20177=EDGE_CURVE ( 'NONE', #15879, #22049, #20821, .T. ) ;
#20184=CARTESIAN_POINT ( 'NONE',  ( 18.13332411963230584, -3581.267160281976885, 2245.875868927712418 ) ) ;
#20186=CARTESIAN_POINT ( 'NONE',  ( 151.1299999999999955, -3694.430000000000291, 2240.279999999999745 ) ) ;
#20189=CIRCLE ( 'NONE', #19433, 0.7619999999999294005 ) ;
#20190=CARTESIAN_POINT ( 'NONE',  ( 141.5845584249510978, -3661.638084686768707, 2249.811463398476462 ) ) ;
#20196=DIRECTION ( 'NONE',  ( 0.000000000000000000, 0.000000000000000000, -1.000000000000000000 ) ) ;
#20202=DIRECTION ( 'NONE',  ( 0.000000000000000000, 0.000000000000000000, -1.000000000000000000 ) ) ;
#20205=AXIS2_PLACEMENT_3D ( 'NONE', #22422, #15762, #4623 ) ;
#20206=DIRECTION ( 'NONE',  ( 0.000000000000000000, 0.000000000000000000, -1.000000000000000000 ) ) ;
#20209=ORIENTED_EDGE ( 'NONE', *, *, #6251, .F. ) ;
#20210=CARTESIAN_POINT ( 'NONE',  ( 142.5172131144081789, -3659.103360921763397, 2250.042044413348322 ) ) ;
#20212=EDGE_LOOP ( 'NONE', ( #21661, #18420, #20741, #15047 ) ) ;
#20213=DIRECTION ( 'NONE',  ( 0.000000000000000000, -1.000000000000000000, 0.000000000000000000 ) ) ;
#20214=AXIS2_PLACEMENT_3D ( 'NONE', #13112, #11010, #16745 ) ;
#20216=CARTESIAN_POINT ( 'NONE',  ( 127.0000000000000000, -3660.140000000000327, 2244.547199999999975 ) ) ;
#20217=DIRECTION ( 'NONE',  ( -0.000000000000000000, -1.000000000000000000, -0.000000000000000000 ) ) ;
#20221=CARTESIAN_POINT ( 'NONE',  ( 147.6115783649720186, -3695.579670240918858, 2259.869798073102174 ) ) ;
#20225=CARTESIAN_POINT ( 'NONE',  ( 101.5999999999999943, -3670.300000000000182, 2261.869999999999891 ) ) ;
#20229=VERTEX_POINT ( 'NONE', #20576 ) ;
#20232=EDGE_CURVE ( 'NONE', #10874, #4775, #3969, .T. ) ;
#20233=CARTESIAN_POINT ( 'NONE',  ( 92.50679999999999836, -3644.899999999999636, 2259.837999999999738 ) ) ;
#20238=CARTESIAN_POINT ( 'NONE',  ( 104.4447999999999865, -3568.700000000000273, 2259.837999999999738 ) ) ;
#20239=ORIENTED_EDGE ( 'NONE', *, *, #18815, .T. ) ;
#20240=CARTESIAN_POINT ( 'NONE',  ( 134.8376892655312815, -3662.508216201634241, 2245.815664034198107 ) ) ;
#20243=EDGE_LOOP ( 'NONE', ( #1042, #12715, #10636, #1282, #9627, #17259 ) ) ;
#20244=CARTESIAN_POINT ( 'NONE',  ( 14.48593475403758468, -3661.719383861308415, 2249.758098224367586 ) ) ;
#20246=VERTEX_POINT ( 'NONE', #6768 ) ;
#20253=ORIENTED_EDGE ( 'NONE', *, *, #18659, .F. ) ;
#20254=FACE_OUTER_BOUND ( 'NONE', #20399, .T. ) ;
#20256=ORIENTED_EDGE ( 'NONE', *, *, #16681, .F. ) ;
#20258=AXIS2_PLACEMENT_3D ( 'NONE', #21522, #17152, #13414 ) ;
#20259=ADVANCED_FACE ( 'NONE', ( #16013 ), #5861, .T. ) ;
#20263=ORIENTED_EDGE ( 'NONE', *, *, #12161, .F. ) ;
#20267=DIRECTION ( 'NONE',  ( 0.000000000000000000, 0.000000000000000000, -1.000000000000000000 ) ) ;
#20269=CARTESIAN_POINT ( 'NONE',  ( 17.91090713674469015, -3661.851834046207841, 2245.119883787194794 ) ) ;
#20272=CARTESIAN_POINT ( 'NONE',  ( 140.9034509249830194, -3576.915841627701411, 2249.469465256947387 ) ) ;
#20273=VERTEX_POINT ( 'NONE', #10150 ) ;
#20275=TOROIDAL_SURFACE ( 'NONE', #5682, 3.606799999999999784, 0.7620000000000000107 ) ;
#20276=FACE_OUTER_BOUND ( 'NONE', #20090, .T. ) ;
#20278=B_SPLINE_CURVE_WITH_KNOTS ( 'NONE', 3,
 ( #14117, #13999, #21030, #4848, #5324, #13769, #19617, #12000, #21149, #5094, #1328, #19386, #8495, #10593, #3320, #17501, #10472, #17617, #19498, #8725, #10709, #23000, #5211, #17856 ),
 .UNSPECIFIED., .F., .F.,
 ( 4, 2, 2, 1, 1, 1, 2, 2, 2, 2, 1, 2, 2, 4 ),
 ( 0.000000000000000000, 0.1250000000047984672, 0.1875000000071320172, 0.2187500000086201601, 0.2343750000093642316, 0.2421875000097362673, 0.2460937500095420061, 0.2500000000093477448, 0.3750000000084149354, 0.4375000000078757556, 0.4687500000073991369, 0.4843750000071607720, 0.5000000000069223516, 1.000000000000000000 ),
 .UNSPECIFIED. ) ;
#20279=EDGE_CURVE ( 'NONE', #11877, #19707, #18934, .T. ) ;
#20282=ORIENTED_EDGE ( 'NONE', *, *, #2524, .T. ) ;
#20283=DIRECTION ( 'NONE',  ( 0.000000000000000000, 0.000000000000000000, -1.000000000000000000 ) ) ;
#20285=CARTESIAN_POINT ( 'NONE',  ( 124.1552000000010025, -3619.500000000000000, 2261.869999999999891 ) ) ;
#20286=CARTESIAN_POINT ( 'NONE',  ( 12.15970647189616116, -3576.701128706128202, 2249.244750392014794 ) ) ;
#20288=CARTESIAN_POINT ( 'NONE',  ( 141.6584232981540765, -3581.559207404357039, 2248.295745760272894 ) ) ;
#20289=EDGE_LOOP ( 'NONE', ( #9905, #9500, #7488, #7969 ) ) ;
#20291=LINE ( 'NONE', #11374, #11491 ) ;
#20296=CARTESIAN_POINT ( 'NONE',  ( 5.080000000000000071, -3694.430000000000291, 2260.600000000000364 ) ) ;
#20298=CARTESIAN_POINT ( 'NONE',  ( 20.66653435520565907, -3543.365340577194729, 2259.732141854306974 ) ) ;
#20303=CIRCLE ( 'NONE', #17662, 2.844799999998995244 ) ;
#20306=ORIENTED_EDGE ( 'NONE', *, *, #17954, .T. ) ;
#20310=ORIENTED_EDGE ( 'NONE', *, *, #23119, .T. ) ;
#20311=CARTESIAN_POINT ( 'NONE',  ( 20.82707948048999924, -3695.699999999999818, 2259.329999999999927 ) ) ;
#20317=( LENGTH_UNIT ( ) NAMED_UNIT ( * ) SI_UNIT ( .MILLI., .METRE. ) );
#20318=DIRECTION ( 'NONE',  ( 0.000000000000000000, 0.000000000000000000, 1.000000000000000000 ) ) ;
#20319=DIRECTION ( 'NONE',  ( 0.000000000000000000, 0.000000000000000000, -1.000000000000000000 ) ) ;
#20320=CIRCLE ( 'NONE', #12823, 2.844799999999994444 ) ;
#20322=CARTESIAN_POINT ( 'NONE',  ( 151.4000000000000057, -3660.140000000000327, 2250.265832635400784 ) ) ;
#20326=DIRECTION ( 'NONE',  ( -1.000000000000000000, 0.000000000000000000, 0.000000000000000000 ) ) ;
#20328=DIRECTION ( 'NONE',  ( 0.000000000000000000, 0.000000000000000000, 1.000000000000000000 ) ) ;
#20330=DIRECTION ( 'NONE',  ( 0.000000000000000000, 0.000000000000000000, 1.000000000000000000 ) ) ;
#20333=CIRCLE ( 'NONE', #7989, 0.7619999999999294005 ) ;
#20336=EDGE_LOOP ( 'NONE', ( #264, #14326 ) ) ;
#20337=ORIENTED_EDGE ( 'NONE', *, *, #21107, .T. ) ;
#20342=EDGE_CURVE ( 'NONE', #14706, #6665, #22865, .T. ) ;
#20344=FACE_OUTER_BOUND ( 'NONE', #8558, .T. ) ;
#20353=CARTESIAN_POINT ( 'NONE',  ( 134.8815275705442502, -3662.578409907537662, 2245.925647646461130 ) ) ;
#20354=CARTESIAN_POINT ( 'NONE',  ( 139.6999999999999886, -3579.494999999999891, 2246.630000000000109 ) ) ;
#20356=CARTESIAN_POINT ( 'NONE',  ( 54.40679999999999694, -3568.700000000000273, 2239.009999999999764 ) ) ;
#20357=CARTESIAN_POINT ( 'NONE',  ( 13.23165581431225846, -3662.300617105160200, 2249.242775709399211 ) ) ;
#20359=VERTEX_POINT ( 'NONE', #22792 ) ;
#20363=CARTESIAN_POINT ( 'NONE',  ( 63.50000000000000000, -3644.899999999999636, 2261.869999999999891 ) ) ;
#20367=VERTEX_POINT ( 'NONE', #8753 ) ;
#20371=CARTESIAN_POINT ( 'NONE',  ( 17.91260410565400463, -3661.848063305847063, 2245.117046218366340 ) ) ;
#20373=DIRECTION ( 'NONE',  ( -1.000000000000000000, 0.000000000000000000, 0.000000000000000000 ) ) ;
#20379=CARTESIAN_POINT ( 'NONE',  ( 7.363939561626733799, -3657.457649646252776, 2246.419592195776659 ) ) ;
#20380=EDGE_CURVE ( 'NONE', #7706, #4416, #4696, .T. ) ;
#20381=CARTESIAN_POINT ( 'NONE',  ( 35.56000000000000227, -3544.570000000000164, 2243.277199999999993 ) ) ;
#20384=DIRECTION ( 'NONE',  ( 0.000000000000000000, 0.000000000000000000, -1.000000000000000000 ) ) ;
#20386=ADVANCED_FACE ( 'NONE', ( #18109 ), #21637, .F. ) ;
#20390=AXIS2_PLACEMENT_3D ( 'NONE', #11413, #20544, #18570 ) ;
#20391=AXIS2_PLACEMENT_3D ( 'NONE', #8340, #18335, #7670 ) ;
#20392=ORIENTED_EDGE ( 'NONE', *, *, #19843, .F. ) ;
#20393=CIRCLE ( 'NONE', #929, 2.873832635400752622 ) ;
#20395=CARTESIAN_POINT ( 'NONE',  ( 15.39520459006179287, -3578.572279200602679, 2250.225720840873237 ) ) ;
#20398=CARTESIAN_POINT ( 'NONE',  ( 142.0826489325229147, -3581.049212494424410, 2249.208663835029711 ) ) ;
#20399=EDGE_LOOP ( 'NONE', ( #22971, #16249, #3878, #16915, #7902, #12879 ) ) ;
#20400=CARTESIAN_POINT ( 'NONE',  ( 151.1299999999999955, -3694.430000000000291, 2240.279999999999745 ) ) ;
#20404=EDGE_CURVE ( 'NONE', #8967, #14295, #14608, .T. ) ;
#20406=AXIS2_PLACEMENT_3D ( 'NONE', #10443, #15839, #22970 ) ;
#20407=EDGE_LOOP ( 'NONE', ( #3475, #14528, #4766, #12258 ) ) ;
#20408=TOROIDAL_SURFACE ( 'NONE', #8069, 4.114799999999999791, 1.270000000000000018 ) ;
#20409=DIRECTION ( 'NONE',  ( 0.000000000000000000, 0.000000000000000000, -1.000000000000000000 ) ) ;
#20410=CIRCLE ( 'NONE', #6574, 4.114799999999974034 ) ;
#20412=ORIENTED_EDGE ( 'NONE', *, *, #16807, .F. ) ;
#20413=EDGE_LOOP ( 'NONE', ( #2942, #5512, #13427, #21835 ) ) ;
#20415=ADVANCED_FACE ( 'NONE', ( #11087 ), #21934, .T. ) ;
#20418=LINE ( 'NONE', #623, #21013 ) ;
#20421=LINE ( 'NONE', #20527, #9967 ) ;
#20425=AXIS2_PLACEMENT_3D ( 'NONE', #16385, #5962, #14402 ) ;
#20429=DIRECTION ( 'NONE',  ( 1.000000000000000000, 0.000000000000000000, 0.000000000000000000 ) ) ;
#20430=VERTEX_POINT ( 'NONE', #21969 ) ;
#20434=ORIENTED_EDGE ( 'NONE', *, *, #13874, .T. ) ;
#20435=CARTESIAN_POINT ( 'NONE',  ( 137.0453141145324309, -3543.765301131294109, 2255.486744313127929 ) ) ;
#20438=B_SPLINE_CURVE_WITH_KNOTS ( 'NONE', 3,
 ( #19718, #20506, #20395, #13131, #9729, #20066, #2246, #14906, #16530, #9396, #18293, #13243, #15014, #6230, #7865, #9840, #2478, #20174, #7981, #18407, #600, #16643, #13029, #18521, #22033, #9620, #22144, #21925, #16766, #2363, #6344, #2582, #485, #7625, #7754, #5997, #5892, #814, #11486, #6117, #18636, #14786, #20286, #4114, #11259, #9502, #4347, #16871, #13364, #15126, #16984, #711, #4232, #22255, #11369, #4454, #11592, #18743, #2692, #931, #8099, #15244, #22371, #4004, #11152, #1842, #7017, #6457, #20862, #17773, #3474, #12390, #15471, #11711, #19423, #21416, #14159, #19534 ),
 .UNSPECIFIED., .F., .F.,
 ( 4, 2, 2, 1, 2, 2, 2, 1, 2, 2, 2, 1, 2, 2, 2, 2, 2, 2, 1, 2, 2, 2, 2, 2, 1, 2, 2, 2, 2, 2, 2, 1, 2, 2, 2, 1, 2, 2, 2, 1, 2, 2, 4 ),
 ( 0.000000000000000000, 0.06249999999819785823, 0.09374999999739346002, 0.1093749999970090869, 0.1171874999969127751, 0.1249999999968164632, 0.1562499999965751007, 0.1718749999963936348, 0.1796874999963606334, 0.1874999999963276320, 0.2187499999966426856, 0.2343749999967737474, 0.2421874999968235131, 0.2499999999968732789, 0.2812499999972781217, 0.2968749999974463205, 0.3124999999976144638, 0.3437499999978942400, 0.3593749999980610510, 0.3671874999981183940, 0.3749999999981757370, 0.4999999999991848743, 0.5624999999996890265, 0.5937499999999581446, 0.6093750000000727196, 0.6171875000001783018, 0.6250000000002837730, 0.6562500000007047696, 0.6718750000008879564, 0.6875000000010711432, 0.7187500000014369617, 0.7343750000015929480, 0.7421875000016709967, 0.7500000000017490454, 0.7812500000019865221, 0.7968750000020596858, 0.8046875000020707880, 0.8125000000020818902, 0.8437500000016395774, 0.8593750000013337109, 0.8671875000012222445, 0.8750000000011106671, 1.000000000000000000 ),
 .UNSPECIFIED. ) ;
#20439=EDGE_LOOP ( 'NONE', ( #11175, #405, #17101, #18301 ) ) ;
#20447=CARTESIAN_POINT ( 'NONE',  ( 20.25432815367999950, -3694.678775005999796, 2260.506484774000000 ) ) ;
#20450=ADVANCED_FACE ( 'NONE', ( #7562 ), #12725, .F. ) ;
#20451=EDGE_CURVE ( 'NONE', #16435, #16187, #13665, .T. ) ;
#20456=CARTESIAN_POINT ( 'NONE',  ( 7.953724235889067629, -3576.303814212001726, 2246.097598271465813 ) ) ;
#20457=VERTEX_POINT ( 'NONE', #980 ) ;
#20461=DIRECTION ( 'NONE',  ( 0.000000000000000000, 0.000000000000000000, -1.000000000000000000 ) ) ;
#20465=EDGE_CURVE ( 'NONE', #473, #10571, #21578, .T. ) ;
#20466=LINE ( 'NONE', #9788, #14459 ) ;
#20470=CARTESIAN_POINT ( 'NONE',  ( 134.6160622235418884, -3576.882542126288627, 2245.342794667374164 ) ) ;
#20471=ORIENTED_EDGE ( 'NONE', *, *, #22986, .F. ) ;
#20472=CARTESIAN_POINT ( 'NONE',  ( 5.080000000000000071, -3544.570000000000164, 2260.600000000000364 ) ) ;
#20473=DIRECTION ( 'NONE',  ( 0.000000000000000000, 0.000000000000000000, -1.000000000000000000 ) ) ;
#20474=DIRECTION ( 'NONE',  ( 0.000000000000000000, 0.000000000000000000, -1.000000000000000000 ) ) ;
#20477=DIRECTION ( 'NONE',  ( -1.000000000000000000, 0.000000000000000000, 0.000000000000000000 ) ) ;
#20481=ORIENTED_EDGE ( 'NONE', *, *, #15467, .F. ) ;
#20486=ORIENTED_EDGE ( 'NONE', *, *, #15049, .T. ) ;
#20489=CARTESIAN_POINT ( 'NONE',  ( 17.91462652069883177, -3661.843557398242410, 2245.113670094950066 ) ) ;
#20490=DIRECTION ( 'NONE',  ( -1.000000000000000000, 0.000000000000000000, 0.000000000000000000 ) ) ;
#20493=DIRECTION ( 'NONE',  ( -1.000000000000000000, -5.378139827789999268E-13, 1.344534956946999995E-13 ) ) ;
#20497=ORIENTED_EDGE ( 'NONE', *, *, #3399, .T. ) ;
#20498=DIRECTION ( 'NONE',  ( 0.000000000000000000, 0.000000000000000000, -1.000000000000000000 ) ) ;
#20505=CARTESIAN_POINT ( 'NONE',  ( 142.2400000000000091, -3658.223872745999870, 2255.774000000000342 ) ) ;
#20506=CARTESIAN_POINT ( 'NONE',  ( 15.43982607913381244, -3578.715157675396313, 2250.236799999999675 ) ) ;
#20508=CARTESIAN_POINT ( 'NONE',  ( 142.5448000000000093, -3579.687792440064641, 2250.120875928858368 ) ) ;
#20509=ORIENTED_EDGE ( 'NONE', *, *, #1771, .F. ) ;
#20510=CARTESIAN_POINT ( 'NONE',  ( 137.1599999999999966, -3580.776127254000130, 2255.774000000000342 ) ) ;
#20512=ADVANCED_FACE ( 'NONE', ( #11754 ), #10006, .T. ) ;
#20514=CARTESIAN_POINT ( 'NONE',  ( 20.68110872146951351, -3543.353673605964104, 2259.695705217817704 ) ) ;
#20521=ORIENTED_EDGE ( 'NONE', *, *, #3776, .F. ) ;
#20523=ORIENTED_EDGE ( 'NONE', *, *, #7926, .F. ) ;
#20525=DIRECTION ( 'NONE',  ( 0.000000000000000000, 0.000000000000000000, 1.000000000000000000 ) ) ;
#20527=CARTESIAN_POINT ( 'NONE',  ( 145.4150000000009868, -3579.494999999999891, 2246.630000000000109 ) ) ;
#20529=DIRECTION ( 'NONE',  ( 0.000000000000000000, -1.000000000000000000, 0.000000000000000000 ) ) ;
#20531=ADVANCED_FACE ( 'NONE', ( #9881 ), #13176, .F. ) ;
#20532=FACE_OUTER_BOUND ( 'NONE', #2659, .T. ) ;
#20541=CARTESIAN_POINT ( 'NONE',  ( 137.1118088725371251, -3544.023782198351910, 2255.653223149521637 ) ) ;
#20544=DIRECTION ( 'NONE',  ( 0.000000000000000000, 0.000000000000000000, -1.000000000000000000 ) ) ;
#20546=ORIENTED_EDGE ( 'NONE', *, *, #10154, .T. ) ;
#20548=EDGE_CURVE ( 'NONE', #15612, #20008, #11456, .T. ) ;
#20550=AXIS2_PLACEMENT_3D ( 'NONE', #12006, #22660, #13775 ) ;
#20555=CARTESIAN_POINT ( 'NONE',  ( 20.68102893033340095, -3695.646326397317353, 2259.695673346840522 ) ) ;
#20556=ORIENTED_EDGE ( 'NONE', *, *, #1097, .F. ) ;
#20562=EDGE_CURVE ( 'NONE', #21589, #5084, #6180, .T. ) ;
#20571=CARTESIAN_POINT ( 'NONE',  ( 144.9116092392395672, -3661.850275630491524, 2245.118708807381154 ) ) ;
#20576=CARTESIAN_POINT ( 'NONE',  ( 127.0000000000000000, -3660.140000000000327, 2250.236800000000130 ) ) ;
#20577=ORIENTED_EDGE ( 'NONE', *, *, #5868, .T. ) ;
#20579=CARTESIAN_POINT ( 'NONE',  ( 143.8794601179999972, -3581.600847530791270, 2246.630001408821499 ) ) ;
#20582=CARTESIAN_POINT ( 'NONE',  ( 15.44495085361937292, -3658.751901201893816, 2249.877081815448491 ) ) ;
#20589=AXIS2_PLACEMENT_3D ( 'NONE', #8818, #23093, #14210 ) ;
#20591=AXIS2_PLACEMENT_3D ( 'NONE', #17128, #6950, #1073 ) ;
#20592=ORIENTED_EDGE ( 'NONE', *, *, #3070, .T. ) ;
#20593=CARTESIAN_POINT ( 'NONE',  ( 145.3761992607832383, -3580.159608052688327, 2244.861392947937929 ) ) ;
#20596=DIRECTION ( 'NONE',  ( -1.000000000000000000, 0.000000000000000000, 0.000000000000000000 ) ) ;
#20599=EDGE_CURVE ( 'NONE', #14558, #3088, #22997, .T. ) ;
#20601=CARTESIAN_POINT ( 'NONE',  ( 137.3767596840099259, -3577.852638866662801, 2250.052719895559676 ) ) ;
#20606=EDGE_LOOP ( 'NONE', ( #22417, #20239, #1105, #19462 ) ) ;
#20607=CARTESIAN_POINT ( 'NONE',  ( 1.270000000000000018, -3695.699999999999818, 2240.279999999999745 ) ) ;
#20608=CARTESIAN_POINT ( 'NONE',  ( 10.88870223824514838, -3657.311324262453127, 2247.705266899251455 ) ) ;
#20610=CIRCLE ( 'NONE', #20258, 2.844800000000001550 ) ;
#20611=ORIENTED_EDGE ( 'NONE', *, *, #7960, .F. ) ;
#20612=VERTEX_POINT ( 'NONE', #15638 ) ;
#20614=EDGE_CURVE ( 'NONE', #13646, #8599, #21263, .T. ) ;
#20620=CARTESIAN_POINT ( 'NONE',  ( 141.5231090388281245, -3581.679082975166239, 2247.783365689513630 ) ) ;
#20621=VERTEX_POINT ( 'NONE', #15754 ) ;
#20622=DIRECTION ( 'NONE',  ( 0.000000000000000000, 0.000000000000000000, -1.000000000000000000 ) ) ;
#20624=CARTESIAN_POINT ( 'NONE',  ( 130.6067999999989979, -3619.500000000000000, 2239.771999999999935 ) ) ;
#20625=CARTESIAN_POINT ( 'NONE',  ( 20.71806297877481029, -3543.329302114565053, 2259.603420030892266 ) ) ;
#20626=CIRCLE ( 'NONE', #13901, 0.7619999999999294005 ) ;
#20627=FACE_OUTER_BOUND ( 'NONE', #9882, .T. ) ;
#20628=CIRCLE ( 'NONE', #10535, 0.7619999999999294005 ) ;
#20629=B_SPLINE_CURVE_WITH_KNOTS ( 'NONE', 3,
 ( #285, #2268, #3903, #14227, #1804, #14464 ),
 .UNSPECIFIED., .F., .F.,
 ( 4, 1, 1, 4 ),
 ( 0.000000000000000000, 0.3333333333333000081, 0.6666666666667000474, 1.000000000000000000 ),
 .UNSPECIFIED. ) ;
#20630=ORIENTED_EDGE ( 'NONE', *, *, #22517, .F. ) ;
#20632=VERTEX_POINT ( 'NONE', #22879 ) ;
#20634=CARTESIAN_POINT ( 'NONE',  ( 79.80679999999999552, -3670.300000000000182, 2239.771999999999935 ) ) ;
#20641=DIRECTION ( 'NONE',  ( 0.000000000000000000, 0.000000000000000000, -1.000000000000000000 ) ) ;
#20644=CARTESIAN_POINT ( 'NONE',  ( 114.2999999999999972, -3644.899999999999636, 2259.837999999999738 ) ) ;
#20649=CARTESIAN_POINT ( 'NONE',  ( 142.3397478532754405, -3658.444484825467953, 2249.676348100301766 ) ) ;
#20654=CARTESIAN_POINT ( 'NONE',  ( 136.8943284708507804, -3543.452888079240893, 2255.108476224739206 ) ) ;
#20657=ORIENTED_EDGE ( 'NONE', *, *, #10421, .T. ) ;
#20660=ADVANCED_FACE ( 'NONE', ( #8371 ), #3202, .F. ) ;
#20663=DIRECTION ( 'NONE',  ( 1.000000000000000000, 0.000000000000000000, 0.000000000000000000 ) ) ;
#20666=CIRCLE ( 'NONE', #1213, 5.714999999999970548 ) ;
#20668=EDGE_CURVE ( 'NONE', #3271, #16691, #3542, .T. ) ;
#20669=EDGE_LOOP ( 'NONE', ( #9259, #12060 ) ) ;
#20671=DIRECTION ( 'NONE',  ( 1.000000000000000000, 0.000000000000000000, 0.000000000000000000 ) ) ;
#20672=DIRECTION ( 'NONE',  ( 1.224646799147353207E-16, 1.000000000000000000, -0.000000000000000000 ) ) ;
#20673=AXIS2_PLACEMENT_3D ( 'NONE', #15183, #18921, #20796 ) ;
#20681=DIRECTION ( 'NONE',  ( 1.000000000000000000, 0.000000000000000000, 0.000000000000000000 ) ) ;
#20682=DIRECTION ( 'NONE',  ( 0.000000000000000000, -1.000000000000000000, 0.000000000000000000 ) ) ;
#20688=CARTESIAN_POINT ( 'NONE',  ( 144.7271686052660300, -3662.223246664079397, 2245.454731745688150 ) ) ;
#20689=B_SPLINE_CURVE_WITH_KNOTS ( 'NONE', 3,
 ( #10406, #8654, #19550, #22929, #6904, #21201, #19435, #8772, #29, #1785, #10687, #6637, #4747, #13531, #19596, #8264, #17158, #12008, #9889 ),
 .UNSPECIFIED., .F., .F.,
 ( 4, 2, 2, 1, 2, 2, 2, 2, 2, 4 ),
 ( 0.000000000000000000, 0.1250000000003315404, 0.1875000000007193135, 0.2187500000009131862, 0.2343750000008835155, 0.2500000000008538725, 0.3750000000007115419, 0.5000000000005692113, 0.7500000000002845502, 1.000000000000000000 ),
 .UNSPECIFIED. ) ;
#20690=VERTEX_POINT ( 'NONE', #10352 ) ;
#20693=CARTESIAN_POINT ( 'NONE',  ( 14.06056753155343308, -3662.003450156426425, 2249.541530534452249 ) ) ;
#20696=VERTEX_POINT ( 'NONE', #3438 ) ;
#20700=CARTESIAN_POINT ( 'NONE',  ( 133.9967742479666697, -3579.071087744469878, 2244.547217120886671 ) ) ;
#20701=CARTESIAN_POINT ( 'NONE',  ( 15.40608766543241082, -3658.626372987976538, 2249.801193023435189 ) ) ;
#20702=CARTESIAN_POINT ( 'NONE',  ( 114.2999999999999972, -3594.099999999999909, 2239.771999999999935 ) ) ;
#20703=VERTEX_POINT ( 'NONE', #11997 ) ;
#20705=EDGE_LOOP ( 'NONE', ( #13876, #14229, #14466, #15205 ) ) ;
#20708=CARTESIAN_POINT ( 'NONE',  ( 98.75520000000000209, -3568.700000000000273, 2259.837999999999738 ) ) ;
#20709=ORIENTED_EDGE ( 'NONE', *, *, #15407, .F. ) ;
#20715=CARTESIAN_POINT ( 'NONE',  ( 54.40679999999999694, -3568.700000000000273, 2260.600000000000364 ) ) ;
#20719=CARTESIAN_POINT ( 'NONE',  ( 137.8138258362651811, -3577.363333663654430, 2249.812340048487840 ) ) ;
#20720=EDGE_LOOP ( 'NONE', ( #8467, #8225, #12482, #2666 ) ) ;
#20721=CIRCLE ( 'NONE', #9506, 3.606799999999001027 ) ;
#20722=EDGE_CURVE ( 'NONE', #15342, #10158, #15524, .T. ) ;
#20726=CARTESIAN_POINT ( 'NONE',  ( 151.4000000000000057, -3660.140000000000327, 2247.392000000000280 ) ) ;
#20727=CARTESIAN_POINT ( 'NONE',  ( 10.81816717404539219, -3657.371485001214296, 2248.046767603714216 ) ) ;
#20728=EDGE_LOOP ( 'NONE', ( #19846, #17774, #20151, #17342 ) ) ;
#20730=LINE ( 'NONE', #11945, #15791 ) ;
#20732=ORIENTED_EDGE ( 'NONE', *, *, #559, .T. ) ;
#20733=EDGE_CURVE ( 'NONE', #17585, #3143, #20629, .T. ) ;
#20736=EDGE_CURVE ( 'NONE', #9068, #1906, #5431, .T. ) ;
#20737=DIRECTION ( 'NONE',  ( 0.000000000000000000, 0.000000000000000000, -1.000000000000000000 ) ) ;
#20740=CARTESIAN_POINT ( 'NONE',  ( 141.8047404989038682, -3581.408896080104114, 2248.655369336666809 ) ) ;
#20741=ORIENTED_EDGE ( 'NONE', *, *, #2364, .F. ) ;
#20746=AXIS2_PLACEMENT_3D ( 'NONE', #14727, #19643, #12621 ) ;
#20747=DIRECTION ( 'NONE',  ( 1.224646799147353207E-16, 1.000000000000000000, -0.000000000000000000 ) ) ;
#20748=CARTESIAN_POINT ( 'NONE',  ( 20.66921499434370091, -3543.363127659929887, 2259.725433999880352 ) ) ;
#20749=EDGE_CURVE ( 'NONE', #21667, #3669, #14780, .T. ) ;
#20750=DIRECTION ( 'NONE',  ( 0.000000000000000000, 0.000000000000000000, -1.000000000000000000 ) ) ;
#20754=EDGE_CURVE ( 'NONE', #15794, #10464, #15584, .T. ) ;
#20756=AXIS2_PLACEMENT_3D ( 'NONE', #22766, #1563, #1324 ) ;
#20757=CARTESIAN_POINT ( 'NONE',  ( 40.94480000000000075, -3594.099999999999909, 2261.869999999999891 ) ) ;
#20758=AXIS2_PLACEMENT_3D ( 'NONE', #18394, #22022, #13018 ) ;
#20762=ORIENTED_EDGE ( 'NONE', *, *, #8801, .T. ) ;
#20764=CARTESIAN_POINT ( 'NONE',  ( 127.0000000000000000, -3619.500000000000000, 2259.837999999999738 ) ) ;
#20769=CARTESIAN_POINT ( 'NONE',  ( 15.24000000000000021, -3694.430000000000291, 2255.774000000000342 ) ) ;
#20771=CARTESIAN_POINT ( 'NONE',  ( 6.996957829346665214, -3659.928346034561400, 2244.547218180292020 ) ) ;
#20772=CARTESIAN_POINT ( 'NONE',  ( 139.6999999999999886, -3659.504999999999654, 2272.030000000000200 ) ) ;
#20773=CARTESIAN_POINT ( 'NONE',  ( 88.90000000000000568, -3644.899999999999636, 2259.837999999999738 ) ) ;
#20776=CARTESIAN_POINT ( 'NONE',  ( 95.25000000000000000, -3670.300000000000182, 2250.236800000000130 ) ) ;
#20780=LINE ( 'NONE', #17144, #8114 ) ;
#20782=CARTESIAN_POINT ( 'NONE',  ( 4.878091718509972807, -3695.444958114254405, 2260.094543566995071 ) ) ;
#20784=EDGE_LOOP ( 'NONE', ( #16157, #19666, #20915, #22026 ) ) ;
#20786=CARTESIAN_POINT ( 'NONE',  ( 54.40679999999999694, -3670.300000000000182, 2239.009999999999764 ) ) ;
#20792=VECTOR ( 'NONE', #13008, 1000.000000000000000 ) ;
#20795=AXIS2_PLACEMENT_3D ( 'NONE', #3029, #3374, #17790 ) ;
#20796=DIRECTION ( 'NONE',  ( 1.000000000000000000, 0.000000000000000000, 0.000000000000000000 ) ) ;
#20798=CARTESIAN_POINT ( 'NONE',  ( 20.57350643676103630, -3695.530403268316604, 2259.964929154887614 ) ) ;
#20803=ORIENTED_EDGE ( 'NONE', *, *, #4852, .T. ) ;
#20806=CARTESIAN_POINT ( 'NONE',  ( 10.68286790803779773, -3581.501839941320668, 2248.451798419007901 ) ) ;
#20809=ADVANCED_FACE ( 'NONE', ( #19848 ), #14348, .F. ) ;
#20810=CIRCLE ( 'NONE', #608, 1.269999999999993356 ) ;
#20811=ORIENTED_EDGE ( 'NONE', *, *, #4359, .T. ) ;
#20813=FACE_BOUND ( 'NONE', #5237, .T. ) ;
#20815=AXIS2_PLACEMENT_3D ( 'NONE', #1216, #22773, #1452 ) ;
#20817=CARTESIAN_POINT ( 'NONE',  ( 144.5620013165544151, -3662.508668946073612, 2245.816465486211655 ) ) ;
#20821=LINE ( 'NONE', #6416, #1332 ) ;
#20833=TOROIDAL_SURFACE ( 'NONE', #2143, 4.114799999999999791, 1.270000000000000018 ) ;
#20834=ORIENTED_EDGE ( 'NONE', *, *, #6839, .F. ) ;
#20837=LINE ( 'NONE', #8886, #21793 ) ;
#20838=ORIENTED_EDGE ( 'NONE', *, *, #16559, .T. ) ;
#20839=ADVANCED_FACE ( 'NONE', ( #8951 ), #19642, .T. ) ;
#20842=EDGE_CURVE ( 'NONE', #14926, #16048, #3780, .T. ) ;
#20845=DIRECTION ( 'NONE',  ( 0.000000000000000000, 0.000000000000000000, 1.000000000000000000 ) ) ;
#20847=EDGE_LOOP ( 'NONE', ( #22497, #21810, #7771, #5394 ) ) ;
#20848=CIRCLE ( 'NONE', #5895, 3.606799999999001027 ) ;
#20850=CIRCLE ( 'NONE', #15619, 0.7619999999999294005 ) ;
#20852=ORIENTED_EDGE ( 'NONE', *, *, #16840, .T. ) ;
#20853=CARTESIAN_POINT ( 'NONE',  ( 147.8270794805000037, -3695.699999999999818, 2259.329999999999927 ) ) ;
#20859=EDGE_CURVE ( 'NONE', #13662, #13759, #22637, .T. ) ;
#20862=CARTESIAN_POINT ( 'NONE',  ( 10.50330237546534207, -3577.685423964297115, 2249.983956755341751 ) ) ;
#20865=VERTEX_POINT ( 'NONE', #8118 ) ;
#20866=CARTESIAN_POINT ( 'NONE',  ( 131.8858715492527267, -3695.429311327186497, 2260.113811941836957 ) ) ;
#20868=AXIS2_PLACEMENT_3D ( 'NONE', #148, #10688, #19829 ) ;
#20869=CYLINDRICAL_SURFACE ( 'NONE', #22721, 1.269999999999900098 ) ;
#20870=EDGE_CURVE ( 'NONE', #21361, #13997, #21899, .T. ) ;
#20871=CARTESIAN_POINT ( 'NONE',  ( 25.39999999999999858, -3619.500000000000000, 2239.009999999999764 ) ) ;
#20872=CIRCLE ( 'NONE', #8113, 0.7619999999999987894 ) ;
#20873=DIRECTION ( 'NONE',  ( 1.000000000000000000, 0.000000000000000000, 0.000000000000000000 ) ) ;
#20875=DIRECTION ( 'NONE',  ( 0.000000000000000000, 0.000000000000000000, 1.000000000000000000 ) ) ;
#20876=ADVANCED_FACE ( 'NONE', ( #7646 ), #18532, .T. ) ;
#20879=LINE ( 'NONE', #22184, #22249 ) ;
#20885=ORIENTED_EDGE ( 'NONE', *, *, #8058, .F. ) ;
#20889=EDGE_CURVE ( 'NONE', #11227, #22687, #17397, .T. ) ;
#20892=CARTESIAN_POINT ( 'NONE',  ( 137.7873330486999919, -3657.399152860999493, 2246.630000000000109 ) ) ;
#20895=CARTESIAN_POINT ( 'NONE',  ( 34.49320000000000164, -3644.899999999999636, 2239.771999999999935 ) ) ;
#20901=DIRECTION ( 'NONE',  ( 0.000000000000000000, 0.000000000000000000, -1.000000000000000000 ) ) ;
#20902=CARTESIAN_POINT ( 'NONE',  ( 141.8231898388004595, -3657.611600801285931, 2248.695890107555897 ) ) ;
#20904=CARTESIAN_POINT ( 'NONE',  ( 136.8581536596348087, -3543.408637599010035, 2255.017959195303774 ) ) ;
#20905=EDGE_CURVE ( 'NONE', #16978, #10242, #6019, .T. ) ;
#20907=ORIENTED_EDGE ( 'NONE', *, *, #11519, .F. ) ;
#20908=DIRECTION ( 'NONE',  ( 0.000000000000000000, 0.000000000000000000, 1.000000000000000000 ) ) ;
#20911=EDGE_LOOP ( 'NONE', ( #20521, #1250, #18062, #3732 ) ) ;
#20912=DIRECTION ( 'NONE',  ( -0.000000000000000000, 1.000000000000000000, -0.000000000000000000 ) ) ;
#20913=DIRECTION ( 'NONE',  ( 0.000000000000000000, 0.000000000000000000, -1.000000000000000000 ) ) ;
#20914=LINE ( 'NONE', #4851, #3595 ) ;
#20915=ORIENTED_EDGE ( 'NONE', *, *, #8439, .T. ) ;
#20919=CARTESIAN_POINT ( 'NONE',  ( 95.25000000000000000, -3670.300000000000182, 2247.392000000000280 ) ) ;
#20920=AXIS2_PLACEMENT_3D ( 'NONE', #9695, #11337, #681 ) ;
#20921=CARTESIAN_POINT ( 'NONE',  ( 92.50679999999999836, -3594.099999999999909, 2239.009999999999764 ) ) ;
#20922=EDGE_LOOP ( 'NONE', ( #8411, #19467, #12586, #5274 ) ) ;
#20924=EDGE_LOOP ( 'NONE', ( #8250, #14635, #342, #22800 ) ) ;
#20925=CARTESIAN_POINT ( 'NONE',  ( 35.56000000000000227, -3694.430000000000291, 2247.392000000000280 ) ) ;
#20926=CARTESIAN_POINT ( 'NONE',  ( 10.89166860073782672, -3581.691115089716277, 2247.681511753725317 ) ) ;
#20927=VERTEX_POINT ( 'NONE', #4134 ) ;
#20930=DIRECTION ( 'NONE',  ( 1.224646799147353207E-16, 1.000000000000000000, -0.000000000000000000 ) ) ;
#20931=AXIS2_PLACEMENT_3D ( 'NONE', #16117, #15658, #67 ) ;
#20933=CARTESIAN_POINT ( 'NONE',  ( 145.2053555853632361, -3661.038792355501755, 2244.692860678725083 ) ) ;
#20935=CARTESIAN_POINT ( 'NONE',  ( 12.69999999999999929, -3659.504999999999654, 2239.009999999999764 ) ) ;
#20936=CARTESIAN_POINT ( 'NONE',  ( 11.49452485132638380, -3662.081945281043318, 2249.471023377334859 ) ) ;
#20938=CARTESIAN_POINT ( 'NONE',  ( 147.4512313346230314, -3543.717426572050044, 2260.271352724699227 ) ) ;
#20939=VERTEX_POINT ( 'NONE', #18762 ) ;
#20940=DIRECTION ( 'NONE',  ( -1.000000000000000000, 0.000000000000000000, 0.000000000000000000 ) ) ;
#20941=DIRECTION ( 'NONE',  ( -1.000000000000000000, 0.000000000000000000, 0.000000000000000000 ) ) ;
#20944=CARTESIAN_POINT ( 'NONE',  ( 15.10427522816852530, -3657.984367098621988, 2249.248490382821274 ) ) ;
#20946=ORIENTED_EDGE ( 'NONE', *, *, #13211, .T. ) ;
#20947=VECTOR ( 'NONE', #6926, 1000.000000000000000 ) ;
#20959=CARTESIAN_POINT ( 'NONE',  ( 127.0000000000000000, -3670.300000000000182, 2239.771999999999935 ) ) ;
#20960=ORIENTED_EDGE ( 'NONE', *, *, #9833, .F. ) ;
#20963=LINE ( 'NONE', #3493, #2452 ) ;
#20964=VERTEX_POINT ( 'NONE', #951 ) ;
#20967=CARTESIAN_POINT ( 'NONE',  ( 147.3199999999999932, -3694.430000000000291, 2260.600000000000364 ) ) ;
#20972=CARTESIAN_POINT ( 'NONE',  ( 114.2999999999999972, -3594.099999999999909, 2239.009999999999764 ) ) ;
#20974=ORIENTED_EDGE ( 'NONE', *, *, #3677, .T. ) ;
#20977=LINE ( 'NONE', #8561, #8519 ) ;
#20979=CARTESIAN_POINT ( 'NONE',  ( 1.270000000000000018, -3694.430000000000291, 2239.009999999999764 ) ) ;
#20984=CARTESIAN_POINT ( 'NONE',  ( 53.64479999999999649, -3670.300000000000182, 2239.771999999999935 ) ) ;
#20986=CARTESIAN_POINT ( 'NONE',  ( 14.64183135348199194, -3581.574010930764416, 2248.245069266252358 ) ) ;
#20988=CARTESIAN_POINT ( 'NONE',  ( 134.1794544657873018, -3658.026865190803619, 2245.487007817819176 ) ) ;
#20989=ADVANCED_FACE ( 'NONE', ( #11609 ), #7323, .T. ) ;
#20990=DIRECTION ( 'NONE',  ( 1.000000000000000000, 0.000000000000000000, 0.000000000000000000 ) ) ;
#20992=CYLINDRICAL_SURFACE ( 'NONE', #14442, 2.844800000000091700 ) ;
#20993=AXIS2_PLACEMENT_3D ( 'NONE', #9333, #18457, #5478 ) ;
#20994=DIRECTION ( 'NONE',  ( -1.000000000000000000, -4.815138086611999802E-14, 0.000000000000000000 ) ) ;
#20996=DIRECTION ( 'NONE',  ( -1.000000000000000000, 0.000000000000000000, 0.000000000000000000 ) ) ;
#20997=DIRECTION ( 'NONE',  ( 0.000000000000000000, 0.000000000000000000, 1.000000000000000000 ) ) ;
#21001=DIRECTION ( 'NONE',  ( 1.000000000000000000, 0.000000000000000000, 0.000000000000000000 ) ) ;
#21005=FACE_OUTER_BOUND ( 'NONE', #17668, .T. ) ;
#21008=CYLINDRICAL_SURFACE ( 'NONE', #2725, 2.844800000000091700 ) ;
#21009=AXIS2_PLACEMENT_3D ( 'NONE', #21733, #21282, #19863 ) ;
#21010=DIRECTION ( 'NONE',  ( 0.000000000000000000, 0.000000000000000000, 1.000000000000000000 ) ) ;
#21012=EDGE_CURVE ( 'NONE', #10683, #6818, #22264, .T. ) ;
#21013=VECTOR ( 'NONE', #8120, 1000.000000000000000 ) ;
#21014=EDGE_CURVE ( 'NONE', #10931, #21665, #15540, .T. ) ;
#21015=DIRECTION ( 'NONE',  ( 0.000000000000000000, 0.000000000000000000, 1.000000000000000000 ) ) ;
#21017=DIRECTION ( 'NONE',  ( 1.000000000000000000, 0.000000000000000000, -1.224646799147353207E-16 ) ) ;
#21018=CARTESIAN_POINT ( 'NONE',  ( 142.0776493914862897, -3657.942898745972343, 2249.199396469671228 ) ) ;
#21019=ADVANCED_FACE ( 'NONE', ( #723 ), #8044, .T. ) ;
#21020=ORIENTED_EDGE ( 'NONE', *, *, #13235, .T. ) ;
#21022=ORIENTED_EDGE ( 'NONE', *, *, #21947, .T. ) ;
#21025=EDGE_CURVE ( 'NONE', #16346, #279, #21157, .T. ) ;
#21030=CARTESIAN_POINT ( 'NONE',  ( 4.658066890921409353, -3543.315017898367387, 2259.542481502586270 ) ) ;
#21031=CARTESIAN_POINT ( 'NONE',  ( 151.1299999999999955, -3695.699999999999818, 2240.279999999999745 ) ) ;
#21032=DIRECTION ( 'NONE',  ( 1.224646799147353207E-16, 1.000000000000000000, -0.000000000000000000 ) ) ;
#21033=ORIENTED_EDGE ( 'NONE', *, *, #18244, .T. ) ;
#21037=CARTESIAN_POINT ( 'NONE',  ( 10.78723565514999905, -3581.600816721000228, 2246.630000000000109 ) ) ;
#21038=AXIS2_PLACEMENT_3D ( 'NONE', #181, #16347, #14248 ) ;
#21044=VECTOR ( 'NONE', #14985, 1000.000000000000000 ) ;
#21046=CARTESIAN_POINT ( 'NONE',  ( 0.000000000000000000, -3544.570000000000164, 2259.329999999999927 ) ) ;
#21048=DIRECTION ( 'NONE',  ( -1.000000000000000000, 0.000000000000000000, 0.000000000000000000 ) ) ;
#21049=ORIENTED_EDGE ( 'NONE', *, *, #8678, .F. ) ;
#21050=FACE_BOUND ( 'NONE', #3352, .T. ) ;
#21052=CARTESIAN_POINT ( 'NONE',  ( 144.3113860274000047, -3662.880847139000252, 2246.630000000000109 ) ) ;
#21057=CARTESIAN_POINT ( 'NONE',  ( 12.01160536040741711, -3662.265695842842433, 2249.282711244598886 ) ) ;
#21059=ORIENTED_EDGE ( 'NONE', *, *, #1235, .T. ) ;
#21061=VECTOR ( 'NONE', #17378, 1000.000000000000000 ) ;
#21062=DIRECTION ( 'NONE',  ( -1.224646799147353207E-16, 1.000000000000000000, 0.000000000000000000 ) ) ;
#21068=CARTESIAN_POINT ( 'NONE',  ( 15.54479999999999862, -3659.504999999999654, 2272.030000000000200 ) ) ;
#21069=VERTEX_POINT ( 'NONE', #13849 ) ;
#21070=CARTESIAN_POINT ( 'NONE',  ( 9.842728535705985493, -3543.392327578453205, 2254.979487868655269 ) ) ;
#21073=FACE_OUTER_BOUND ( 'NONE', #13609, .T. ) ;
#21074=CARTESIAN_POINT ( 'NONE',  ( 101.5999999999999943, -3619.500000000000000, 2260.600000000000364 ) ) ;
#21076=CIRCLE ( 'NONE', #16942, 0.7619999999999294005 ) ;
#21082=DIRECTION ( 'NONE',  ( -1.000000000000000000, 0.000000000000000000, 0.000000000000000000 ) ) ;
#21088=CARTESIAN_POINT ( 'NONE',  ( 9.855099624826999971, -3659.505002774999411, 2250.165042250000170 ) ) ;
#21090=VERTEX_POINT ( 'NONE', #21116 ) ;
#21091=CARTESIAN_POINT ( 'NONE',  ( 134.2981814352962999, -3581.361247027981335, 2246.035952059839019 ) ) ;
#21093=ORIENTED_EDGE ( 'NONE', *, *, #3770, .T. ) ;
#21097=CARTESIAN_POINT ( 'NONE',  ( 1.270000000000000018, -3695.699999999999818, 2240.279999999999745 ) ) ;
#21098=VERTEX_POINT ( 'NONE', #5060 ) ;
#21099=CARTESIAN_POINT ( 'NONE',  ( 131.5729205195000020, -3695.699999999999818, 2259.329999999999927 ) ) ;
#21104=VECTOR ( 'NONE', #14332, 1000.000000000000000 ) ;
#21105=CARTESIAN_POINT ( 'NONE',  ( 134.1374959654496308, -3658.193646307140625, 2245.317243222136312 ) ) ;
#21107=EDGE_CURVE ( 'NONE', #12370, #19652, #4680, .T. ) ;
#21108=DIRECTION ( 'NONE',  ( 0.000000000000000000, 0.000000000000000000, -1.000000000000000000 ) ) ;
#21111=ADVANCED_FACE ( 'NONE', ( #8346 ), #6571, .T. ) ;
#21112=ORIENTED_EDGE ( 'NONE', *, *, #19476, .T. ) ;
#21114=VERTEX_POINT ( 'NONE', #6942 ) ;
#21115=CARTESIAN_POINT ( 'NONE',  ( 38.10000000000000142, -3594.099999999999909, 2261.869999999999891 ) ) ;
#21116=CARTESIAN_POINT ( 'NONE',  ( 105.2067999999999870, -3670.300000000000182, 2239.009999999999764 ) ) ;
#21117=ORIENTED_EDGE ( 'NONE', *, *, #9825, .T. ) ;
#21124=CARTESIAN_POINT ( 'NONE',  ( 139.6999999999999886, -3579.494999999999891, 2246.630000000000109 ) ) ;
#21125=MANIFOLD_SOLID_BREP ( 'SOLID2-16[1]', #139 ) ;
#21126=( LENGTH_UNIT ( ) NAMED_UNIT ( * ) SI_UNIT ( .MILLI., .METRE. ) );
#21129=FACE_OUTER_BOUND ( 'NONE', #20924, .T. ) ;
#21134=CARTESIAN_POINT ( 'NONE',  ( 141.5613417780174927, -3657.352510518997406, 2246.797770067877991 ) ) ;
#21136=ORIENTED_EDGE ( 'NONE', *, *, #7221, .T. ) ;
#21142=ORIENTED_EDGE ( 'NONE', *, *, #4933, .F. ) ;
#21144=ORIENTED_EDGE ( 'NONE', *, *, #14855, .T. ) ;
#21145=ORIENTED_EDGE ( 'NONE', *, *, #4489, .F. ) ;
#21146=CARTESIAN_POINT ( 'NONE',  ( 57.14999999999999858, -3695.699999999999818, 2247.392000000000280 ) ) ;
#21149=CARTESIAN_POINT ( 'NONE',  ( 4.767653496878255126, -3543.397347668057137, 2259.817636094936915 ) ) ;
#21153=VERTEX_POINT ( 'NONE', #9976 ) ;
#21155=FACE_BOUND ( 'NONE', #12131, .T. ) ;
#21157=CIRCLE ( 'NONE', #15175, 2.844799999998995244 ) ;
#21158=VECTOR ( 'NONE', #10733, 1000.000000000000000 ) ;
#21159=ORIENTED_EDGE ( 'NONE', *, *, #6869, .F. ) ;
#21161=CIRCLE ( 'NONE', #16284, 3.606800000000000228 ) ;
#21163=CIRCLE ( 'NONE', #17786, 0.7619999999999294005 ) ;
#21165=CARTESIAN_POINT ( 'NONE',  ( 10.43004745555305846, -3581.209769231029895, 2248.995792276846714 ) ) ;
#21166=CARTESIAN_POINT ( 'NONE',  ( 127.0000000000000000, -3568.700000000000273, 2239.009999999999764 ) ) ;
#21168=DIRECTION ( 'NONE',  ( 0.000000000000000000, 0.000000000000000000, 1.000000000000000000 ) ) ;
#21169=CIRCLE ( 'NONE', #7694, 3.606799999998994366 ) ;
#21172=B_SPLINE_CURVE_WITH_KNOTS ( 'NONE', 3,
 ( #10332, #19242, #1181, #12091, #17588, #3179, #17475, #22748, #4943, #6605 ),
 .UNSPECIFIED., .F., .F.,
 ( 4, 2, 1, 1, 2, 4 ),
 ( 0.000000000000000000, 0.06249999999947680740, 0.1249999999989536148, 0.2500000000000294209, 0.5000000000000967004, 1.000000000000000000 ),
 .UNSPECIFIED. ) ;
#21174=CIRCLE ( 'NONE', #10303, 1.269999999999882334 ) ;
#21175=CARTESIAN_POINT ( 'NONE',  ( 10.87509742458831319, -3661.689672940328819, 2249.779197371474766 ) ) ;
#21177=ADVANCED_FACE ( 'NONE', ( #22622 ), #14044, .T. ) ;
#21179=DIRECTION ( 'NONE',  ( 0.000000000000000000, 0.000000000000000000, -1.000000000000000000 ) ) ;
#21180=AXIS2_PLACEMENT_3D ( 'NONE', #15227, #22358, #17550 ) ;
#21181=ORIENTED_EDGE ( 'NONE', *, *, #10817, .T. ) ;
#21186=CARTESIAN_POINT ( 'NONE',  ( 15.08810205602369514, -3657.959134956293383, 2249.218684437550110 ) ) ;
#21187=CARTESIAN_POINT ( 'NONE',  ( 15.52167594717750809, -3579.072456535235233, 2250.236800948000109 ) ) ;
#21188=VERTEX_POINT ( 'NONE', #8922 ) ;
#21191=DIRECTION ( 'NONE',  ( 0.000000000000000000, -1.000000000000000000, 1.319970543219000025E-14 ) ) ;
#21199=CIRCLE ( 'NONE', #4725, 2.844799999999994444 ) ;
#21200=DIRECTION ( 'NONE',  ( -1.000000000000000000, 0.000000000000000000, 0.000000000000000000 ) ) ;
#21201=CARTESIAN_POINT ( 'NONE',  ( 17.49835313622208233, -3576.390213567464798, 2245.979654398315688 ) ) ;
#21203=CIRCLE ( 'NONE', #5870, 2.844799999999994444 ) ;
#21206=CARTESIAN_POINT ( 'NONE',  ( 25.39999999999999858, -3670.300000000000182, 2260.600000000000364 ) ) ;
#21207=ADVANCED_FACE ( 'NONE', ( #7062 ), #8804, .T. ) ;
#21209=DIRECTION ( 'NONE',  ( 0.000000000000000000, 0.000000000000000000, -1.000000000000000000 ) ) ;
#21210=ORIENTED_EDGE ( 'NONE', *, *, #14817, .F. ) ;
#21211=CARTESIAN_POINT ( 'NONE',  ( 21.79320000000099711, -3670.300000000000182, 2239.009999999999764 ) ) ;
#21214=CARTESIAN_POINT ( 'NONE',  ( 134.2546079315347356, -3581.231065619790115, 2245.814675045431159 ) ) ;
#21215=ORIENTED_EDGE ( 'NONE', *, *, #11232, .T. ) ;
#21223=DIRECTION ( 'NONE',  ( -1.000000000000000000, 0.000000000000000000, 0.000000000000000000 ) ) ;
#21224=CARTESIAN_POINT ( 'NONE',  ( 15.01285743453679267, -3581.153169946162961, 2249.079238002240345 ) ) ;
#21225=VECTOR ( 'NONE', #11719, 1000.000000000000000 ) ;
#21227=DIRECTION ( 'NONE',  ( 0.000000000000000000, -1.000000000000000000, 0.000000000000000000 ) ) ;
#21228=AXIS2_PLACEMENT_3D ( 'NONE', #13623, #17131, #11740 ) ;
#21229=DIRECTION ( 'NONE',  ( 0.000000000000000000, 0.000000000000000000, 1.000000000000000000 ) ) ;
#21231=CARTESIAN_POINT ( 'NONE',  ( 79.80679999999999552, -3568.700000000000273, 2239.009999999999764 ) ) ;
#21233=DIRECTION ( 'NONE',  ( 1.000000000000000000, 0.000000000000000000, 0.000000000000000000 ) ) ;
#21234=ORIENTED_EDGE ( 'NONE', *, *, #21561, .T. ) ;
#21240=DIRECTION ( 'NONE',  ( 0.000000000000000000, 0.000000000000000000, -1.000000000000000000 ) ) ;
#21241=CARTESIAN_POINT ( 'NONE',  ( 139.6999999999999886, -3579.494999999999891, 2239.771999999999935 ) ) ;
#21243=CIRCLE ( 'NONE', #6661, 0.7619999999999294005 ) ;
#21245=CARTESIAN_POINT ( 'NONE',  ( 15.47880416110802670, -3660.114175108592917, 2250.236712862199965 ) ) ;
#21247=CARTESIAN_POINT ( 'NONE',  ( 136.8551999999999964, -3579.495007806000103, 2250.165025852999861 ) ) ;
#21250=AXIS2_PLACEMENT_3D ( 'NONE', #16261, #3259, #3718 ) ;
#21251=AXIS2_PLACEMENT_3D ( 'NONE', #20624, #15710, #940 ) ;
#21254=CARTESIAN_POINT ( 'NONE',  ( 137.5852380282969136, -3657.602178072644620, 2248.677473072372322 ) ) ;
#21255=ORIENTED_EDGE ( 'NONE', *, *, #12439, .T. ) ;
#21256=DIRECTION ( 'NONE',  ( 0.000000000000000000, 1.000000000000000000, 0.000000000000000000 ) ) ;
#21259=VERTEX_POINT ( 'NONE', #4191 ) ;
#21260=ORIENTED_EDGE ( 'NONE', *, *, #3256, .T. ) ;
#21263=LINE ( 'NONE', #19495, #7720 ) ;
#21264=ORIENTED_EDGE ( 'NONE', *, *, #9516, .F. ) ;
#21269=ORIENTED_EDGE ( 'NONE', *, *, #20870, .F. ) ;
#21270=DIRECTION ( 'NONE',  ( -1.000000000000000000, 0.000000000000000000, 0.000000000000000000 ) ) ;
#21277=ORIENTED_EDGE ( 'NONE', *, *, #7436, .F. ) ;
#21279=EDGE_CURVE ( 'NONE', #16839, #8573, #17799, .T. ) ;
#21282=DIRECTION ( 'NONE',  ( 0.000000000000000000, 0.000000000000000000, -1.000000000000000000 ) ) ;
#21283=CARTESIAN_POINT ( 'NONE',  ( 10.29510451277807093, -3581.014576728029624, 2249.249714666130330 ) ) ;
#21285=CARTESIAN_POINT ( 'NONE',  ( 151.1299999999999955, -3578.860000000000127, 2247.392000000000280 ) ) ;
#21286=ADVANCED_FACE ( 'NONE', ( #12437 ), #18370, .T. ) ;
#21288=FACE_BOUND ( 'NONE', #13387, .T. ) ;
#21293=CARTESIAN_POINT ( 'NONE',  ( 10.67302639621317795, -3661.501522125889096, 2249.890123210526326 ) ) ;
#21295=CARTESIAN_POINT ( 'NONE',  ( 15.54478936534684941, -3659.505023738319323, 2250.165136749944850 ) ) ;
#21299=LINE ( 'NONE', #7011, #1853 ) ;
#21300=CARTESIAN_POINT ( 'NONE',  ( 15.34531583769129526, -3658.458524271727129, 2249.686710455694993 ) ) ;
#21301=CARTESIAN_POINT ( 'NONE',  ( 137.0372536546044842, -3695.258941568228238, 2255.466568422051296 ) ) ;
#21303=DIRECTION ( 'NONE',  ( 1.073225997510925892E-13, 0.000000000000000000, 1.000000000000000000 ) ) ;
#21304=ORIENTED_EDGE ( 'NONE', *, *, #18994, .T. ) ;
#21305=EDGE_CURVE ( 'NONE', #6861, #21259, #10695, .T. ) ;
#21309=ADVANCED_FACE ( 'NONE', ( #3521 ), #10678, .F. ) ;
#21310=CARTESIAN_POINT ( 'NONE',  ( 18.01287425285000410, -3657.399152860999493, 2246.630000000000109 ) ) ;
#21312=FACE_OUTER_BOUND ( 'NONE', #127, .T. ) ;
#21315=DIRECTION ( 'NONE',  ( 0.000000000000000000, 0.000000000000000000, 1.000000000000000000 ) ) ;
#21317=CARTESIAN_POINT ( 'NONE',  ( 21.79320000000099711, -3619.500000000000000, 2239.771999999999935 ) ) ;
#21318=EDGE_CURVE ( 'NONE', #1510, #18991, #17813, .T. ) ;
#21319=ORIENTED_EDGE ( 'NONE', *, *, #6012, .F. ) ;
#21322=ORIENTED_EDGE ( 'NONE', *, *, #818, .T. ) ;
#21324=EDGE_CURVE ( 'NONE', #10158, #6778, #22280, .T. ) ;
#21327=AXIS2_PLACEMENT_3D ( 'NONE', #3326, #12247, #17742 ) ;
#21328=ORIENTED_EDGE ( 'NONE', *, *, #5737, .T. ) ;
#21329=ORIENTED_EDGE ( 'NONE', *, *, #20614, .F. ) ;
#21335=CYLINDRICAL_SURFACE ( 'NONE', #22430, 1.269999999999882334 ) ;
#21336=CARTESIAN_POINT ( 'NONE',  ( 14.85086632574098964, -3581.357178777328954, 2248.755707450937734 ) ) ;
#21337=AXIS2_PLACEMENT_3D ( 'NONE', #10779, #5278, #1872 ) ;
#21338=DIRECTION ( 'NONE',  ( -1.000000000000000000, 0.000000000000000000, 0.000000000000000000 ) ) ;
#21343=SPHERICAL_SURFACE ( 'NONE', #4326, 1.270000000000000018 ) ;
#21344=FACE_OUTER_BOUND ( 'NONE', #11178, .T. ) ;
#21347=DIRECTION ( 'NONE',  ( 0.000000000000000000, 0.000000000000000000, -1.000000000000000000 ) ) ;
#21350=CARTESIAN_POINT ( 'NONE',  ( 20.31206600733000300, -3544.241663918999620, 2260.533847755999886 ) ) ;
#21351=VERTEX_POINT ( 'NONE', #3006 ) ;
#21354=AXIS2_PLACEMENT_3D ( 'NONE', #6901, #1738, #3484 ) ;
#21355=ORIENTED_EDGE ( 'NONE', *, *, #21839, .T. ) ;
#21356=CARTESIAN_POINT ( 'NONE',  ( 9.855200000000998273, -3659.504999999999654, 2256.063560000000052 ) ) ;
#21361=VERTEX_POINT ( 'NONE', #2551 ) ;
#21364=DIRECTION ( 'NONE',  ( -1.000000000000000000, 0.000000000000000000, 0.000000000000000000 ) ) ;
#21366=DIRECTION ( 'NONE',  ( 0.000000000000000000, -1.000000000000000000, 0.000000000000000000 ) ) ;
#21369=ORIENTED_EDGE ( 'NONE', *, *, #2078, .T. ) ;
#21370=ORIENTED_EDGE ( 'NONE', *, *, #3846, .T. ) ;
#21373=ORIENTED_EDGE ( 'NONE', *, *, #13086, .F. ) ;
#21376=EDGE_LOOP ( 'NONE', ( #11448, #11254, #15300, #4099 ) ) ;
#21380=ADVANCED_BREP_SHAPE_REPRESENTATION ( '', ( #21125, #5611 ), #2239 ) ;
#21383=CIRCLE ( 'NONE', #11273, 1.240967364599221412 ) ;
#21385=DIRECTION ( 'NONE',  ( 0.000000000000000000, 0.000000000000000000, -1.000000000000000000 ) ) ;
#21386=DIRECTION ( 'NONE',  ( 1.000000000000000000, 0.000000000000000000, 0.000000000000000000 ) ) ;
#21387=DIRECTION ( 'NONE',  ( 1.073225997510925892E-13, 0.000000000000000000, 1.000000000000000000 ) ) ;
#21390=CYLINDRICAL_SURFACE ( 'NONE', #16535, 1.269999999999898099 ) ;
#21397=FACE_BOUND ( 'NONE', #18473, .T. ) ;
#21399=EDGE_CURVE ( 'NONE', #13234, #17172, #21169, .T. ) ;
#21403=B_SPLINE_CURVE_WITH_KNOTS ( 'NONE', 3,
 ( #13196, #9350, #4069, #16487, #5731, #11439, #20353, #3955, #13089, #20240, #18591, #9238, #11324, #18474, #16717, #16824, #669 ),
 .UNSPECIFIED., .F., .F.,
 ( 4, 2, 2, 1, 2, 2, 2, 2, 4 ),
 ( 0.000000000000000000, 0.1249999999998916422, 0.1875000000000623945, 0.2187500000002796374, 0.2343750000001848244, 0.2500000000000900391, 0.5000000000000599520, 0.7500000000000299760, 1.000000000000000000 ),
 .UNSPECIFIED. ) ;
#21405=DIRECTION ( 'NONE',  ( 1.000000000000000000, 0.000000000000000000, 0.000000000000000000 ) ) ;
#21408=VERTEX_POINT ( 'NONE', #8405 ) ;
#21409=DIRECTION ( 'NONE',  ( -1.000000000000000000, 0.000000000000000000, 0.000000000000000000 ) ) ;
#21410=DIRECTION ( 'NONE',  ( -1.000000000000000000, 0.000000000000000000, 0.000000000000000000 ) ) ;
#21411=LINE ( 'NONE', #7349, #19059 ) ;
#21412=CARTESIAN_POINT ( 'NONE',  ( 14.62318399493629784, -3657.408672365483653, 2248.187748315331646 ) ) ;
#21414=CARTESIAN_POINT ( 'NONE',  ( 136.8552720942020073, -3695.594480551561446, 2255.010851275907498 ) ) ;
#21415=AXIS2_PLACEMENT_3D ( 'NONE', #4038, #18327, #9429 ) ;
#21416=CARTESIAN_POINT ( 'NONE',  ( 10.10523630290581565, -3578.289363367462556, 2250.192408352016173 ) ) ;
#21422=FACE_OUTER_BOUND ( 'NONE', #21816, .T. ) ;
#21428=PLANE ( 'NONE',  #162 ) ;
#21432=ADVANCED_FACE ( 'NONE', ( #11452, #781, #7945 ), #22218, .F. ) ;
#21437=ORIENTED_EDGE ( 'NONE', *, *, #14118, .T. ) ;
#21438=CARTESIAN_POINT ( 'NONE',  ( 142.2881911273701689, -3694.976217802131487, 2255.653223149227415 ) ) ;
#21439=FACE_OUTER_BOUND ( 'NONE', #22801, .T. ) ;
#21441=ORIENTED_EDGE ( 'NONE', *, *, #988, .F. ) ;
#21443=CARTESIAN_POINT ( 'NONE',  ( 137.2439122574247108, -3580.930587627222394, 2249.343187823710650 ) ) ;
#21444=EDGE_LOOP ( 'NONE', ( #8698, #9307 ) ) ;
#21445=CIRCLE ( 'NONE', #20673, 3.606799999999993567 ) ;
#21449=CARTESIAN_POINT ( 'NONE',  ( 12.69999999999999929, -3659.504999999999654, 2255.774000000000342 ) ) ;
#21450=CARTESIAN_POINT ( 'NONE',  ( 0.000000000000000000, -3578.860000000000127, 2247.392000000000280 ) ) ;
#21452=DIRECTION ( 'NONE',  ( 0.000000000000000000, -1.000000000000000000, 0.000000000000000000 ) ) ;
#21453=CARTESIAN_POINT ( 'NONE',  ( 1.270000000000000018, -3578.860000000000127, 2247.392000000000280 ) ) ;
#21455=CARTESIAN_POINT ( 'NONE',  ( 134.0275598363577103, -3578.798113836681750, 2244.547775376694972 ) ) ;
#21456=DIRECTION ( 'NONE',  ( 0.000000000000000000, 0.000000000000000000, 1.000000000000000000 ) ) ;
#21457=ORIENTED_EDGE ( 'NONE', *, *, #7657, .F. ) ;
#21460=AXIS2_PLACEMENT_3D ( 'NONE', #14241, #17508, #21386 ) ;
#21465=ORIENTED_EDGE ( 'NONE', *, *, #19286, .F. ) ;
#21467=CARTESIAN_POINT ( 'NONE',  ( 29.00679999999900005, -3619.500000000000000, 2259.837999999999738 ) ) ;
#21469=ORIENTED_EDGE ( 'NONE', *, *, #12816, .F. ) ;
#21470=DIRECTION ( 'NONE',  ( 0.000000000000000000, 0.000000000000000000, 1.000000000000000000 ) ) ;
#21473=DIRECTION ( 'NONE',  ( -0.000000000000000000, 1.000000000000000000, 0.000000000000000000 ) ) ;
#21474=ADVANCED_FACE ( 'NONE', ( #17530 ), #9210, .T. ) ;
#21478=EDGE_LOOP ( 'NONE', ( #8737, #20481, #20306, #18565 ) ) ;
#21481=ORIENTED_EDGE ( 'NONE', *, *, #14817, .T. ) ;
#21483=EDGE_CURVE ( 'NONE', #22588, #13787, #14454, .T. ) ;
#21484=CARTESIAN_POINT ( 'NONE',  ( 137.2895610191548599, -3657.994247822125999, 2249.259792710935926 ) ) ;
#21486=ORIENTED_EDGE ( 'NONE', *, *, #13517, .F. ) ;
#21490=VERTEX_POINT ( 'NONE', #5358 ) ;
#21491=ORIENTED_EDGE ( 'NONE', *, *, #13378, .F. ) ;
#21493=DIRECTION ( 'NONE',  ( 0.000000000000000000, -1.000000000000000000, 0.000000000000000000 ) ) ;
#21494=AXIS2_PLACEMENT_3D ( 'NONE', #18001, #1950, #19882 ) ;
#21495=ORIENTED_EDGE ( 'NONE', *, *, #1034, .T. ) ;
#21496=ORIENTED_EDGE ( 'NONE', *, *, #20599, .T. ) ;
#21497=FACE_OUTER_BOUND ( 'NONE', #13683, .T. ) ;
#21499=DIRECTION ( 'NONE',  ( 0.000000000000000000, 0.000000000000000000, -1.000000000000000000 ) ) ;
#21501=ORIENTED_EDGE ( 'NONE', *, *, #402, .F. ) ;
#21507=ORIENTED_EDGE ( 'NONE', *, *, #9652, .T. ) ;
#21508=CARTESIAN_POINT ( 'NONE',  ( 148.1947118165999768, -3544.570000000000164, 2259.679250718999810 ) ) ;
#21509=CIRCLE ( 'NONE', #11028, 5.715000000000999947 ) ;
#21512=FACE_OUTER_BOUND ( 'NONE', #14316, .T. ) ;
#21516=DIRECTION ( 'NONE',  ( 1.000000000000000000, 0.000000000000000000, 0.000000000000000000 ) ) ;
#21517=CARTESIAN_POINT ( 'NONE',  ( 9.855200000000998273, -3579.494999999999891, 2256.063560000000052 ) ) ;
#21518=DIRECTION ( 'NONE',  ( 0.000000000000000000, 0.000000000000000000, -1.000000000000000000 ) ) ;
#21520=DIRECTION ( 'NONE',  ( -1.000000000000000000, 0.000000000000000000, 0.000000000000000000 ) ) ;
#21522=CARTESIAN_POINT ( 'NONE',  ( 38.10000000000000142, -3644.899999999999636, 2239.771999999999935 ) ) ;
#21523=AXIS2_PLACEMENT_3D ( 'NONE', #10706, #18083, #16438 ) ;
#21525=AXIS2_PLACEMENT_3D ( 'NONE', #12320, #14661, #11248 ) ;
#21528=DIRECTION ( 'NONE',  ( 0.000000000000000000, -1.000000000000000000, 0.000000000000000000 ) ) ;
#21529=CIRCLE ( 'NONE', #1676, 3.606799999999993567 ) ;
#21530=CARTESIAN_POINT ( 'NONE',  ( 142.2650958631953699, -3544.173420540363168, 2255.711176449677623 ) ) ;
#21533=CARTESIAN_POINT ( 'NONE',  ( 7.263164726804554050, -3577.728755824955442, 2244.777032313797463 ) ) ;
#21537=EDGE_CURVE ( 'NONE', #10186, #22006, #945, .T. ) ;
#21538=CARTESIAN_POINT ( 'NONE',  ( 10.11273377225878889, -3543.933445092538022, 2255.655515828512762 ) ) ;
#21543=DIRECTION ( 'NONE',  ( 0.000000000000000000, 1.000000000000000000, 0.000000000000000000 ) ) ;
#21545=DIRECTION ( 'NONE',  ( 0.000000000000000000, 0.000000000000000000, -1.000000000000000000 ) ) ;
#21546=AXIS2_PLACEMENT_3D ( 'NONE', #16274, #7373, #14525 ) ;
#21550=CARTESIAN_POINT ( 'NONE',  ( 35.56000000000000227, -3544.570000000000164, 2247.392000000000280 ) ) ;
#21553=CARTESIAN_POINT ( 'NONE',  ( 151.1299999999999955, -3544.570000000000164, 2259.329999999999927 ) ) ;
#21557=AXIS2_PLACEMENT_3D ( 'NONE', #19589, #14977, #20 ) ;
#21558=AXIS2_PLACEMENT_3D ( 'NONE', #2321, #560, #7709 ) ;
#21560=CIRCLE ( 'NONE', #8088, 1.269999999999882334 ) ;
#21561=EDGE_CURVE ( 'NONE', #21114, #21667, #5467, .T. ) ;
#21565=AXIS2_PLACEMENT_3D ( 'NONE', #6877, #14020, #3576 ) ;
#21570=DIRECTION ( 'NONE',  ( 0.000000000000000000, 0.000000000000000000, 1.000000000000000000 ) ) ;
#21571=VECTOR ( 'NONE', #6615, 1000.000000000000000 ) ;
#21572=CARTESIAN_POINT ( 'NONE',  ( 95.25000000000000000, -3568.700000000000273, 2244.547199999999975 ) ) ;
#21576=CARTESIAN_POINT ( 'NONE',  ( 141.7174201517051131, -3577.487138885433524, 2249.884650219001742 ) ) ;
#21578=CIRCLE ( 'NONE', #22675, 2.844800000000091700 ) ;
#21579=CARTESIAN_POINT ( 'NONE',  ( 134.9664275409213587, -3576.291810119500042, 2246.166055327845697 ) ) ;
#21581=ORIENTED_EDGE ( 'NONE', *, *, #1656, .F. ) ;
#21582=ADVANCED_FACE ( 'NONE', ( #17645 ), #6660, .F. ) ;
#21586=ORIENTED_EDGE ( 'NONE', *, *, #9071, .F. ) ;
#21587=DIRECTION ( 'NONE',  ( -0.7249994335945011414, 6.625572310375012166E-14, 0.6887494619146010688 ) ) ;
#21589=VERTEX_POINT ( 'NONE', #10270 ) ;
#21593=DIRECTION ( 'NONE',  ( -1.000000000000000000, 0.000000000000000000, 0.000000000000000000 ) ) ;
#21596=AXIS2_PLACEMENT_3D ( 'NONE', #11867, #15965, #3422 ) ;
#21598=CARTESIAN_POINT ( 'NONE',  ( 9.832632294452492872, -3695.617810904429916, 2254.953892138222272 ) ) ;
#21600=CARTESIAN_POINT ( 'NONE',  ( 18.28253570787369142, -3580.718563225802882, 2245.237727082001129 ) ) ;
#21602=AXIS2_PLACEMENT_3D ( 'NONE', #18535, #832, #19003 ) ;
#21603=EDGE_CURVE ( 'NONE', #13127, #12999, #7336, .T. ) ;
#21604=FACE_OUTER_BOUND ( 'NONE', #7138, .T. ) ;
#21606=TOROIDAL_SURFACE ( 'NONE', #16358, 3.606799999999999784, 0.7620000000000000107 ) ;
#21607=ORIENTED_EDGE ( 'NONE', *, *, #5081, .F. ) ;
#21608=CARTESIAN_POINT ( 'NONE',  ( 138.3834544057343976, -3662.027211347764023, 2249.520849656408245 ) ) ;
#21609=ORIENTED_EDGE ( 'NONE', *, *, #13874, .F. ) ;
#21611=ORIENTED_EDGE ( 'NONE', *, *, #4263, .F. ) ;
#21613=ORIENTED_EDGE ( 'NONE', *, *, #20842, .T. ) ;
#21614=ORIENTED_EDGE ( 'NONE', *, *, #8354, .F. ) ;
#21615=DIRECTION ( 'NONE',  ( 0.000000000000000000, 0.000000000000000000, -1.000000000000000000 ) ) ;
#21622=DIRECTION ( 'NONE',  ( 0.000000000000000000, 0.000000000000000000, 1.000000000000000000 ) ) ;
#21624=DIRECTION ( 'NONE',  ( 0.000000000000000000, 0.000000000000000000, -1.000000000000000000 ) ) ;
#21626=ORIENTED_EDGE ( 'NONE', *, *, #7774, .T. ) ;
#21627=CARTESIAN_POINT ( 'NONE',  ( 131.9075161311309046, -3543.615630485107431, 2260.168083407881113 ) ) ;
#21633=CARTESIAN_POINT ( 'NONE',  ( 151.1299999999999955, -3544.570000000000164, 2240.279999999999745 ) ) ;
#21636=CARTESIAN_POINT ( 'NONE',  ( 142.5447999999989861, -3659.504999999999654, 2272.030000000000200 ) ) ;
#21637=CYLINDRICAL_SURFACE ( 'NONE', #961, 2.844799999999009010 ) ;
#21638=ORIENTED_EDGE ( 'NONE', *, *, #3562, .T. ) ;
#21640=CARTESIAN_POINT ( 'NONE',  ( 35.25520000000000209, -3594.099999999999909, 2259.837999999999738 ) ) ;
#21641=DIRECTION ( 'NONE',  ( -1.000000000000000000, 0.000000000000000000, 0.000000000000000000 ) ) ;
#21642=EDGE_CURVE ( 'NONE', #20964, #6627, #10318, .T. ) ;
#21644=DIRECTION ( 'NONE',  ( 0.000000000000000000, 0.000000000000000000, -1.000000000000000000 ) ) ;
#21645=DIRECTION ( 'NONE',  ( 1.000000000000000000, 0.000000000000000000, 0.000000000000000000 ) ) ;
#21646=CARTESIAN_POINT ( 'NONE',  ( 136.9169929778280164, -3695.514947979135286, 2255.165585416540125 ) ) ;
#21648=CARTESIAN_POINT ( 'NONE',  ( 25.39999999999999858, -3578.860000000000127, 2250.236800000000130 ) ) ;
#21651=CARTESIAN_POINT ( 'NONE',  ( 47.19319999999999737, -3568.700000000000273, 2259.837999999999738 ) ) ;
#21656=DIRECTION ( 'NONE',  ( 0.000000000000000000, 0.000000000000000000, -1.000000000000000000 ) ) ;
#21657=CARTESIAN_POINT ( 'NONE',  ( 92.50679999999999836, -3594.099999999999909, 2239.771999999999935 ) ) ;
#21660=CARTESIAN_POINT ( 'NONE',  ( 132.3005794017000198, -3544.570000000000164, 2260.390449568000349 ) ) ;
#21661=ORIENTED_EDGE ( 'NONE', *, *, #10950, .F. ) ;
#21664=DIRECTION ( 'NONE',  ( 0.000000000000000000, 0.000000000000000000, -1.000000000000000000 ) ) ;
#21665=VERTEX_POINT ( 'NONE', #12729 ) ;
#21667=VERTEX_POINT ( 'NONE', #16470 ) ;
#21668=CARTESIAN_POINT ( 'NONE',  ( 142.3627523022312857, -3695.258941566818521, 2255.466570801501348 ) ) ;
#21671=CARTESIAN_POINT ( 'NONE',  ( 137.8189483952010903, -3581.629460150263640, 2248.048772148962144 ) ) ;
#21672=VERTEX_POINT ( 'NONE', #9336 ) ;
#21674=CARTESIAN_POINT ( 'NONE',  ( 0.000000000000000000, -3544.570000000000164, 2240.279999999999745 ) ) ;
#21676=DIRECTION ( 'NONE',  ( 0.000000000000000000, 0.000000000000000000, -1.000000000000000000 ) ) ;
#21677=CARTESIAN_POINT ( 'NONE',  ( 146.1769999999999925, -3659.504999999999654, 2239.009999999999764 ) ) ;
#21681=CARTESIAN_POINT ( 'NONE',  ( 139.0560147878972828, -3576.723841947683468, 2249.270788651956991 ) ) ;
#21682=ORIENTED_EDGE ( 'NONE', *, *, #9652, .F. ) ;
#21683=CARTESIAN_POINT ( 'NONE',  ( 134.6682978865242148, -3576.785158905799108, 2245.445731933577008 ) ) ;
#21684=AXIS2_PLACEMENT_3D ( 'NONE', #8859, #16003, #12259 ) ;
#21686=VERTEX_POINT ( 'NONE', #3701 ) ;
#21687=DIRECTION ( 'NONE',  ( 0.000000000000000000, 0.000000000000000000, -1.000000000000000000 ) ) ;
#21691=AXIS2_PLACEMENT_3D ( 'NONE', #6142, #18434, #20202 ) ;
#21692=CARTESIAN_POINT ( 'NONE',  ( 111.4552000000009997, -3644.899999999999636, 2259.837999999999738 ) ) ;
#21693=EDGE_CURVE ( 'NONE', #2966, #3298, #8082, .T. ) ;
#21698=CARTESIAN_POINT ( 'NONE',  ( 88.90000000000000568, -3594.099999999999909, 2261.869999999999891 ) ) ;
#21704=AXIS2_PLACEMENT_3D ( 'NONE', #3626, #12541, #17689 ) ;
#21705=CARTESIAN_POINT ( 'NONE',  ( 60.65520000000000067, -3594.099999999999909, 2239.771999999999935 ) ) ;
#21706=CARTESIAN_POINT ( 'NONE',  ( 98.75520000000000209, -3568.700000000000273, 2239.771999999999935 ) ) ;
#21707=ORIENTED_EDGE ( 'NONE', *, *, #3504, .F. ) ;
#21709=DIRECTION ( 'NONE',  ( -1.000000000000000000, 0.000000000000000000, 0.000000000000000000 ) ) ;
#21712=CARTESIAN_POINT ( 'NONE',  ( 137.8779939444977458, -3657.320203822652729, 2246.982792015143787 ) ) ;
#21714=CARTESIAN_POINT ( 'NONE',  ( 137.2246884197096222, -3660.907179621593968, 2250.131455798929437 ) ) ;
#21716=VERTEX_POINT ( 'NONE', #18231 ) ;
#21723=CARTESIAN_POINT ( 'NONE',  ( 15.54479999999932716, -3659.053785370524565, 2256.063560000000962 ) ) ;
#21730=CARTESIAN_POINT ( 'NONE',  ( 7.289238816486445671, -3581.334923857885769, 2245.989158447137015 ) ) ;
#21731=CARTESIAN_POINT ( 'NONE',  ( 53.64479999999999649, -3619.500000000000000, 2261.869999999999891 ) ) ;
#21733=CARTESIAN_POINT ( 'NONE',  ( 88.90000000000000568, -3644.899999999999636, 2261.869999999999891 ) ) ;
#21736=CARTESIAN_POINT ( 'NONE',  ( 35.56000000000000227, -3670.300000000000182, 2247.392000000000280 ) ) ;
#21742=CARTESIAN_POINT ( 'NONE',  ( 129.8447999999989975, -3568.700000000000273, 2259.837999999999738 ) ) ;
#21743=DIRECTION ( 'NONE',  ( 0.000000000000000000, 0.000000000000000000, 1.000000000000000000 ) ) ;
#21745=DIRECTION ( 'NONE',  ( 0.000000000000000000, 0.000000000000000000, -1.000000000000000000 ) ) ;
#21748=CARTESIAN_POINT ( 'NONE',  ( 147.6473055386096007, -3543.381058770634354, 2259.780196767977031 ) ) ;
#21750=CARTESIAN_POINT ( 'NONE',  ( 147.5486189909101995, -3695.492037868064472, 2260.027647172040361 ) ) ;
#21752=EDGE_CURVE ( 'NONE', #15774, #14725, #9924, .T. ) ;
#21755=DIRECTION ( 'NONE',  ( 1.097617497454356000E-13, 0.000000000000000000, 1.000000000000000000 ) ) ;
#21763=FACE_OUTER_BOUND ( 'NONE', #895, .T. ) ;
#21764=CIRCLE ( 'NONE', #9766, 0.7619999999999987894 ) ;
#21766=AXIS2_PLACEMENT_3D ( 'NONE', #1780, #3752, #8924 ) ;
#21767=DIRECTION ( 'NONE',  ( 1.000000000000000000, 0.000000000000000000, 0.000000000000000000 ) ) ;
#21768=DIRECTION ( 'NONE',  ( 0.000000000000000000, -1.000000000000000000, 0.000000000000000000 ) ) ;
#21770=CARTESIAN_POINT ( 'NONE',  ( 76.20000000000000284, -3568.700000000000273, 2239.009999999999764 ) ) ;
#21774=DIRECTION ( 'NONE',  ( 1.000000000000000000, 0.000000000000000000, 0.000000000000000000 ) ) ;
#21775=EDGE_LOOP ( 'NONE', ( #4466, #16827, #12808, #22830, #1527, #7119, #1172, #6779, #14871, #5114, #21586, #640 ) ) ;
#21776=DIRECTION ( 'NONE',  ( 0.000000000000000000, 0.000000000000000000, -1.000000000000000000 ) ) ;
#21778=ORIENTED_EDGE ( 'NONE', *, *, #20465, .F. ) ;
#21779=DIRECTION ( 'NONE',  ( 0.000000000000000000, 0.000000000000000000, -1.000000000000000000 ) ) ;
#21782=EDGE_LOOP ( 'NONE', ( #16325, #19215, #8687, #15985 ) ) ;
#21783=CARTESIAN_POINT ( 'NONE',  ( 142.5673055393761786, -3695.618941230270593, 2254.954196765868346 ) ) ;
#21785=CARTESIAN_POINT ( 'NONE',  ( 137.8884899131788586, -3581.688494919837467, 2247.706546665592668 ) ) ;
#21786=ORIENTED_EDGE ( 'NONE', *, *, #1621, .T. ) ;
#21790=CYLINDRICAL_SURFACE ( 'NONE', #18691, 2.844799999999994444 ) ;
#21792=VECTOR ( 'NONE', #7293, 1000.000000000000000 ) ;
#21793=VECTOR ( 'NONE', #3135, 1000.000000000000000 ) ;
#21797=CARTESIAN_POINT ( 'NONE',  ( 138.1443562676044223, -3577.112753218966191, 2249.637217027982842 ) ) ;
#21798=ORIENTED_EDGE ( 'NONE', *, *, #18857, .T. ) ;
#21799=CARTESIAN_POINT ( 'NONE',  ( 134.0354590894625915, -3578.735571264413466, 2244.549527799902535 ) ) ;
#21801=CARTESIAN_POINT ( 'NONE',  ( 127.0000000000000000, -3578.860000000000127, 2247.392000000000280 ) ) ;
#21805=CIRCLE ( 'NONE', #19936, 2.844799999999009010 ) ;
#21808=DIRECTION ( 'NONE',  ( 0.000000000000000000, -1.000000000000000000, 0.000000000000000000 ) ) ;
#21810=ORIENTED_EDGE ( 'NONE', *, *, #21820, .F. ) ;
#21815=CARTESIAN_POINT ( 'NONE',  ( 141.5113688234855545, -3581.688645776049725, 2247.086479173670796 ) ) ;
#21816=EDGE_LOOP ( 'NONE', ( #19715, #12605, #11724, #10250 ) ) ;
#21820=EDGE_CURVE ( 'NONE', #10484, #3518, #18563, .T. ) ;
#21822=DIRECTION ( 'NONE',  ( 0.000000000000000000, 0.000000000000000000, -1.000000000000000000 ) ) ;
#21823=ORIENTED_EDGE ( 'NONE', *, *, #10437, .T. ) ;
#21824=CARTESIAN_POINT ( 'NONE',  ( 1.270000000000000018, -3694.430000000000291, 2240.279999999999745 ) ) ;
#21829=EDGE_LOOP ( 'NONE', ( #16367, #10528, #22488, #2004 ) ) ;
#21830=ORIENTED_EDGE ( 'NONE', *, *, #1697, .F. ) ;
#21831=VECTOR ( 'NONE', #9313, 1000.000000000000000 ) ;
#21832=CARTESIAN_POINT ( 'NONE',  ( 138.8454383216908070, -3662.218504070199288, 2249.334367105925594 ) ) ;
#21835=ORIENTED_EDGE ( 'NONE', *, *, #10438, .T. ) ;
#21837=ORIENTED_EDGE ( 'NONE', *, *, #11102, .T. ) ;
#21838=DIRECTION ( 'NONE',  ( 0.000000000000000000, -1.000000000000000000, 0.000000000000000000 ) ) ;
#21839=EDGE_CURVE ( 'NONE', #14116, #13045, #14468, .T. ) ;
#21840=CARTESIAN_POINT ( 'NONE',  ( 110.6932000000009992, -3644.899999999999636, 2260.600000000000364 ) ) ;
#21841=CIRCLE ( 'NONE', #7258, 1.269999999999882334 ) ;
#21842=ORIENTED_EDGE ( 'NONE', *, *, #15826, .F. ) ;
#21845=CARTESIAN_POINT ( 'NONE',  ( 7.197112922637037613, -3581.033299165524113, 2245.555178679493110 ) ) ;
#21848=VECTOR ( 'NONE', #16066, 1000.000000000000000 ) ;
#21852=CARTESIAN_POINT ( 'NONE',  ( 63.50000000000000000, -3644.899999999999636, 2259.837999999999738 ) ) ;
#21857=CARTESIAN_POINT ( 'NONE',  ( 35.56000000000000227, -3695.699999999999818, 2243.277199999999993 ) ) ;
#21860=CARTESIAN_POINT ( 'NONE',  ( 25.39999999999999858, -3670.300000000000182, 2239.009999999999764 ) ) ;
#21861=DIRECTION ( 'NONE',  ( -1.000000000000000000, 0.000000000000000000, 0.000000000000000000 ) ) ;
#21862=ORIENTED_EDGE ( 'NONE', *, *, #5288, .T. ) ;
#21863=CARTESIAN_POINT ( 'NONE',  ( 147.6177471794484859, -3695.586719555673881, 2259.854339697793421 ) ) ;
#21865=CARTESIAN_POINT ( 'NONE',  ( 38.10000000000000142, -3644.899999999999636, 2239.009999999999764 ) ) ;
#21867=CARTESIAN_POINT ( 'NONE',  ( 25.39999999999999858, -3568.700000000000273, 2239.771999999999935 ) ) ;
#21868=CARTESIAN_POINT ( 'NONE',  ( 142.5673427038165642, -3543.381058771931293, 2254.954211610746825 ) ) ;
#21873=VECTOR ( 'NONE', #14378, 1000.000000000000000 ) ;
#21874=CARTESIAN_POINT ( 'NONE',  ( 145.3974439044723113, -3659.043045737660577, 2244.764295548285190 ) ) ;
#21875=DIRECTION ( 'NONE',  ( 0.000000000000000000, -1.000000000000000000, 0.000000000000000000 ) ) ;
#21876=CARTESIAN_POINT ( 'NONE',  ( 117.1447999999989946, -3594.099999999999909, 2259.837999999999738 ) ) ;
#21877=CARTESIAN_POINT ( 'NONE',  ( 34.49320000000000164, -3594.099999999999909, 2260.600000000000364 ) ) ;
#21880=ADVANCED_FACE ( 'NONE', ( #4502 ), #15179, .T. ) ;
#21882=ORIENTED_EDGE ( 'NONE', *, *, #22247, .T. ) ;
#21884=CARTESIAN_POINT ( 'NONE',  ( 151.4000000000000057, -3544.570000000000164, 2260.570967364599255 ) ) ;
#21887=AXIS2_PLACEMENT_3D ( 'NONE', #6023, #14925, #9747 ) ;
#21888=ORIENTED_EDGE ( 'NONE', *, *, #17116, .T. ) ;
#21889=EDGE_CURVE ( 'NONE', #11527, #8900, #19037, .T. ) ;
#21892=ORIENTED_EDGE ( 'NONE', *, *, #10960, .T. ) ;
#21895=EDGE_CURVE ( 'NONE', #279, #5355, #18916, .T. ) ;
#21898=CARTESIAN_POINT ( 'NONE',  ( 57.14999999999999858, -3694.430000000000291, 2247.392000000000280 ) ) ;
#21899=CIRCLE ( 'NONE', #12550, 3.606799999999993567 ) ;
#21900=ORIENTED_EDGE ( 'NONE', *, *, #12865, .T. ) ;
#21901=CARTESIAN_POINT ( 'NONE',  ( 145.1247579277662112, -3581.293143190419869, 2245.917988638741008 ) ) ;
#21907=CARTESIAN_POINT ( 'NONE',  ( 17.58063922156827630, -3662.478349466719010, 2245.771667880976565 ) ) ;
#21911=CARTESIAN_POINT ( 'NONE',  ( 139.5668999253178697, -3576.650121873226453, 2249.183459103710447 ) ) ;
#21913=DIRECTION ( 'NONE',  ( 0.000000000000000000, 0.000000000000000000, 1.000000000000000000 ) ) ;
#21915=AXIS2_PLACEMENT_3D ( 'NONE', #9221, #4053, #21975 ) ;
#21917=CARTESIAN_POINT ( 'NONE',  ( 15.24000000000000021, -3544.570000000000164, 2255.774000000000342 ) ) ;
#21919=CIRCLE ( 'NONE', #21180, 1.269999999999882334 ) ;
#21920=ORIENTED_EDGE ( 'NONE', *, *, #21839, .F. ) ;
#21922=DIRECTION ( 'NONE',  ( 0.000000000000000000, 0.000000000000000000, -1.000000000000000000 ) ) ;
#21923=ORIENTED_EDGE ( 'NONE', *, *, #17606, .F. ) ;
#21925=CARTESIAN_POINT ( 'NONE',  ( 14.13894186833527655, -3577.040487938397291, 2249.579033631703169 ) ) ;
#21927=EDGE_LOOP ( 'NONE', ( #6597, #15836, #13254, #21373 ) ) ;
#21933=AXIS2_PLACEMENT_3D ( 'NONE', #10475, #12242, #22771 ) ;
#21934=TOROIDAL_SURFACE ( 'NONE', #8826, 6.477000000001000402, 0.7620000000000000107 ) ;
#21936=TOROIDAL_SURFACE ( 'NONE', #238, 3.606799999999999784, 0.7620000000000000107 ) ;
#21938=CARTESIAN_POINT ( 'NONE',  ( 137.9195094541193214, -3661.723873492530402, 2249.755159743324384 ) ) ;
#21940=ORIENTED_EDGE ( 'NONE', *, *, #3127, .T. ) ;
#21946=CARTESIAN_POINT ( 'NONE',  ( 35.56000000000000227, -3544.570000000000164, 2250.236800000000130 ) ) ;
#21947=EDGE_CURVE ( 'NONE', #9977, #16048, #10337, .T. ) ;
#21948=VERTEX_POINT ( 'NONE', #19153 ) ;
#21949=AXIS2_PLACEMENT_3D ( 'NONE', #8311, #16857, #6212 ) ;
#21950=CARTESIAN_POINT ( 'NONE',  ( 6.999092514601316317, -3659.102275462906164, 2244.742506506137033 ) ) ;
#21952=AXIS2_PLACEMENT_3D ( 'NONE', #7735, #11241, #7608 ) ;
#21953=CARTESIAN_POINT ( 'NONE',  ( 116.8400000000000034, -3544.570000000000164, 2247.392000000000280 ) ) ;
#21956=DIRECTION ( 'NONE',  ( 0.000000000000000000, 0.000000000000000000, 1.000000000000000000 ) ) ;
#21957=ORIENTED_EDGE ( 'NONE', *, *, #4147, .F. ) ;
#21960=EDGE_LOOP ( 'NONE', ( #4621, #23133, #488, #4672, #4086, #12297, #5626, #2514 ) ) ;
#21961=AXIS2_PLACEMENT_3D ( 'NONE', #7, #1873, #5398 ) ;
#21962=FACE_OUTER_BOUND ( 'NONE', #9883, .T. ) ;
#21965=DIRECTION ( 'NONE',  ( 1.000000000000000000, 0.000000000000000000, 0.000000000000000000 ) ) ;
#21969=CARTESIAN_POINT ( 'NONE',  ( 7.020348529275000082, -3578.860230781999689, 2244.548186305999934 ) ) ;
#21973=DIRECTION ( 'NONE',  ( 0.000000000000000000, 0.000000000000000000, -1.000000000000000000 ) ) ;
#21975=DIRECTION ( 'NONE',  ( 1.000000000000000000, 0.000000000000000000, 0.000000000000000000 ) ) ;
#21978=CARTESIAN_POINT ( 'NONE',  ( 142.3712129903081518, -3543.717426572816294, 2255.445345401364193 ) ) ;
#21980=CARTESIAN_POINT ( 'NONE',  ( 7.057989306600019219, -3578.573285425562972, 2244.557874998726220 ) ) ;
#21984=CARTESIAN_POINT ( 'NONE',  ( 145.4149999979000256, -3659.390788570165569, 2244.645112239727041 ) ) ;
#21987=CARTESIAN_POINT ( 'NONE',  ( 9.887444566626168552, -3579.928195997985313, 2250.029480932760180 ) ) ;
#21988=VECTOR ( 'NONE', #17220, 1000.000000000000000 ) ;
#21990=EDGE_CURVE ( 'NONE', #21351, #2568, #6610, .T. ) ;
#21992=DIRECTION ( 'NONE',  ( -1.000000000000000000, 0.000000000000000000, 0.000000000000000000 ) ) ;
#21994=EDGE_LOOP ( 'NONE', ( #1879, #5178 ) ) ;
#21996=VECTOR ( 'NONE', #21191, 1000.000000000000000 ) ;
#21997=DIRECTION ( 'NONE',  ( -1.000000000000000000, 0.000000000000000000, 0.000000000000000000 ) ) ;
#21998=VERTEX_POINT ( 'NONE', #12118 ) ;
#21999=CARTESIAN_POINT ( 'NONE',  ( 10.78733304872000076, -3657.399152860999493, 2246.630000000000109 ) ) ;
#22000=DIRECTION ( 'NONE',  ( -1.000000000000000000, 0.000000000000000000, 0.000000000000000000 ) ) ;
#22001=AXIS2_PLACEMENT_3D ( 'NONE', #7789, #9090, #7333 ) ;
#22002=EDGE_CURVE ( 'NONE', #5746, #11629, #12216, .T. ) ;
#22004=DIRECTION ( 'NONE',  ( 0.000000000000000000, 0.000000000000000000, -1.000000000000000000 ) ) ;
#22006=VERTEX_POINT ( 'NONE', #12355 ) ;
#22007=ADVANCED_FACE ( 'NONE', ( #17737 ), #19501, .F. ) ;
#22009=DIRECTION ( 'NONE',  ( 0.000000000000000000, 0.000000000000000000, -1.000000000000000000 ) ) ;
#22011=CARTESIAN_POINT ( 'NONE',  ( 145.3179258180492752, -3580.544012085779286, 2245.098288301110188 ) ) ;
#22014=CARTESIAN_POINT ( 'NONE',  ( 17.87993129502918777, -3661.919911407861491, 2245.171352655763712 ) ) ;
#22015=EDGE_CURVE ( 'NONE', #4703, #15062, #1733, .T. ) ;
#22018=CARTESIAN_POINT ( 'NONE',  ( 141.5164385476758753, -3577.305427569615858, 2249.774537136630897 ) ) ;
#22022=DIRECTION ( 'NONE',  ( 0.000000000000000000, 1.000000000000000000, 0.000000000000000000 ) ) ;
#22025=DIRECTION ( 'NONE',  ( 0.000000000000000000, 0.000000000000000000, -1.000000000000000000 ) ) ;
#22026=ORIENTED_EDGE ( 'NONE', *, *, #4987, .T. ) ;
#22027=DIRECTION ( 'NONE',  ( -1.000000000000000000, 0.000000000000000000, 0.000000000000000000 ) ) ;
#22032=EDGE_CURVE ( 'NONE', #9684, #17959, #17814, .T. ) ;
#22033=CARTESIAN_POINT ( 'NONE',  ( 14.37057332318734382, -3577.190483362103805, 2249.696470782429969 ) ) ;
#22035=CARTESIAN_POINT ( 'NONE',  ( 142.0869831723413199, -3581.042548131108560, 2249.216657478487832 ) ) ;
#22036=VERTEX_POINT ( 'NONE', #6742 ) ;
#22037=DIRECTION ( 'NONE',  ( -1.000000000000000000, 0.000000000000000000, 0.000000000000000000 ) ) ;
#22039=DIRECTION ( 'NONE',  ( 1.000000000000000000, 0.000000000000000000, 0.000000000000000000 ) ) ;
#22040=CARTESIAN_POINT ( 'NONE',  ( 25.39999999999999858, -3660.140000000000327, 2247.392000000000280 ) ) ;
#22044=ORIENTED_EDGE ( 'NONE', *, *, #19094, .F. ) ;
#22046=CARTESIAN_POINT ( 'NONE',  ( 140.2432324407819237, -3662.298289484956513, 2249.245429607616643 ) ) ;
#22048=ORIENTED_EDGE ( 'NONE', *, *, #18850, .T. ) ;
#22049=VERTEX_POINT ( 'NONE', #8610 ) ;
#22054=AXIS2_PLACEMENT_3D ( 'NONE', #22705, #13694, #1257 ) ;
#22055=ORIENTED_EDGE ( 'NONE', *, *, #837, .T. ) ;
#22058=DIRECTION ( 'NONE',  ( -4.702395060216999850E-14, -1.000000000000000000, 1.319970543219000025E-14 ) ) ;
#22065=DIRECTION ( 'NONE',  ( 0.000000000000000000, 0.000000000000000000, 1.000000000000000000 ) ) ;
#22066=CARTESIAN_POINT ( 'NONE',  ( 144.3113860274000047, -3662.880847139000252, 2246.630000000000109 ) ) ;
#22067=LINE ( 'NONE', #12608, #13765 ) ;
#22069=B_SPLINE_CURVE_WITH_KNOTS ( 'NONE', 3,
 ( #3963, #10997, #7712, #21999 ),
 .UNSPECIFIED., .F., .F.,
 ( 4, 4 ),
 ( 0.000000000000000000, 1.000000000000000000 ),
 .UNSPECIFIED. ) ;
#22070=FACE_OUTER_BOUND ( 'NONE', #6257, .T. ) ;
#22074=ORIENTED_EDGE ( 'NONE', *, *, #15512, .F. ) ;
#22077=VERTEX_POINT ( 'NONE', #19620 ) ;
#22084=CARTESIAN_POINT ( 'NONE',  ( 116.8400000000000034, -3694.430000000000291, 2247.392000000000280 ) ) ;
#22089=AXIS2_PLACEMENT_3D ( 'NONE', #6322, #13455, #2784 ) ;
#22094=CARTESIAN_POINT ( 'NONE',  ( 9.915707903441028037, -3580.080243487859207, 2249.961828650349162 ) ) ;
#22096=EDGE_CURVE ( 'NONE', #22077, #8967, #20810, .T. ) ;
#22097=FACE_OUTER_BOUND ( 'NONE', #19397, .T. ) ;
#22098=EDGE_CURVE ( 'NONE', #18111, #2160, #20914, .T. ) ;
#22100=LINE ( 'NONE', #2205, #2902 ) ;
#22101=ADVANCED_FACE ( 'NONE', ( #12592 ), #54, .F. ) ;
#22103=CARTESIAN_POINT ( 'NONE',  ( 9.855190710340998805, -3579.495000415000050, 2250.165025612000136 ) ) ;
#22104=CARTESIAN_POINT ( 'NONE',  ( 13.37322708549078065, -3662.269940902608596, 2249.277995755860502 ) ) ;
#22112=ORIENTED_EDGE ( 'NONE', *, *, #22969, .F. ) ;
#22114=DIRECTION ( 'NONE',  ( 0.000000000000000000, 0.000000000000000000, -1.000000000000000000 ) ) ;
#22115=ADVANCED_FACE ( 'NONE', ( #5447 ), #15298, .T. ) ;
#22116=ORIENTED_EDGE ( 'NONE', *, *, #620, .T. ) ;
#22117=AXIS2_PLACEMENT_3D ( 'NONE', #20925, #19401, #13895 ) ;
#22118=EDGE_LOOP ( 'NONE', ( #13040, #9111, #5769, #15589 ) ) ;
#22121=ORIENTED_EDGE ( 'NONE', *, *, #12670, .T. ) ;
#22122=CARTESIAN_POINT ( 'NONE',  ( 145.0727138887509398, -3581.449656632165443, 2246.178647461291348 ) ) ;
#22124=CARTESIAN_POINT ( 'NONE',  ( 145.3795747169000094, -3578.859731361000286, 2244.547525601999951 ) ) ;
#22125=CARTESIAN_POINT ( 'NONE',  ( 18.21227314848903944, -3661.013619535250200, 2244.684649758042724 ) ) ;
#22126=EDGE_CURVE ( 'NONE', #11962, #7810, #4361, .T. ) ;
#22127=CARTESIAN_POINT ( 'NONE',  ( 79.80679999999999552, -3568.700000000000273, 2259.837999999999738 ) ) ;
#22128=ADVANCED_FACE ( 'NONE', ( #1922 ), #2946, .T. ) ;
#22129=CARTESIAN_POINT ( 'NONE',  ( 137.7151180025381336, -3577.456461149886763, 2249.866723821840424 ) ) ;
#22133=CIRCLE ( 'NONE', #19897, 2.844799999998931295 ) ;
#22134=DIRECTION ( 'NONE',  ( 1.000000000000000000, 0.000000000000000000, 0.000000000000000000 ) ) ;
#22136=CARTESIAN_POINT ( 'NONE',  ( 18.37893127878000143, -3660.140301727999940, 2244.547200027999679 ) ) ;
#22139=ORIENTED_EDGE ( 'NONE', *, *, #10361, .F. ) ;
#22141=CARTESIAN_POINT ( 'NONE',  ( 101.5999999999999943, -3619.500000000000000, 2260.600000000000364 ) ) ;
#22144=CARTESIAN_POINT ( 'NONE',  ( 14.17803026764341467, -3577.063814636674124, 2249.598259528346262 ) ) ;
#22145=CARTESIAN_POINT ( 'NONE',  ( 142.4822567032824452, -3580.090015056482571, 2249.957167306039082 ) ) ;
#22146=ORIENTED_EDGE ( 'NONE', *, *, #4364, .T. ) ;
#22150=CIRCLE ( 'NONE', #1961, 2.844800000000091700 ) ;
#22151=CARTESIAN_POINT ( 'NONE',  ( 12.69999999999999929, -3579.494999999999891, 2239.771999999999935 ) ) ;
#22152=DIRECTION ( 'NONE',  ( -1.224646799147353207E-16, 1.000000000000000000, 0.000000000000000000 ) ) ;
#22153=CARTESIAN_POINT ( 'NONE',  ( 139.6999999999999886, -3659.504999999999654, 2246.630000000000109 ) ) ;
#22155=CIRCLE ( 'NONE', #4205, 3.606799999999993567 ) ;
#22157=EDGE_CURVE ( 'NONE', #14295, #7706, #7201, .T. ) ;
#22159=EDGE_LOOP ( 'NONE', ( #4222, #11473, #2332, #21441, #23014 ) ) ;
#22160=EDGE_CURVE ( 'NONE', #12867, #11171, #2105, .T. ) ;
#22163=AXIS2_PLACEMENT_3D ( 'NONE', #16953, #783, #11454 ) ;
#22164=DIRECTION ( 'NONE',  ( -1.000000000000000000, 0.000000000000000000, 0.000000000000000000 ) ) ;
#22167=DIRECTION ( 'NONE',  ( 1.000000000000000000, 0.000000000000000000, 0.000000000000000000 ) ) ;
#22168=EDGE_CURVE ( 'NONE', #21153, #13850, #7728, .T. ) ;
#22171=CYLINDRICAL_SURFACE ( 'NONE', #4721, 1.269999999999882334 ) ;
#22172=DIRECTION ( 'NONE',  ( 0.000000000000000000, 0.000000000000000000, 1.000000000000000000 ) ) ;
#22173=CYLINDRICAL_SURFACE ( 'NONE', #2378, 1.269999999999993356 ) ;
#22178=ADVANCED_FACE ( 'NONE', ( #2217 ), #23143, .T. ) ;
#22182=ORIENTED_EDGE ( 'NONE', *, *, #22517, .T. ) ;
#22183=CARTESIAN_POINT ( 'NONE',  ( 9.926985991717000246, -3578.860012824000023, 2250.236835079999764 ) ) ;
#22184=CARTESIAN_POINT ( 'NONE',  ( 0.000000000000000000, -3544.570000000000164, 2259.329999999999927 ) ) ;
#22189=DIRECTION ( 'NONE',  ( 0.000000000000000000, 0.000000000000000000, -1.000000000000000000 ) ) ;
#22192=CARTESIAN_POINT ( 'NONE',  ( 25.39999999999999858, -3660.140000000000327, 2250.236800000000130 ) ) ;
#22196=VECTOR ( 'NONE', #8342, 1000.000000000000000 ) ;
#22200=LINE ( 'NONE', #18802, #8336 ) ;
#22201=VERTEX_POINT ( 'NONE', #5266 ) ;
#22206=CARTESIAN_POINT ( 'NONE',  ( 91.74479999999999791, -3594.099999999999909, 2239.771999999999935 ) ) ;
#22212=CARTESIAN_POINT ( 'NONE',  ( 15.47299515201000020, -3578.859991782000179, 2250.236800948000109 ) ) ;
#22213=DIRECTION ( 'NONE',  ( 0.000000000000000000, 0.000000000000000000, -1.000000000000000000 ) ) ;
#22218=PLANE ( 'NONE',  #11435 ) ;
#22219=ADVANCED_FACE ( 'NONE', ( #11001 ), #2563, .T. ) ;
#22225=ADVANCED_FACE ( 'NONE', ( #17797 ), #10770, .F. ) ;
#22228=CARTESIAN_POINT ( 'NONE',  ( 145.2068972130955160, -3581.023318633427607, 2245.544194199756021 ) ) ;
#22231=CARTESIAN_POINT ( 'NONE',  ( 17.31138602737999932, -3662.880847139000252, 2246.630000000000109 ) ) ;
#22233=PLANE ( 'NONE',  #14859 ) ;
#22237=DIRECTION ( 'NONE',  ( -1.000000000000000000, 0.000000000000000000, 0.000000000000000000 ) ) ;
#22240=CARTESIAN_POINT ( 'NONE',  ( 57.15000000000030411, -3568.700000000000273, 2250.236800000000130 ) ) ;
#22243=VERTEX_POINT ( 'NONE', #10491 ) ;
#22247=EDGE_CURVE ( 'NONE', #14198, #5555, #8188, .T. ) ;
#22249=VECTOR ( 'NONE', #2402, 1000.000000000000000 ) ;
#22251=ORIENTED_EDGE ( 'NONE', *, *, #17519, .F. ) ;
#22252=AXIS2_PLACEMENT_3D ( 'NONE', #8434, #6687, #13825 ) ;
#22255=CARTESIAN_POINT ( 'NONE',  ( 11.46140658660981693, -3576.933588766896719, 2249.485458673201265 ) ) ;
#22257=CARTESIAN_POINT ( 'NONE',  ( 142.0110375026553129, -3581.154241066639315, 2249.074962378318560 ) ) ;
#22262=CARTESIAN_POINT ( 'NONE',  ( 20.60974739964567348, -3543.420597440594065, 2259.874498643110655 ) ) ;
#22264=CIRCLE ( 'NONE', #14432, 0.7619999999999987894 ) ;
#22270=ORIENTED_EDGE ( 'NONE', *, *, #8662, .F. ) ;
#22274=DIRECTION ( 'NONE',  ( -1.000000000000000000, 0.000000000000000000, 0.000000000000000000 ) ) ;
#22275=DIRECTION ( 'NONE',  ( 0.000000000000000000, 0.000000000000000000, 1.000000000000000000 ) ) ;
#22276=ORIENTED_EDGE ( 'NONE', *, *, #21947, .F. ) ;
#22277=ADVANCED_FACE ( 'NONE', ( #9472 ), #11185, .T. ) ;
#22280=CIRCLE ( 'NONE', #11803, 2.844800000000001550 ) ;
#22282=DIRECTION ( 'NONE',  ( 0.000000000000000000, -1.000000000000000000, 0.000000000000000000 ) ) ;
#22284=EDGE_CURVE ( 'NONE', #15874, #21686, #7443, .T. ) ;
#22286=ADVANCED_FACE ( 'NONE', ( #22338 ), #4313, .F. ) ;
#22287=DIRECTION ( 'NONE',  ( 0.000000000000000000, 0.000000000000000000, -1.000000000000000000 ) ) ;
#22291=DIRECTION ( 'NONE',  ( -0.000000000000000000, -1.000000000000000000, -0.000000000000000000 ) ) ;
#22296=DIRECTION ( 'NONE',  ( -1.000000000000000000, 0.000000000000000000, 0.000000000000000000 ) ) ;
#22303=EDGE_CURVE ( 'NONE', #6778, #10158, #9688, .T. ) ;
#22304=CARTESIAN_POINT ( 'NONE',  ( 101.5999999999999943, -3670.300000000000182, 2260.600000000000364 ) ) ;
#22305=ORIENTED_EDGE ( 'NONE', *, *, #63, .T. ) ;
#22306=VERTEX_POINT ( 'NONE', #14979 ) ;
#22309=AXIS2_PLACEMENT_3D ( 'NONE', #2059, #20213, #14489 ) ;
#22312=CARTESIAN_POINT ( 'NONE',  ( 142.4730239663999782, -3578.859999866000180, 2250.236800057000437 ) ) ;
#22319=VECTOR ( 'NONE', #13482, 1000.000000000000000 ) ;
#22321=AXIS2_PLACEMENT_3D ( 'NONE', #20644, #11292, #632 ) ;
#22323=AXIS2_PLACEMENT_3D ( 'NONE', #2564, #9710, #20490 ) ;
#22324=EDGE_LOOP ( 'NONE', ( #22910, #13932 ) ) ;
#22326=CIRCLE ( 'NONE', #5142, 1.269999999999882334 ) ;
#22327=DIRECTION ( 'NONE',  ( 0.000000000000000000, 0.000000000000000000, 1.000000000000000000 ) ) ;
#22328=CARTESIAN_POINT ( 'NONE',  ( 145.3724401638749839, -3660.201886162340543, 2244.547775376675872 ) ) ;
#22329=ORIENTED_EDGE ( 'NONE', *, *, #468, .T. ) ;
#22330=DIRECTION ( 'NONE',  ( 0.000000000000000000, -1.000000000000000000, 0.000000000000000000 ) ) ;
#22331=EDGE_CURVE ( 'NONE', #4775, #10874, #13060, .T. ) ;
#22337=CIRCLE ( 'NONE', #5908, 2.844800000000091700 ) ;
#22338=FACE_OUTER_BOUND ( 'NONE', #13293, .T. ) ;
#22339=CARTESIAN_POINT ( 'NONE',  ( 136.6540434515666504, -3581.600851036878794, 2246.630014020016006 ) ) ;
#22341=VERTEX_POINT ( 'NONE', #18373 ) ;
#22342=CIRCLE ( 'NONE', #15626, 1.240967364599221412 ) ;
#22343=VECTOR ( 'NONE', #19953, 1000.000000000000000 ) ;
#22344=LINE ( 'NONE', #18713, #21044 ) ;
#22346=B_SPLINE_CURVE_WITH_KNOTS ( 'NONE', 3,
 ( #16627, #5875, #4098, #18274, #11015, #584, #5981, #16177, #14424, #5530, #9268, #7738, #128, #13013, #12772, #7273, #12659, #18159, #21576, #469, #14890, #22018, #11244, #20049, #13119, #5639, #1999, #7610, #9379, #14545, #20272, #4214, #17924, #1878, #3985, #16404, #3743, #11136, #18390, #21911, #9030, #10900, #9488, #21681, #7392, #16513, #19812, #20160, #2344, #356, #14771, #14656, #7497, #18049, #19928, #9149, #21797, #16290, #251, #5758, #12892, #6100, #20719, #22129, #2461, #6561, #15110, #14996, #13699, #2914, #20601, #795, #17199, #11352, #1145, #2567, #16970, #10054 ),
 .UNSPECIFIED., .F., .F.,
 ( 4, 2, 2, 1, 2, 2, 2, 1, 2, 2, 2, 1, 2, 2, 2, 2, 2, 2, 1, 2, 2, 2, 2, 2, 1, 2, 2, 2, 2, 2, 2, 1, 2, 2, 2, 1, 2, 2, 2, 1, 2, 2, 4 ),
 ( 0.000000000000000000, 0.06249999999892112690, 0.09374999999839656040, 0.1093749999981342841, 0.1171874999980031529, 0.1249999999978720078, 0.1562499999974240328, 0.1718749999971419806, 0.1796874999969980680, 0.1874999999968541553, 0.2187499999964742092, 0.2343749999963266051, 0.2421874999962923825, 0.2499999999962581598, 0.2812499999963358199, 0.2968749999963781194, 0.3124999999964203634, 0.3437499999965609732, 0.3593749999966041053, 0.3671874999966006636, 0.3749999999965971664, 0.4999999999971623810, 0.5624999999974512610, 0.5937499999976098009, 0.6093749999976889598, 0.6171874999977259302, 0.6249999999977630116, 0.6562499999977361442, 0.6718749999976957321, 0.6874999999976552090, 0.7187499999976278975, 0.7343749999976073584, 0.7421874999976002529, 0.7499999999975931475, 0.7812499999979156673, 0.7968749999980019316, 0.8046874999980959675, 0.8124999999981898924, 0.8437499999986749488, 0.8593749999989175326, 0.8671874999990610844, 0.8749999999992046362, 1.000000000000000000 ),
 .UNSPECIFIED. ) ;
#22347=CARTESIAN_POINT ( 'NONE',  ( 145.1333241165027630, -3581.267160291652999, 2245.875868943096521 ) ) ;
#22353=CARTESIAN_POINT ( 'NONE',  ( 40.94480000000000075, -3594.099999999999909, 2259.837999999999738 ) ) ;
#22354=AXIS2_PLACEMENT_3D ( 'NONE', #14510, #5250, #16142 ) ;
#22357=B_SPLINE_CURVE_WITH_KNOTS ( 'NONE', 3,
 ( #9913, #20579, #17062, #11795 ),
 .UNSPECIFIED., .F., .F.,
 ( 4, 4 ),
 ( 0.000000000000000000, 1.000000000000000000 ),
 .UNSPECIFIED. ) ;
#22358=DIRECTION ( 'NONE',  ( 0.000000000000000000, 1.000000000000000000, -1.224646799147353207E-16 ) ) ;
#22362=DIRECTION ( 'NONE',  ( 0.000000000000000000, 0.000000000000000000, -1.000000000000000000 ) ) ;
#22363=CARTESIAN_POINT ( 'NONE',  ( 15.42885205981449737, -3543.580319130768657, 2255.300839617613747 ) ) ;
#22364=VERTEX_POINT ( 'NONE', #14872 ) ;
#22366=ORIENTED_EDGE ( 'NONE', *, *, #11567, .F. ) ;
#22370=DIRECTION ( 'NONE',  ( 1.224646799147353207E-16, 1.000000000000000000, -0.000000000000000000 ) ) ;
#22371=CARTESIAN_POINT ( 'NONE',  ( 10.81400611534258083, -3577.363169334261784, 2249.812237833679774 ) ) ;
#22373=CARTESIAN_POINT ( 'NONE',  ( 141.5988453809077896, -3581.613352772223152, 2248.107586786265529 ) ) ;
#22374=ORIENTED_EDGE ( 'NONE', *, *, #3256, .F. ) ;
#22375=DIRECTION ( 'NONE',  ( 1.000000000000000000, 0.000000000000000000, 0.000000000000000000 ) ) ;
#22379=CARTESIAN_POINT ( 'NONE',  ( 29.00679999999900005, -3568.700000000000273, 2239.009999999999764 ) ) ;
#22380=CARTESIAN_POINT ( 'NONE',  ( 134.3871257472000025, -3657.399152860999493, 2246.630000000000109 ) ) ;
#22382=ADVANCED_FACE ( 'NONE', ( #20254 ), #9916, .F. ) ;
#22384=CYLINDRICAL_SURFACE ( 'NONE', #2458, 1.269999999999882334 ) ;
#22385=EDGE_CURVE ( 'NONE', #12207, #20359, #11537, .T. ) ;
#22388=ORIENTED_EDGE ( 'NONE', *, *, #11023, .T. ) ;
#22390=ORIENTED_EDGE ( 'NONE', *, *, #22331, .F. ) ;
#22395=CARTESIAN_POINT ( 'NONE',  ( 6.988638255462328530, -3659.275913659694197, 2244.678801586293503 ) ) ;
#22396=DIRECTION ( 'NONE',  ( -1.224646799147353207E-16, 1.000000000000000000, 0.000000000000000000 ) ) ;
#22397=EDGE_CURVE ( 'NONE', #20612, #5300, #1835, .T. ) ;
#22399=B_SPLINE_CURVE_WITH_KNOTS ( 'NONE', 3,
 ( #13751, #1546, #10219, #15849, #17711, #21247 ),
 .UNSPECIFIED., .F., .F.,
 ( 4, 1, 1, 4 ),
 ( 0.000000000000000000, 0.3333333333333000081, 0.6666666666667000474, 1.000000000000000000 ),
 .UNSPECIFIED. ) ;
#22404=CARTESIAN_POINT ( 'NONE',  ( 142.5447969220999767, -3659.505006299999877, 2250.165025787000104 ) ) ;
#22405=LINE ( 'NONE', #15051, #16754 ) ;
#22406=ORIENTED_EDGE ( 'NONE', *, *, #3964, .F. ) ;
#22413=ADVANCED_FACE ( 'NONE', ( #15673 ), #5130, .F. ) ;
#22415=CARTESIAN_POINT ( 'NONE',  ( 151.1299999999999955, -3578.860000000000127, 2247.392000000000280 ) ) ;
#22417=ORIENTED_EDGE ( 'NONE', *, *, #5225, .F. ) ;
#22422=CARTESIAN_POINT ( 'NONE',  ( 25.39999999999999858, -3568.700000000000273, 2260.600000000000364 ) ) ;
#22425=ORIENTED_EDGE ( 'NONE', *, *, #20548, .F. ) ;
#22427=ORIENTED_EDGE ( 'NONE', *, *, #9513, .T. ) ;
#22429=EDGE_CURVE ( 'NONE', #12173, #2094, #7146, .T. ) ;
#22430=AXIS2_PLACEMENT_3D ( 'NONE', #16170, #18042, #21676 ) ;
#22431=CARTESIAN_POINT ( 'NONE',  ( 57.14999999999999858, -3695.699999999999818, 2243.277199999999993 ) ) ;
#22432=DIRECTION ( 'NONE',  ( 0.000000000000000000, 0.000000000000000000, -1.000000000000000000 ) ) ;
#22434=ORIENTED_EDGE ( 'NONE', *, *, #10154, .F. ) ;
#22435=DIRECTION ( 'NONE',  ( 1.000000000000000000, 0.000000000000000000, 0.000000000000000000 ) ) ;
#22437=CARTESIAN_POINT ( 'NONE',  ( 144.5596709333768786, -3662.512440222478745, 2245.822145638152051 ) ) ;
#22438=ORIENTED_EDGE ( 'NONE', *, *, #3375, .T. ) ;
#22439=CARTESIAN_POINT ( 'NONE',  ( 15.54479999999999862, -3579.494999999999891, 2256.063560000000052 ) ) ;
#22440=CARTESIAN_POINT ( 'NONE',  ( 14.00164913856103155, -3662.034655424634366, 2249.514152627225485 ) ) ;
#22442=EDGE_CURVE ( 'NONE', #19682, #21716, #1367, .T. ) ;
#22446=DIRECTION ( 'NONE',  ( 0.000000000000000000, 0.000000000000000000, -1.000000000000000000 ) ) ;
#22447=CARTESIAN_POINT ( 'NONE',  ( 151.4000000000000057, 0.000000000000000000, 0.000000000000000000 ) ) ;
#22448=CARTESIAN_POINT ( 'NONE',  ( 10.78723565514999905, -3581.600816721000228, 2246.630000000000109 ) ) ;
#22457=CARTESIAN_POINT ( 'NONE',  ( 28.24479999999899604, -3670.300000000000182, 2261.869999999999891 ) ) ;
#22462=DIRECTION ( 'NONE',  ( -1.000000000000000000, 0.000000000000000000, 0.000000000000000000 ) ) ;
#22463=EDGE_CURVE ( 'NONE', #4345, #6749, #18343, .T. ) ;
#22464=DIRECTION ( 'NONE',  ( -0.000000000000000000, -1.000000000000000000, -0.000000000000000000 ) ) ;
#22465=CARTESIAN_POINT ( 'NONE',  ( 88.90000000000000568, -3644.899999999999636, 2259.837999999999738 ) ) ;
#22471=VERTEX_POINT ( 'NONE', #10392 ) ;
#22473=CARTESIAN_POINT ( 'NONE',  ( 111.4552000000009997, -3594.099999999999909, 2259.837999999999738 ) ) ;
#22475=ORIENTED_EDGE ( 'NONE', *, *, #5999, .F. ) ;
#22477=CARTESIAN_POINT ( 'NONE',  ( 10.58079812952956544, -3657.607136393252858, 2248.687184364275254 ) ) ;
#22478=VERTEX_POINT ( 'NONE', #13678 ) ;
#22480=ORIENTED_EDGE ( 'NONE', *, *, #16938, .T. ) ;
#22481=VERTEX_POINT ( 'NONE', #14032 ) ;
#22483=ORIENTED_EDGE ( 'NONE', *, *, #1679, .T. ) ;
#22487=CARTESIAN_POINT ( 'NONE',  ( 141.9350057454958574, -3581.255064581549959, 2248.927129471270291 ) ) ;
#22488=ORIENTED_EDGE ( 'NONE', *, *, #9106, .T. ) ;
#22492=DIRECTION ( 'NONE',  ( -1.000000000000000000, 0.000000000000000000, 0.000000000000000000 ) ) ;
#22493=LINE ( 'NONE', #15363, #21225 ) ;
#22494=CIRCLE ( 'NONE', #11630, 0.7619999999999294005 ) ;
#22496=AXIS2_PLACEMENT_3D ( 'NONE', #11859, #17587, #22855 ) ;
#22497=ORIENTED_EDGE ( 'NONE', *, *, #2483, .F. ) ;
#22500=ORIENTED_EDGE ( 'NONE', *, *, #2351, .F. ) ;
#22506=DIRECTION ( 'NONE',  ( 0.000000000000000000, 0.000000000000000000, -1.000000000000000000 ) ) ;
#22508=VECTOR ( 'NONE', #13626, 1000.000000000000000 ) ;
#22510=CIRCLE ( 'NONE', #15420, 2.844800000000091700 ) ;
#22515=DIRECTION ( 'NONE',  ( 1.000000000000000000, 0.000000000000000000, 0.000000000000000000 ) ) ;
#22517=EDGE_CURVE ( 'NONE', #8026, #12415, #1826, .T. ) ;
#22523=ADVANCED_FACE ( 'NONE', ( #8407 ), #7094, .T. ) ;
#22525=ORIENTED_EDGE ( 'NONE', *, *, #10137, .F. ) ;
#22526=CIRCLE ( 'NONE', #18426, 2.844800000000091700 ) ;
#22527=CARTESIAN_POINT ( 'NONE',  ( 76.20000000000000284, -3670.300000000000182, 2239.771999999999935 ) ) ;
#22529=ORIENTED_EDGE ( 'NONE', *, *, #18147, .F. ) ;
#22533=EDGE_LOOP ( 'NONE', ( #5822, #48, #6569, #2104 ) ) ;
#22534=DIRECTION ( 'NONE',  ( -1.000000000000000000, 0.000000000000000000, 0.000000000000000000 ) ) ;
#22536=VECTOR ( 'NONE', #20326, 1000.000000000000000 ) ;
#22540=FACE_OUTER_BOUND ( 'NONE', #5436, .T. ) ;
#22544=AXIS2_PLACEMENT_3D ( 'NONE', #6314, #8289, #21922 ) ;
#22545=CARTESIAN_POINT ( 'NONE',  ( 20.66649961935109303, -3695.634659422622462, 2259.732127985863372 ) ) ;
#22546=EDGE_CURVE ( 'NONE', #5890, #2680, #17768, .T. ) ;
#22550=CIRCLE ( 'NONE', #16928, 5.715000000000997282 ) ;
#22553=CIRCLE ( 'NONE', #5366, 2.844800000000091700 ) ;
#22554=CARTESIAN_POINT ( 'NONE',  ( 10.90907282900277409, -3581.705358305645859, 2247.446708594144638 ) ) ;
#22555=DIRECTION ( 'NONE',  ( 0.000000000000000000, 0.000000000000000000, 1.000000000000000000 ) ) ;
#22557=CIRCLE ( 'NONE', #18813, 2.844800000000091700 ) ;
#22558=DIRECTION ( 'NONE',  ( 0.000000000000000000, 0.000000000000000000, -1.000000000000000000 ) ) ;
#22559=EDGE_CURVE ( 'NONE', #15832, #7984, #13865, .T. ) ;
#22560=CARTESIAN_POINT ( 'NONE',  ( 50.79999999999999716, -3670.300000000000182, 2259.837999999999738 ) ) ;
#22561=CARTESIAN_POINT ( 'NONE',  ( 144.6090632468122976, -3662.431858318084778, 2245.704773982281495 ) ) ;
#22563=DIRECTION ( 'NONE',  ( 0.000000000000000000, 0.000000000000000000, 1.000000000000000000 ) ) ;
#22564=CARTESIAN_POINT ( 'NONE',  ( 11.95719394751944620, -3662.251176165646939, 2249.298813514415542 ) ) ;
#22567=ORIENTED_EDGE ( 'NONE', *, *, #20232, .T. ) ;
#22568=CARTESIAN_POINT ( 'NONE',  ( 127.0000000000000000, -3619.500000000000000, 2259.837999999999738 ) ) ;
#22570=CARTESIAN_POINT ( 'NONE',  ( 88.90000000000000568, -3594.099999999999909, 2261.869999999999891 ) ) ;
#22574=ORIENTED_EDGE ( 'NONE', *, *, #7383, .F. ) ;
#22575=CARTESIAN_POINT ( 'NONE',  ( 116.8400000000000034, -3543.300000000000182, 2243.277199999999993 ) ) ;
#22576=EDGE_LOOP ( 'NONE', ( #16550, #19938, #3924, #11302 ) ) ;
#22581=EDGE_CURVE ( 'NONE', #4464, #18295, #20189, .T. ) ;
#22582=CARTESIAN_POINT ( 'NONE',  ( 147.8270794805000037, -3543.299999999999727, 2259.329999999999927 ) ) ;
#22583=DIRECTION ( 'NONE',  ( 0.000000000000000000, 0.000000000000000000, -1.000000000000000000 ) ) ;
#22585=CARTESIAN_POINT ( 'NONE',  ( 10.78733304872000076, -3657.399152860999493, 2246.630000000000109 ) ) ;
#22586=FACE_OUTER_BOUND ( 'NONE', #3203, .T. ) ;
#22588=VERTEX_POINT ( 'NONE', #10856 ) ;
#22589=AXIS2_PLACEMENT_3D ( 'NONE', #14175, #15802, #8892 ) ;
#22590=CARTESIAN_POINT ( 'NONE',  ( 101.5999999999999943, -3670.300000000000182, 2259.837999999999738 ) ) ;
#22591=LINE ( 'NONE', #801, #8807 ) ;
#22593=CARTESIAN_POINT ( 'NONE',  ( 10.55978476029679491, -3657.630734846978157, 2248.732827181204811 ) ) ;
#22594=ADVANCED_FACE ( 'NONE', ( #18004 ), #9108, .F. ) ;
#22595=ORIENTED_EDGE ( 'NONE', *, *, #10723, .F. ) ;
#22601=CARTESIAN_POINT ( 'NONE',  ( 105.2067999999999870, -3568.700000000000273, 2260.600000000000364 ) ) ;
#22603=DIRECTION ( 'NONE',  ( 0.6887494619146554697, 0.000000000000000000, -0.7249994335944496271 ) ) ;
#22604=ORIENTED_EDGE ( 'NONE', *, *, #16524, .T. ) ;
#22605=CARTESIAN_POINT ( 'NONE',  ( 131.8996122109008979, -3695.401597382865475, 2260.148187843663891 ) ) ;
#22608=AXIS2_PLACEMENT_3D ( 'NONE', #9880, #8143, #15286 ) ;
#22609=EDGE_CURVE ( 'NONE', #10895, #21188, #21299, .T. ) ;
#22610=TOROIDAL_SURFACE ( 'NONE', #11376, 3.606799999999999784, 0.7620000000000000107 ) ;
#22612=DIRECTION ( 'NONE',  ( 0.000000000000000000, 0.000000000000000000, 1.000000000000000000 ) ) ;
#22613=CARTESIAN_POINT ( 'NONE',  ( 127.0000000000000000, -3578.860000000000127, 2247.392000000000280 ) ) ;
#22619=DIRECTION ( 'NONE',  ( 0.000000000000000000, 0.000000000000000000, -1.000000000000000000 ) ) ;
#22620=TOROIDAL_SURFACE ( 'NONE', #8049, 4.114799999999999791, 1.270000000000000018 ) ;
#22621=VECTOR ( 'NONE', #17674, 1000.000000000000000 ) ;
#22622=FACE_OUTER_BOUND ( 'NONE', #21376, .T. ) ;
#22625=VERTEX_POINT ( 'NONE', #23145 ) ;
#22628=ORIENTED_EDGE ( 'NONE', *, *, #20614, .T. ) ;
#22630=CARTESIAN_POINT ( 'NONE',  ( 136.8552000000009912, -3659.504999999999654, 2272.030000000000200 ) ) ;
#22631=DIRECTION ( 'NONE',  ( -1.000000000000000000, 0.000000000000000000, 0.000000000000000000 ) ) ;
#22632=DIRECTION ( 'NONE',  ( -1.000000000000000000, 0.000000000000000000, 0.000000000000000000 ) ) ;
#22636=CARTESIAN_POINT ( 'NONE',  ( 18.41499991942999870, -3579.495498070999474, 2244.618783703000190 ) ) ;
#22637=CIRCLE ( 'NONE', #6197, 1.269999999999882334 ) ;
#22638=AXIS2_PLACEMENT_3D ( 'NONE', #18625, #10058, #916 ) ;
#22640=AXIS2_PLACEMENT_3D ( 'NONE', #21553, #2213, #3724 ) ;
#22641=CARTESIAN_POINT ( 'NONE',  ( 142.0593047748026265, -3657.915120415264937, 2249.165646973382536 ) ) ;
#22647=ORIENTED_EDGE ( 'NONE', *, *, #79, .F. ) ;
#22648=CARTESIAN_POINT ( 'NONE',  ( 4.572920519510999426, -3695.699999999999818, 2259.329999999999927 ) ) ;
#22656=DIRECTION ( 'NONE',  ( 1.000000000000000000, 0.000000000000000000, 0.000000000000000000 ) ) ;
#22658=AXIS2_PLACEMENT_3D ( 'NONE', #8545, #10168, #12165 ) ;
#22660=DIRECTION ( 'NONE',  ( 0.000000000000000000, 0.000000000000000000, -1.000000000000000000 ) ) ;
#22661=CIRCLE ( 'NONE', #6202, 5.714999999999998082 ) ;
#22662=CARTESIAN_POINT ( 'NONE',  ( 147.3199999999999932, -3694.430000000000291, 2260.600000000000364 ) ) ;
#22663=PLANE ( 'NONE',  #17712 ) ;
#22667=ORIENTED_EDGE ( 'NONE', *, *, #20668, .F. ) ;
#22668=CIRCLE ( 'NONE', #16328, 2.873832635400752622 ) ;
#22671=CARTESIAN_POINT ( 'NONE',  ( 10.25511876121471211, -3580.949311574155672, 2249.322936109902002 ) ) ;
#22674=ORIENTED_EDGE ( 'NONE', *, *, #21820, .T. ) ;
#22675=AXIS2_PLACEMENT_3D ( 'NONE', #22415, #14946, #22189 ) ;
#22678=ADVANCED_FACE ( 'NONE', ( #3703 ), #1837, .T. ) ;
#22680=CARTESIAN_POINT ( 'NONE',  ( 151.1299999999999955, -3694.430000000000291, 2259.329999999999927 ) ) ;
#22681=CARTESIAN_POINT ( 'NONE',  ( 144.5842015178808708, -3662.472695314643261, 2245.762539381157694 ) ) ;
#22682=LINE ( 'NONE', #8750, #9240 ) ;
#22683=CARTESIAN_POINT ( 'NONE',  ( 11.14436922434143895, -3661.887241596394233, 2249.637207235594815 ) ) ;
#22684=EDGE_CURVE ( 'NONE', #4703, #20008, #21411, .T. ) ;
#22685=CARTESIAN_POINT ( 'NONE',  ( 15.54478140927793284, -3659.506684851170121, 2250.165409776138404 ) ) ;
#22687=VERTEX_POINT ( 'NONE', #12731 ) ;
#22691=CARTESIAN_POINT ( 'NONE',  ( 14.47352478144048327, -3657.280624183466898, 2247.292342066113633 ) ) ;
#22693=ORIENTED_EDGE ( 'NONE', *, *, #8014, .T. ) ;
#22694=ORIENTED_EDGE ( 'NONE', *, *, #18857, .F. ) ;
#22695=CIRCLE ( 'NONE', #20107, 3.606799999999993567 ) ;
#22701=TOROIDAL_SURFACE ( 'NONE', #3618, 3.606799999999999784, 0.7620000000000000107 ) ;
#22703=DIRECTION ( 'NONE',  ( 0.000000000000000000, 0.000000000000000000, 1.000000000000000000 ) ) ;
#22705=CARTESIAN_POINT ( 'NONE',  ( 72.59320000000001016, -3670.300000000000182, 2239.771999999999935 ) ) ;
#22707=CARTESIAN_POINT ( 'NONE',  ( 137.1599999999999966, -3694.430000000000291, 2255.774000000000342 ) ) ;
#22708=CARTESIAN_POINT ( 'NONE',  ( 101.5999999999999943, -3568.700000000000273, 2261.869999999999891 ) ) ;
#22709=DIRECTION ( 'NONE',  ( 0.000000000000000000, -1.000000000000000000, 0.000000000000000000 ) ) ;
#22713=AXIS2_PLACEMENT_3D ( 'NONE', #9022, #14191, #5522 ) ;
#22715=ORIENTED_EDGE ( 'NONE', *, *, #11102, .F. ) ;
#22717=CARTESIAN_POINT ( 'NONE',  ( 10.61582386584563764, -3657.568526570700215, 2248.609309335925900 ) ) ;
#22720=ADVANCED_FACE ( 'NONE', ( #18683 ), #6728, .T. ) ;
#22721=AXIS2_PLACEMENT_3D ( 'NONE', #19228, #19107, #11843 ) ;
#22722=ORIENTED_EDGE ( 'NONE', *, *, #8578, .F. ) ;
#22723=DIRECTION ( 'NONE',  ( 0.000000000000000000, 0.000000000000000000, 1.000000000000000000 ) ) ;
#22724=EDGE_LOOP ( 'NONE', ( #22270, #3200, #9843, #21319 ) ) ;
#22733=EDGE_CURVE ( 'NONE', #11364, #982, #16433, .T. ) ;
#22734=AXIS2_PLACEMENT_3D ( 'NONE', #13063, #2286, #5693 ) ;
#22735=CARTESIAN_POINT ( 'NONE',  ( 134.1280881846921886, -3658.234155390725846, 2245.279838229026609 ) ) ;
#22736=DIRECTION ( 'NONE',  ( 1.000000000000000000, 0.000000000000000000, 0.000000000000000000 ) ) ;
#22738=CARTESIAN_POINT ( 'NONE',  ( 15.42897132338017130, -3695.419680871121727, 2255.300887234111087 ) ) ;
#22739=CARTESIAN_POINT ( 'NONE',  ( 29.00679999999900005, -3568.700000000000273, 2260.600000000000364 ) ) ;
#22742=AXIS2_PLACEMENT_3D ( 'NONE', #7763, #2486, #9847 ) ;
#22745=ORIENTED_EDGE ( 'NONE', *, *, #9968, .T. ) ;
#22746=EDGE_LOOP ( 'NONE', ( #9386, #7530, #3796, #13991 ) ) ;
#22748=CARTESIAN_POINT ( 'NONE',  ( 133.9879525578283221, -3659.716236870563534, 2244.576910402178783 ) ) ;
#22750=DIRECTION ( 'NONE',  ( -0.000000000000000000, -0.000000000000000000, -1.000000000000000000 ) ) ;
#22751=DIRECTION ( 'NONE',  ( 0.9296367896514280416, -0.3684771896964403326, 0.000000000000000000 ) ) ;
#22752=LINE ( 'NONE', #1308, #1989 ) ;
#22753=PLANE ( 'NONE',  #3613 ) ;
#22755=CARTESIAN_POINT ( 'NONE',  ( 6.985153502415998972, -3659.715133692337531, 2244.570904742638959 ) ) ;
#22757=CARTESIAN_POINT ( 'NONE',  ( 18.39651424583543005, -3579.956683882389825, 2244.766317903216077 ) ) ;
#22760=CARTESIAN_POINT ( 'NONE',  ( 141.6278228631028355, -3657.412925642543541, 2248.202207075162733 ) ) ;
#22762=AXIS2_PLACEMENT_3D ( 'NONE', #566, #11561, #22004 ) ;
#22763=CARTESIAN_POINT ( 'NONE',  ( 35.56000000000000227, -3695.699999999999818, 2247.392000000000280 ) ) ;
#22764=VERTEX_POINT ( 'NONE', #754 ) ;
#22765=ORIENTED_EDGE ( 'NONE', *, *, #4408, .F. ) ;
#22766=CARTESIAN_POINT ( 'NONE',  ( 139.6999999999999886, -3579.494999999999891, 2246.630000000000109 ) ) ;
#22770=CARTESIAN_POINT ( 'NONE',  ( 79.04479999999999507, -3670.300000000000182, 2259.837999999999738 ) ) ;
#22771=DIRECTION ( 'NONE',  ( -1.000000000000000000, 0.000000000000000000, 0.000000000000000000 ) ) ;
#22773=DIRECTION ( 'NONE',  ( -0.000000000000000000, -1.000000000000000000, -0.000000000000000000 ) ) ;
#22775=CARTESIAN_POINT ( 'NONE',  ( 131.7757523116999891, -3694.430000000000291, 2260.600000000000364 ) ) ;
#22780=VERTEX_POINT ( 'NONE', #13417 ) ;
#22781=FACE_OUTER_BOUND ( 'NONE', #13942, .T. ) ;
#22782=CARTESIAN_POINT ( 'NONE',  ( 10.48988688109928091, -3581.286862158647182, 2248.877936337259598 ) ) ;
#22783=DIRECTION ( 'NONE',  ( -1.000000000000000000, 0.000000000000000000, 0.000000000000000000 ) ) ;
#22785=ORIENTED_EDGE ( 'NONE', *, *, #19843, .T. ) ;
#22786=FACE_BOUND ( 'NONE', #16476, .T. ) ;
#22788=CARTESIAN_POINT ( 'NONE',  ( 144.3368584422871379, -3662.846051980176981, 2246.504844866363328 ) ) ;
#22790=CARTESIAN_POINT ( 'NONE',  ( 131.8084955422000064, -3694.472271328999796, 2260.600000000000364 ) ) ;
#22791=CARTESIAN_POINT ( 'NONE',  ( 12.37593526700610447, -3662.332104801266269, 2249.205209426644615 ) ) ;
#22792=CARTESIAN_POINT ( 'NONE',  ( 95.25000000000000000, -3694.430000000000291, 2244.547199999999975 ) ) ;
#22795=DIRECTION ( 'NONE',  ( 0.000000000000000000, -1.000000000000000000, 0.000000000000000000 ) ) ;
#22800=ORIENTED_EDGE ( 'NONE', *, *, #16015, .F. ) ;
#22801=EDGE_LOOP ( 'NONE', ( #19633, #7642, #4749, #19673, #3911, #3038, #10669, #19990 ) ) ;
#22806=ADVANCED_FACE ( 'NONE', ( #13300 ), #4285, .F. ) ;
#22808=AXIS2_PLACEMENT_3D ( 'NONE', #18798, #1100, #8261 ) ;
#22809=DIRECTION ( 'NONE',  ( 0.000000000000000000, 0.000000000000000000, -1.000000000000000000 ) ) ;
#22812=DIRECTION ( 'NONE',  ( 0.000000000000000000, -1.000000000000000000, 0.000000000000000000 ) ) ;
#22813=CARTESIAN_POINT ( 'NONE',  ( 130.6067999999989979, -3670.300000000000182, 2259.837999999999738 ) ) ;
#22815=FACE_OUTER_BOUND ( 'NONE', #13360, .T. ) ;
#22816=DIRECTION ( 'NONE',  ( 1.000000000000000000, 0.000000000000000000, 0.000000000000000000 ) ) ;
#22826=CARTESIAN_POINT ( 'NONE',  ( 10.07389198931091379, -3658.410956137315225, 2249.651275816309408 ) ) ;
#22829=CARTESIAN_POINT ( 'NONE',  ( 123.3932000000010021, -3568.700000000000273, 2239.009999999999764 ) ) ;
#22830=ORIENTED_EDGE ( 'NONE', *, *, #3677, .F. ) ;
#22836=ADVANCED_FACE ( 'NONE', ( #9337 ), #20120, .F. ) ;
#22838=ADVANCED_FACE ( 'NONE', ( #7569 ), #1455, .T. ) ;
#22841=CARTESIAN_POINT ( 'NONE',  ( 14.51399612240442671, -3581.686433941361429, 2247.717691707798622 ) ) ;
#22843=DIRECTION ( 'NONE',  ( 1.000000000000000000, 0.000000000000000000, 0.000000000000000000 ) ) ;
#22844=CARTESIAN_POINT ( 'NONE',  ( 86.05520000000001346, -3594.099999999999909, 2261.869999999999891 ) ) ;
#22845=EDGE_LOOP ( 'NONE', ( #18646, #9787, #19689, #4990 ) ) ;
#22846=CARTESIAN_POINT ( 'NONE',  ( 15.74707948048999917, -3695.699999999999818, 2254.503999999999905 ) ) ;
#22847=CIRCLE ( 'NONE', #421, 3.606800000000000228 ) ;
#22853=ORIENTED_EDGE ( 'NONE', *, *, #6732, .F. ) ;
#22855=DIRECTION ( 'NONE',  ( 1.000000000000000000, 0.000000000000000000, 0.000000000000000000 ) ) ;
#22857=EDGE_LOOP ( 'NONE', ( #16154, #19734, #338, #21255 ) ) ;
#22860=AXIS2_PLACEMENT_3D ( 'NONE', #5491, #3708, #7239 ) ;
#22861=DIRECTION ( 'NONE',  ( -0.000000000000000000, -1.000000000000000000, -0.000000000000000000 ) ) ;
#22863=AXIS2_PLACEMENT_3D ( 'NONE', #10824, #50, #394 ) ;
#22865=B_SPLINE_CURVE_WITH_KNOTS ( 'NONE', 3,
 ( #10385, #7112, #22685, #21295 ),
 .UNSPECIFIED., .F., .F.,
 ( 4, 4 ),
 ( 0.000000000000000000, 0.001021189648326963767 ),
 .UNSPECIFIED. ) ;
#22866=FACE_OUTER_BOUND ( 'NONE', #3197, .T. ) ;
#22867=DIRECTION ( 'NONE',  ( 0.000000000000000000, 0.000000000000000000, -1.000000000000000000 ) ) ;
#22868=CARTESIAN_POINT ( 'NONE',  ( 141.9677625471535123, -3657.787406547741739, 2248.991461943488048 ) ) ;
#22870=ADVANCED_FACE ( 'NONE', ( #22540 ), #6340, .T. ) ;
#22871=ORIENTED_EDGE ( 'NONE', *, *, #10723, .T. ) ;
#22879=CARTESIAN_POINT ( 'NONE',  ( 57.14999999999999858, -3670.300000000000182, 2250.236800000000130 ) ) ;
#22880=ORIENTED_EDGE ( 'NONE', *, *, #18452, .F. ) ;
#22884=DIRECTION ( 'NONE',  ( -1.000000000000000000, 0.000000000000000000, 0.000000000000000000 ) ) ;
#22886=VERTEX_POINT ( 'NONE', #1453 ) ;
#22887=FACE_OUTER_BOUND ( 'NONE', #1805, .T. ) ;
#22888=EDGE_CURVE ( 'NONE', #3220, #553, #18306, .T. ) ;
#22889=DIRECTION ( 'NONE',  ( 0.000000000000000000, 0.000000000000000000, -1.000000000000000000 ) ) ;
#22893=ORIENTED_EDGE ( 'NONE', *, *, #4275, .F. ) ;
#22897=AXIS2_PLACEMENT_3D ( 'NONE', #12908, #21473, #16533 ) ;
#22898=AXIS2_PLACEMENT_3D ( 'NONE', #9293, #14793, #379 ) ;
#22899=CARTESIAN_POINT ( 'NONE',  ( 10.77847718860299864, -3581.592869849620911, 2248.182432005671672 ) ) ;
#22902=ORIENTED_EDGE ( 'NONE', *, *, #2411, .T. ) ;
#22905=CARTESIAN_POINT ( 'NONE',  ( 144.5397947572051862, -3576.455561248520553, 2245.871466275620605 ) ) ;
#22908=CARTESIAN_POINT ( 'NONE',  ( 11.58645765754818413, -3662.123185233198910, 2249.431876995093717 ) ) ;
#22910=ORIENTED_EDGE ( 'NONE', *, *, #2274, .T. ) ;
#22913=DIRECTION ( 'NONE',  ( 0.000000000000000000, 0.000000000000000000, -1.000000000000000000 ) ) ;
#22916=CARTESIAN_POINT ( 'NONE',  ( 14.81248791361788264, -3657.599670035482177, 2248.672483178674611 ) ) ;
#22918=ORIENTED_EDGE ( 'NONE', *, *, #17863, .F. ) ;
#22919=LINE ( 'NONE', #21068, #15069 ) ;
#22920=VERTEX_POINT ( 'NONE', #2981 ) ;
#22921=CARTESIAN_POINT ( 'NONE',  ( 9.849632180192781306, -3543.399485434482813, 2254.996746371144127 ) ) ;
#22923=CIRCLE ( 'NONE', #11339, 3.606799999998994366 ) ;
#22924=DIRECTION ( 'NONE',  ( -1.000000000000000000, 0.000000000000000000, 0.000000000000000000 ) ) ;
#22927=AXIS2_PLACEMENT_3D ( 'NONE', #844, #7782, #9648 ) ;
#22929=CARTESIAN_POINT ( 'NONE',  ( 17.43609829863562766, -3576.295497495339077, 2246.158273476378326 ) ) ;
#22933=CARTESIAN_POINT ( 'NONE',  ( 97.99320000000000164, -3670.300000000000182, 2259.837999999999738 ) ) ;
#22934=EDGE_CURVE ( 'NONE', #16518, #7082, #11569, .T. ) ;
#22936=ORIENTED_EDGE ( 'NONE', *, *, #6216, .F. ) ;
#22937=CARTESIAN_POINT ( 'NONE',  ( 151.1299999999999955, -3544.570000000000164, 2260.600000000000364 ) ) ;
#22938=CARTESIAN_POINT ( 'NONE',  ( 10.29540294594043459, -3657.984965862048739, 2249.249084432865402 ) ) ;
#22939=AXIS2_PLACEMENT_3D ( 'NONE', #18218, #14171, #7029 ) ;
#22941=AXIS2_PLACEMENT_3D ( 'NONE', #11836, #13598, #20737 ) ;
#22942=VERTEX_POINT ( 'NONE', #8613 ) ;
#22944=ORIENTED_EDGE ( 'NONE', *, *, #19975, .T. ) ;
#22945=AXIS2_PLACEMENT_3D ( 'NONE', #21097, #3278, #1404 ) ;
#22949=CARTESIAN_POINT ( 'NONE',  ( 151.1299999999999955, -3660.140000000000327, 2244.547199999999975 ) ) ;
#22951=CARTESIAN_POINT ( 'NONE',  ( 145.4149999978999972, -3659.505243078000149, 2244.618209833000492 ) ) ;
#22952=ORIENTED_EDGE ( 'NONE', *, *, #4200, .T. ) ;
#22953=DIRECTION ( 'NONE',  ( 1.000000000000000000, 0.000000000000000000, 0.000000000000000000 ) ) ;
#22955=CARTESIAN_POINT ( 'NONE',  ( 66.34479999999999222, -3644.899999999999636, 2259.837999999999738 ) ) ;
#22956=CARTESIAN_POINT ( 'NONE',  ( 15.36332509443848160, -3580.494850336225227, 2249.720163181383214 ) ) ;
#22961=DIRECTION ( 'NONE',  ( 1.000000000000000000, 0.000000000000000000, 0.000000000000000000 ) ) ;
#22966=DIRECTION ( 'NONE',  ( 0.000000000000000000, 0.000000000000000000, -1.000000000000000000 ) ) ;
#22969=EDGE_CURVE ( 'NONE', #10469, #19192, #17955, .T. ) ;
#22970=DIRECTION ( 'NONE',  ( -1.000000000000000000, 0.000000000000000000, 0.000000000000000000 ) ) ;
#22971=ORIENTED_EDGE ( 'NONE', *, *, #19975, .F. ) ;
#22973=DIRECTION ( 'NONE',  ( -1.000000000000000000, 0.000000000000000000, 0.000000000000000000 ) ) ;
#22977=DIRECTION ( 'NONE',  ( 0.000000000000000000, 0.000000000000000000, -1.000000000000000000 ) ) ;
#22981=CARTESIAN_POINT ( 'NONE',  ( 15.74707948048999917, -3543.299999999999727, 2254.503999999999905 ) ) ;
#22984=CARTESIAN_POINT ( 'NONE',  ( 9.917068668310200508, -3695.517456592285271, 2255.165289491444582 ) ) ;
#22985=CARTESIAN_POINT ( 'NONE',  ( 18.30773776737111902, -3580.597427895495912, 2245.138331176275187 ) ) ;
#22986=EDGE_CURVE ( 'NONE', #5385, #14198, #17560, .T. ) ;
#22987=CARTESIAN_POINT ( 'NONE',  ( 137.3365850758355009, -3657.921631524508030, 2249.173164983783863 ) ) ;
#22988=VERTEX_POINT ( 'NONE', #4856 ) ;
#22994=VERTEX_POINT ( 'NONE', #2871 ) ;
#22997=LINE ( 'NONE', #3087, #7659 ) ;
#23000=CARTESIAN_POINT ( 'NONE',  ( 5.032662079066502869, -3543.933445094263789, 2260.481544455695257 ) ) ;
#23001=LINE ( 'NONE', #8608, #18138 ) ;
#23004=ORIENTED_EDGE ( 'NONE', *, *, #20045, .T. ) ;
#23005=EDGE_CURVE ( 'NONE', #5300, #20612, #13087, .T. ) ;
#23007=FACE_BOUND ( 'NONE', #3035, .T. ) ;
#23013=AXIS2_PLACEMENT_3D ( 'NONE', #16522, #14897, #474 ) ;
#23014=ORIENTED_EDGE ( 'NONE', *, *, #8012, .T. ) ;
#23015=AXIS2_PLACEMENT_3D ( 'NONE', #2272, #13266, #9420 ) ;
#23016=CARTESIAN_POINT ( 'NONE',  ( 9.855190710340998805, -3579.506215806999990, 2250.162457373000052 ) ) ;
#23017=EDGE_CURVE ( 'NONE', #10297, #2915, #19074, .T. ) ;
#23018=CARTESIAN_POINT ( 'NONE',  ( 10.30632217271526407, -3581.032148460298231, 2249.229053156336704 ) ) ;
#23020=EDGE_LOOP ( 'NONE', ( #3293, #5521, #6468, #16925 ) ) ;
#23023=EDGE_CURVE ( 'NONE', #982, #11364, #16822, .T. ) ;
#23025=CARTESIAN_POINT ( 'NONE',  ( 144.3716542413253876, -3576.201486203970035, 2246.367958886398810 ) ) ;
#23028=CARTESIAN_POINT ( 'NONE',  ( 11.90120768189071399, -3662.235409550263739, 2249.316113763095018 ) ) ;
#23030=CARTESIAN_POINT ( 'NONE',  ( 147.3200000001525041, -3544.490134410611063, 2260.599999999840747 ) ) ;
#23032=ORIENTED_EDGE ( 'NONE', *, *, #2841, .T. ) ;
#23033=CARTESIAN_POINT ( 'NONE',  ( 63.50000000000000000, -3594.099999999999909, 2260.600000000000364 ) ) ;
#23035=EDGE_CURVE ( 'NONE', #1541, #15774, #731, .T. ) ;
#23037=CARTESIAN_POINT ( 'NONE',  ( 14.95882340859066417, -3657.775661874956313, 2248.974051916531153 ) ) ;
#23038=CARTESIAN_POINT ( 'NONE',  ( 137.1569580771884489, -3694.590198011679149, 2255.766443268656985 ) ) ;
#23040=CARTESIAN_POINT ( 'NONE',  ( 127.0000000000000000, -3578.860000000000127, 2247.392000000000280 ) ) ;
#23043=AXIS2_PLACEMENT_3D ( 'NONE', #5099, #7089, #22884 ) ;
#23044=CARTESIAN_POINT ( 'NONE',  ( 10.16000000000000014, -3544.253380982895578, 2255.773999999999887 ) ) ;
#23046=DIRECTION ( 'NONE',  ( -1.000000000000000000, 0.000000000000000000, 0.000000000000000000 ) ) ;
#23047=AXIS2_PLACEMENT_3D ( 'NONE', #15761, #1337, #6744 ) ;
#23049=CARTESIAN_POINT ( 'NONE',  ( 116.8400000000000034, -3544.570000000000164, 2243.277199999999993 ) ) ;
#23052=DIRECTION ( 'NONE',  ( 1.000000000000000000, 0.000000000000000000, 0.000000000000000000 ) ) ;
#23053=CARTESIAN_POINT ( 'NONE',  ( 130.6067999999989979, -3619.500000000000000, 2239.009999999999764 ) ) ;
#23054=CIRCLE ( 'NONE', #12965, 0.7619999999999987894 ) ;
#23055=DIRECTION ( 'NONE',  ( 1.000000000000000000, 0.000000000000000000, 0.000000000000000000 ) ) ;
#23063=CIRCLE ( 'NONE', #22323, 2.844799999998995244 ) ;
#23065=EDGE_LOOP ( 'NONE', ( #11970, #11905, #3975, #3060 ) ) ;
#23067=CIRCLE ( 'NONE', #615, 2.844799999998998796 ) ;
#23069=ORIENTED_EDGE ( 'NONE', *, *, #63, .F. ) ;
#23073=CARTESIAN_POINT ( 'NONE',  ( 15.18361069157601229, -3580.883465275520393, 2249.392984458128922 ) ) ;
#23074=AXIS2_PLACEMENT_3D ( 'NONE', #9143, #16509, #17809 ) ;
#23075=CARTESIAN_POINT ( 'NONE',  ( 25.39999999999999858, -3568.700000000000273, 2259.837999999999738 ) ) ;
#23076=CARTESIAN_POINT ( 'NONE',  ( 142.4730284656999970, -3660.140000970000074, 2250.236800000000130 ) ) ;
#23078=DIRECTION ( 'NONE',  ( 0.000000000000000000, 0.000000000000000000, 1.000000000000000000 ) ) ;
#23079=EDGE_LOOP ( 'NONE', ( #663, #20974, #13126, #11939 ) ) ;
#23081=CIRCLE ( 'NONE', #5518, 6.477000000000010971 ) ;
#23085=DIRECTION ( 'NONE',  ( 0.000000000000000000, 0.000000000000000000, -1.000000000000000000 ) ) ;
#23086=VERTEX_POINT ( 'NONE', #14475 ) ;
#23088=DIRECTION ( 'NONE',  ( 0.000000000000000000, -1.000000000000000000, 0.000000000000000000 ) ) ;
#23093=DIRECTION ( 'NONE',  ( 0.7249994335945011414, 0.000000000000000000, -0.6887494619146010688 ) ) ;
#23094=( NAMED_UNIT ( * ) SI_UNIT ( $, .STERADIAN. ) SOLID_ANGLE_UNIT ( ) );
#23098=ORIENTED_EDGE ( 'NONE', *, *, #9137, .F. ) ;
#23099=ADVANCED_FACE ( 'NONE', ( #19857 ), #1866, .T. ) ;
#23102=FACE_OUTER_BOUND ( 'NONE', #11755, .T. ) ;
#23103=CARTESIAN_POINT ( 'NONE',  ( 116.8400000000000034, -3694.430000000000291, 2251.506800000000112 ) ) ;
#23105=ADVANCED_FACE ( 'NONE', ( #10831 ), #59, .F. ) ;
#23106=CARTESIAN_POINT ( 'NONE',  ( 137.0738540380190216, -3658.411045518359970, 2249.651344139286721 ) ) ;
#23107=ORIENTED_EDGE ( 'NONE', *, *, #10979, .F. ) ;
#23109=CARTESIAN_POINT ( 'NONE',  ( 137.1703043731272658, -3660.806955517932238, 2250.157730413952777 ) ) ;
#23111=ORIENTED_EDGE ( 'NONE', *, *, #4207, .T. ) ;
#23112=EDGE_CURVE ( 'NONE', #10464, #15794, #4850, .T. ) ;
#23114=EDGE_LOOP ( 'NONE', ( #18925, #1755, #3250 ) ) ;
#23116=ORIENTED_EDGE ( 'NONE', *, *, #5932, .T. ) ;
#23118=DIRECTION ( 'NONE',  ( 1.000000000000000000, 0.000000000000000000, 0.000000000000000000 ) ) ;
#23119=EDGE_CURVE ( 'NONE', #5432, #20367, #18093, .T. ) ;
#23124=FACE_BOUND ( 'NONE', #18983, .T. ) ;
#23125=CARTESIAN_POINT ( 'NONE',  ( 133.2229999999989900, -3579.494999999999891, 2239.009999999999764 ) ) ;
#23129=CARTESIAN_POINT ( 'NONE',  ( 131.5729205195000020, -3543.299999999999727, 2259.329999999999927 ) ) ;
#23131=DIRECTION ( 'NONE',  ( 0.000000000000000000, 0.000000000000000000, -1.000000000000000000 ) ) ;
#23132=FACE_OUTER_BOUND ( 'NONE', #12686, .T. ) ;
#23133=ORIENTED_EDGE ( 'NONE', *, *, #4371, .F. ) ;
#23134=CARTESIAN_POINT ( 'NONE',  ( 53.64479999999999649, -3619.500000000000000, 2259.837999999999738 ) ) ;
#23135=ADVANCED_FACE ( 'NONE', ( #8962, #23124, #14007, #16109, #5330, #7204, #7093, #21155, #3447, #10478, #1689, #14240, #17624, #1573, #23007, #6983, #12358, #10600, #12475, #10718, #7653, #20093, #11290, #4144, #5918, #5685, #18208 ), #18546, .T. ) ;
#23136=DIRECTION ( 'NONE',  ( -1.000000000000000000, 0.000000000000000000, 0.000000000000000000 ) ) ;
#23137=DIRECTION ( 'NONE',  ( 0.000000000000000000, 0.000000000000000000, -1.000000000000000000 ) ) ;
#23138=DIRECTION ( 'NONE',  ( 1.000000000000000000, 0.000000000000000000, 0.000000000000000000 ) ) ;
#23140=DIRECTION ( 'NONE',  ( -1.000000000000000000, 0.000000000000000000, 0.000000000000000000 ) ) ;
#23143=TOROIDAL_SURFACE ( 'NONE', #17529, 3.606799999998999695, 0.7620000000000000107 ) ;
#23144=CARTESIAN_POINT ( 'NONE',  ( 50.79999999999999716, -3568.700000000000273, 2260.600000000000364 ) ) ;
#23145=CARTESIAN_POINT ( 'NONE',  ( 7.020566483207999475, -3660.139755500999854, 2244.547200037999573 ) ) ;
#23146=CARTESIAN_POINT ( 'NONE',  ( 14.72058396313755146, -3657.501534252188321, 2248.460308617039573 ) ) ;
#23147=CARTESIAN_POINT ( 'NONE',  ( 136.6986431023520652, -3695.699999999999818, 2254.618513962067482 ) ) ;
#23148=ORIENTED_EDGE ( 'NONE', *, *, #6221, .F. ) ;
#23152=DIRECTION ( 'NONE',  ( 0.000000000000000000, 0.000000000000000000, -1.000000000000000000 ) ) ;
#23155=CARTESIAN_POINT ( 'NONE',  ( 114.2999999999999972, -3594.099999999999909, 2259.837999999999738 ) ) ;
#23156=CARTESIAN_POINT ( 'NONE',  ( 137.1599999999999966, -3694.430000000000291, 2255.774000000000342 ) ) ;
#23158=CARTESIAN_POINT ( 'NONE',  ( 127.0000000000000000, -3568.700000000000273, 2239.771999999999935 ) ) ;
#23160=EDGE_CURVE ( 'NONE', #21686, #3088, #3731, .T. ) ;
#23161=ADVANCED_FACE ( 'NONE', ( #14928 ), #14586, .T. ) ;
#23180=COLOUR_RGB('Dark Blue',0.08,0.2,0.34);
#23181=FILL_AREA_STYLE_COLOUR('',#23180);
#23182=FILL_AREA_STYLE('',(#23181));
#23183=SURFACE_STYLE_FILL_AREA(#23182);
#23184=SURFACE_SIDE_STYLE('',(#23183));
#23185=SURFACE_STYLE_USAGE(.BOTH.,#23184);
#23186=PRESENTATION_STYLE_ASSIGNMENT((#23185));
#23232=STYLED_ITEM('',(#23186),#21125);
#23237=MECHANICAL_DESIGN_GEOMETRIC_PRESENTATION_REPRESENTATION('',(#23232),#2257);
ENDSEC;
END-ISO-10303-21;
